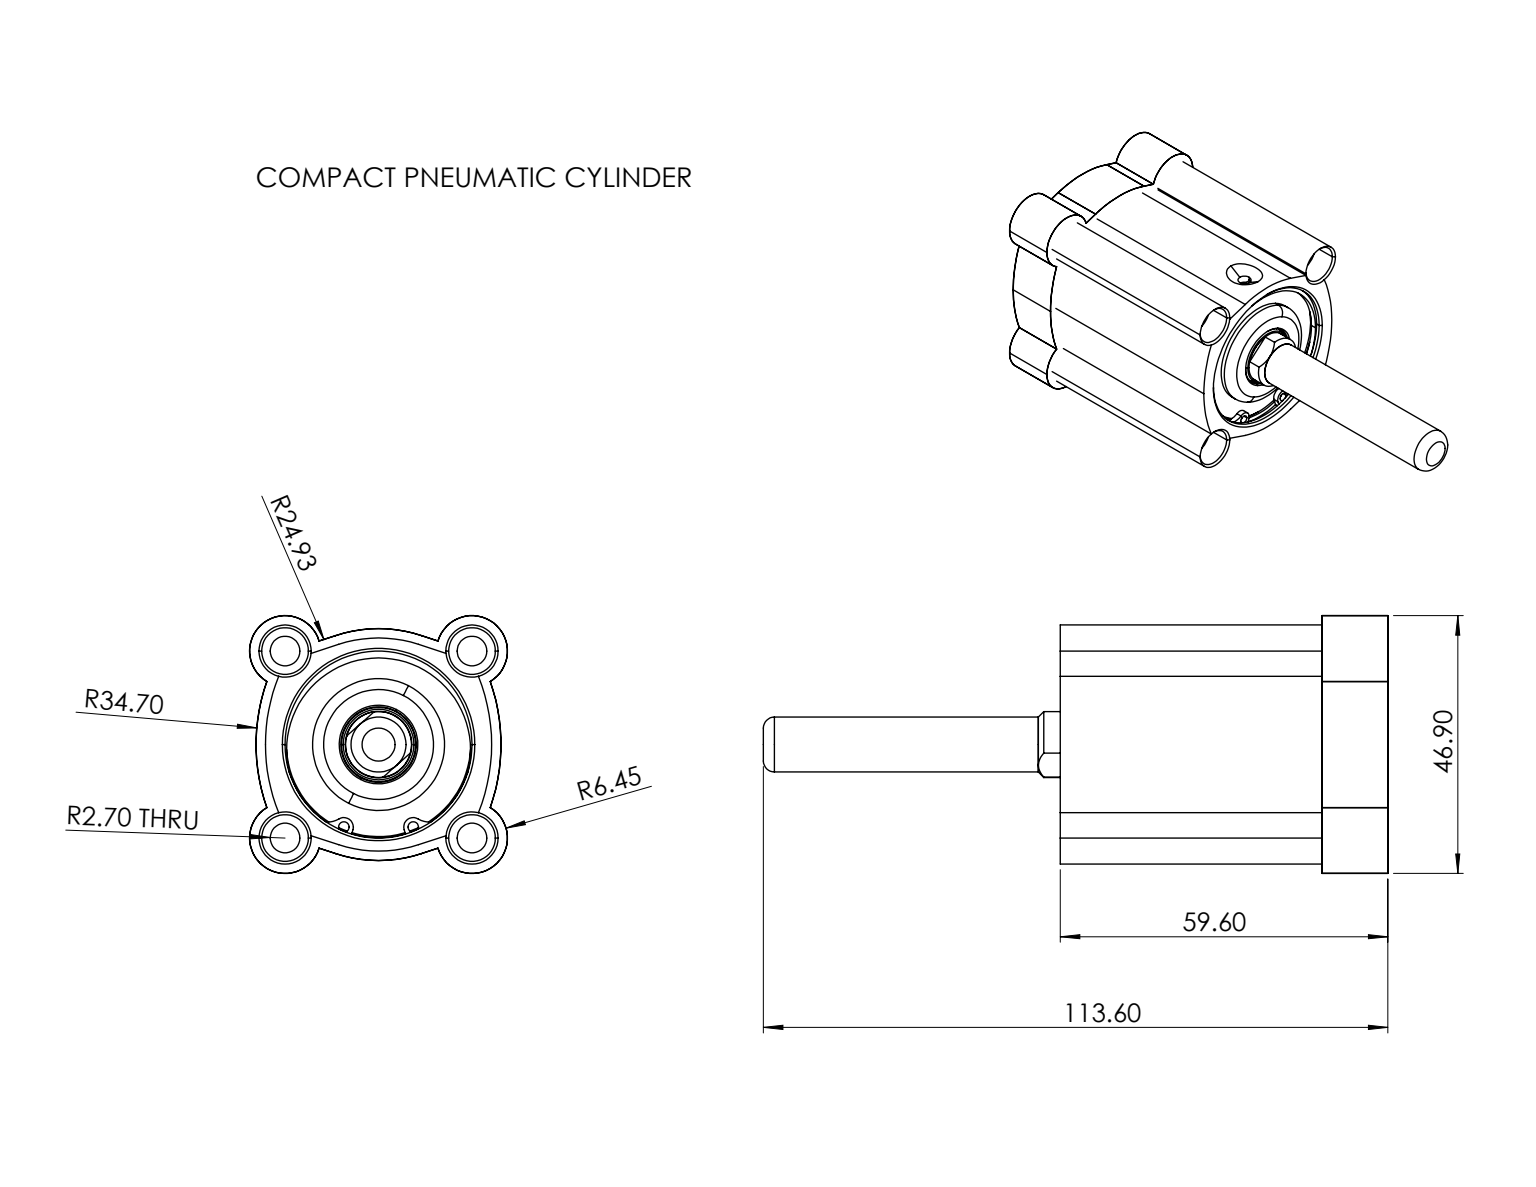
ISO-10303-21;
HEADER;
FILE_DESCRIPTION (('STEP AP214'),
    '1' );
FILE_NAME ('compact pneumatic cylinder.step',
    '2026-10-07T17:53:07',
    ( '' ),
    ( '' ),
    'SwSTEP 2.0',
    'SolidWorks 2025',
    '' );
FILE_SCHEMA (( 'AUTOMOTIVE_DESIGN' ));
ENDSEC;

DATA;
#3=CARTESIAN_POINT ( 'NONE',  ( -18.05918829504999934, 10.97290950744599947, 5.250000000000000000 ) ) ;
#4=FACE_OUTER_BOUND ( 'NONE', #8386, .T. ) ;
#6=VERTEX_POINT ( 'NONE', #3958 ) ;
#8=DIRECTION ( 'NONE',  ( -1.000000000000000000, 0.000000000000000000, 0.000000000000000000 ) ) ;
#10=AXIS2_PLACEMENT_3D ( 'NONE', #13272, #6842, #503 ) ;
#12=CARTESIAN_POINT ( 'NONE',  ( -40.33164489498319938, 10.97290950744599947, 5.250000000000000000 ) ) ;
#16=AXIS2_PLACEMENT_3D ( 'NONE', #5876, #10870, #7634 ) ;
#17=DIRECTION ( 'NONE',  ( -1.000000000000000000, 0.000000000000000000, 0.000000000000000000 ) ) ;
#19=CIRCLE ( 'NONE', #13399, 4.000000000000000888 ) ;
#22=ORIENTED_EDGE ( 'NONE', *, *, #9153, .T. ) ;
#23=EDGE_LOOP ( 'NONE', ( #6039, #6851, #1913, #2067 ) ) ;
#24=CARTESIAN_POINT ( 'NONE',  ( -26.35918829505000005, 10.97290950744599947, 61.86500000000000199 ) ) ;
#26=EDGE_LOOP ( 'NONE', ( #8749, #11948, #13282, #3929 ) ) ;
#27=DIRECTION ( 'NONE',  ( 0.000000000000000000, 0.000000000000000000, -1.000000000000000000 ) ) ;
#28=FACE_OUTER_BOUND ( 'NONE', #13183, .T. ) ;
#30=CARTESIAN_POINT ( 'NONE',  ( -18.05918829504999934, 10.97290950744599947, 57.35000000000000142 ) ) ;
#33=CIRCLE ( 'NONE', #3398, 4.749999999999997335 ) ;
#35=ADVANCED_FACE ( 'NONE', ( #1932 ), #13451, .T. ) ;
#40=CARTESIAN_POINT ( 'NONE',  ( -23.49332020752115113, 0.2738342970428629952, 62.85000000000000142 ) ) ;
#41=DIRECTION ( 'NONE',  ( 1.000000000000000000, 0.000000000000000000, 0.000000000000000000 ) ) ;
#42=CARTESIAN_POINT ( 'NONE',  ( -18.32356812262639068, 30.35913048975403683, 52.99871736656052690 ) ) ;
#44=CARTESIAN_POINT ( 'NONE',  ( -18.05918829505001355, 3.709013078446008027, 62.03182374100007479 ) ) ;
#46=CARTESIAN_POINT ( 'NONE',  ( -1.904759825251885141, 5.678153534393399759, 62.14999999999999858 ) ) ;
#48=( NAMED_UNIT ( * ) SI_UNIT ( $, .STERADIAN. ) SOLID_ANGLE_UNIT ( ) );
#49=CONICAL_SURFACE ( 'NONE', #4748, 17.00000000000000000, 0.7853981633974476129 ) ;
#50=EDGE_CURVE ( 'NONE', #1000, #13804, #2021, .T. ) ;
#53=ORIENTED_EDGE ( 'NONE', *, *, #11858, .F. ) ;
#55=CARTESIAN_POINT ( 'NONE',  ( -10.25088531517542023, -8.860076549334110041, 17.25000000000000000 ) ) ;
#56=CIRCLE ( 'NONE', #12775, 5.000000000000000888 ) ;
#57=CARTESIAN_POINT ( 'NONE',  ( -18.05918829504999934, 10.97290950744599947, 64.85000000000000853 ) ) ;
#58=SURFACE_SIDE_STYLE ('',( #2323 ) ) ;
#59=ORIENTED_EDGE ( 'NONE', *, *, #13776, .F. ) ;
#60=PLANE ( 'NONE',  #2670 ) ;
#62=DIRECTION ( 'NONE',  ( 1.000000000000000000, 0.000000000000000000, 0.000000000000000000 ) ) ;
#63=CARTESIAN_POINT ( 'NONE',  ( -5.631644894983189431, 10.97290950744599947, 17.25000000000000000 ) ) ;
#64=AXIS2_PLACEMENT_3D ( 'NONE', #1240, #10758, #11538 ) ;
#65=ORIENTED_EDGE ( 'NONE', *, *, #6040, .F. ) ;
#69=FACE_OUTER_BOUND ( 'NONE', #8366, .T. ) ;
#70=EDGE_CURVE ( 'NONE', #6919, #7844, #9610, .T. ) ;
#77=CARTESIAN_POINT ( 'NONE',  ( -24.37001676333060018, -4.028726038184999858, 62.14999999999999858 ) ) ;
#78=FACE_OUTER_BOUND ( 'NONE', #2382, .T. ) ;
#82=ORIENTED_EDGE ( 'NONE', *, *, #9714, .T. ) ;
#83=ORIENTED_EDGE ( 'NONE', *, *, #1868, .T. ) ;
#84=EDGE_LOOP ( 'NONE', ( #6155, #12083, #10918, #3272 ) ) ;
#87=VERTEX_POINT ( 'NONE', #8553 ) ;
#90=CARTESIAN_POINT ( 'NONE',  ( -19.42965429280413048, 26.91526772932534683, 56.72114474750378577 ) ) ;
#92=FACE_OUTER_BOUND ( 'NONE', #5027, .T. ) ;
#93=DIRECTION ( 'NONE',  ( 0.000000000000000000, 0.000000000000000000, -1.000000000000000000 ) ) ;
#94=ORIENTED_EDGE ( 'NONE', *, *, #9388, .F. ) ;
#95=VERTEX_POINT ( 'NONE', #8619 ) ;
#96=CARTESIAN_POINT ( 'NONE',  ( -15.05918829504999756, 10.97290950744599947, 118.8499999999999943 ) ) ;
#97=ORIENTED_EDGE ( 'NONE', *, *, #11700, .F. ) ;
#101=AXIS2_PLACEMENT_3D ( 'NONE', #2685, #3784, #6912 ) ;
#103=CARTESIAN_POINT ( 'NONE',  ( -29.51816008892539855, -2.179141222803619993, 63.45000000000000284 ) ) ;
#104=ORIENTED_EDGE ( 'NONE', *, *, #12811, .F. ) ;
#105=CARTESIAN_POINT ( 'NONE',  ( -3.531395436049983960, 3.709013078445997369, 62.03182374100001084 ) ) ;
#107=CARTESIAN_POINT ( 'NONE',  ( -20.77625425128555392, 5.623371902244430842, 57.35000000000000142 ) ) ;
#110=CLOSED_SHELL ( 'NONE', ( #5060, #3881, #6623, #9987, #3732, #7105, #7461, #11688, #1191, #4265, #947, #3436, #2543, #10818, #12397, #3818, #11545, #6558, #4609, #2381, #2843, #3214, #13267, #5308, #5232, #10919, #9049, #5614, #7802, #750 ) ) ;
#113=AXIS2_PLACEMENT_3D ( 'NONE', #7430, #11720, #2167 ) ;
#114=DIRECTION ( 'NONE',  ( 0.000000000000000000, 0.000000000000000000, 1.000000000000000000 ) ) ;
#116=ORIENTED_EDGE ( 'NONE', *, *, #8831, .F. ) ;
#117=ORIENTED_EDGE ( 'NONE', *, *, #6877, .T. ) ;
#118=PLANE ( 'NONE',  #6613 ) ;
#121=CYLINDRICAL_SURFACE ( 'NONE', #12455, 6.000000000000000888 ) ;
#122=LINE ( 'NONE', #4468, #12298 ) ;
#123=AXIS2_PLACEMENT_3D ( 'NONE', #1081, #954, #12877 ) ;
#124=DIRECTION ( 'NONE',  ( 0.000000000000000000, 0.000000000000000000, 1.000000000000000000 ) ) ;
#125=CARTESIAN_POINT ( 'NONE',  ( -18.05918829504999934, 10.97290950744599947, 68.84999999999999432 ) ) ;
#129=VERTEX_POINT ( 'NONE', #4238 ) ;
#130=EDGE_CURVE ( 'NONE', #6071, #11290, #13719, .T. ) ;
#131=CARTESIAN_POINT ( 'NONE',  ( -15.41688231577083101, 30.20956267305470178, 54.20385837980890642 ) ) ;
#134=FACE_OUTER_BOUND ( 'NONE', #5191, .T. ) ;
#136=PLANE ( 'NONE',  #5988 ) ;
#138=DIRECTION ( 'NONE',  ( 0.000000000000000000, 0.000000000000000000, 1.000000000000000000 ) ) ;
#139=ADVANCED_FACE ( 'NONE', ( #10588 ), #13367, .T. ) ;
#142=ORIENTED_EDGE ( 'NONE', *, *, #754, .F. ) ;
#143=EDGE_CURVE ( 'NONE', #7877, #9433, #12710, .T. ) ;
#144=DIRECTION ( 'NONE',  ( 0.000000000000000000, 0.000000000000000000, -1.000000000000000000 ) ) ;
#145=ORIENTED_EDGE ( 'NONE', *, *, #6603, .F. ) ;
#148=CARTESIAN_POINT ( 'NONE',  ( -25.33503448090910126, -7.245613863947209410, 64.85000000000000853 ) ) ;
#149=LINE ( 'NONE', #12938, #855 ) ;
#150=ORIENTED_EDGE ( 'NONE', *, *, #10812, .F. ) ;
#151=CARTESIAN_POINT ( 'NONE',  ( -1.059188295049996231, -6.027090492554000534, 7.250000000000000000 ) ) ;
#153=LINE ( 'NONE', #1273, #6867 ) ;
#154=CARTESIAN_POINT ( 'NONE',  ( -30.48673169511680214, 10.97290950744599947, 5.250000000000000000 ) ) ;
#160=VECTOR ( 'NONE', #1857, 1000.000000000000000 ) ;
#163=EDGE_LOOP ( 'NONE', ( #919, #320, #6279, #11884 ) ) ;
#164=EDGE_LOOP ( 'NONE', ( #8775, #9502, #10616, #5660 ) ) ;
#165=FACE_OUTER_BOUND ( 'NONE', #7206, .T. ) ;
#168=CIRCLE ( 'NONE', #7293, 6.299999999999998046 ) ;
#171=CARTESIAN_POINT ( 'NONE',  ( -20.25693731790400776, 30.25607652235614964, 53.78764270006948323 ) ) ;
#173=CARTESIAN_POINT ( 'NONE',  ( -8.964285665223000521, 0.3335619008453594714, 62.14999999999999858 ) ) ;
#175=CARTESIAN_POINT ( 'NONE',  ( -18.05918829504999934, 10.97290950744599947, 67.84999999999999432 ) ) ;
#176=CARTESIAN_POINT ( 'NONE',  ( -18.05918829504999934, 10.97290950744599947, 56.84999999999999432 ) ) ;
#178=AXIS2_PLACEMENT_3D ( 'NONE', #8254, #12725, #10295 ) ;
#180=AXIS2_PLACEMENT_3D ( 'NONE', #7057, #3723, #3934 ) ;
#185=ORIENTED_EDGE ( 'NONE', *, *, #5640, .F. ) ;
#192=VECTOR ( 'NONE', #12361, 1000.000000000000000 ) ;
#193=FILL_AREA_STYLE_COLOUR ( '', #3402 ) ;
#194=VERTEX_POINT ( 'NONE', #10221 ) ;
#195=VECTOR ( 'NONE', #13133, 1000.000000000000114 ) ;
#196=CARTESIAN_POINT ( 'NONE',  ( -35.05918829505000645, -6.027090492554000534, 7.250000000000000000 ) ) ;
#197=DIRECTION ( 'NONE',  ( 0.000000000000000000, 0.000000000000000000, -1.000000000000000000 ) ) ;
#199=CARTESIAN_POINT ( 'NONE',  ( -1.059188295049996231, 27.97290950744599769, 7.250000000000000000 ) ) ;
#203=CIRCLE ( 'NONE', #9813, 17.00000000000000355 ) ;
#204=CARTESIAN_POINT ( 'NONE',  ( -16.07719306376069568, 30.27579076690150117, 53.62366803667482174 ) ) ;
#206=EDGE_CURVE ( 'NONE', #7753, #7831, #10944, .T. ) ;
#210=PRESENTATION_STYLE_ASSIGNMENT (( #5374 ) ) ;
#213=CARTESIAN_POINT ( 'NONE',  ( -24.10918829505000005, 10.97290950744599947, 64.85000000000000853 ) ) ;
#214=AXIS2_PLACEMENT_3D ( 'NONE', #10840, #5509, #2126 ) ;
#215=AXIS2_PLACEMENT_3D ( 'NONE', #11989, #2447, #13100 ) ;
#216=ORIENTED_EDGE ( 'NONE', *, *, #2968, .F. ) ;
#218=ORIENTED_EDGE ( 'NONE', *, *, #1514, .T. ) ;
#219=DIRECTION ( 'NONE',  ( 0.000000000000000000, 0.000000000000000000, 1.000000000000000000 ) ) ;
#221=EDGE_CURVE ( 'NONE', #8225, #10962, #1891, .T. ) ;
#223=VERTEX_POINT ( 'NONE', #1688 ) ;
#224=VECTOR ( 'NONE', #4940, 1000.000000000000114 ) ;
#226=CIRCLE ( 'NONE', #12506, 15.45000000000000462 ) ;
#227=CONICAL_SURFACE ( 'NONE', #2931, 8.300000000000000711, 0.08573846772804097349 ) ;
#228=AXIS2_PLACEMENT_3D ( 'NONE', #13430, #6224, #8258 ) ;
#229=MANIFOLD_SOLID_BREP ( 'Boss-Extrude1', #6124 ) ;
#232=DIRECTION ( 'NONE',  ( 0.000000000000000000, 0.000000000000000000, 1.000000000000000000 ) ) ;
#233=EDGE_LOOP ( 'NONE', ( #8305, #2316, #6219, #5928, #5645 ) ) ;
#234=EDGE_CURVE ( 'NONE', #8205, #12910, #5618, .T. ) ;
#235=FACE_OUTER_BOUND ( 'NONE', #11663, .T. ) ;
#236=DIRECTION ( 'NONE',  ( -1.000000000000000000, 0.000000000000000000, 0.000000000000000000 ) ) ;
#237=CARTESIAN_POINT ( 'NONE',  ( -18.05918829504999223, 19.28555359244598932, 63.26601075299999621 ) ) ;
#238=CARTESIAN_POINT ( 'NONE',  ( -1.059188295049996231, 27.97290950744599769, 68.85549045786049760 ) ) ;
#239=ADVANCED_FACE ( 'NONE', ( #2830 ), #5929, .T. ) ;
#241=CIRCLE ( 'NONE', #3164, 3.450000000000001510 ) ;
#244=CIRCLE ( 'NONE', #12065, 6.449999999999997513 ) ;
#248=DIRECTION ( 'NONE',  ( 1.000000000000000000, 0.000000000000000000, 0.000000000000000000 ) ) ;
#250=DIRECTION ( 'NONE',  ( 0.000000000000000000, 0.000000000000000000, -1.000000000000000000 ) ) ;
#252=PLANE ( 'NONE',  #16 ) ;
#254=CARTESIAN_POINT ( 'NONE',  ( -19.60333775920156185, 30.30889438432964056, 53.36507960493299407 ) ) ;
#256=CIRCLE ( 'NONE', #8054, 7.618085573000000110 ) ;
#260=VECTOR ( 'NONE', #6397, 1000.000000000000000 ) ;
#261=DIRECTION ( 'NONE',  ( 1.000000000000000000, 0.000000000000000000, 0.000000000000000000 ) ) ;
#265=CIRCLE ( 'NONE', #7605, 16.66282263685194920 ) ;
#270=LINE ( 'NONE', #7860, #10180 ) ;
#271=ORIENTED_EDGE ( 'NONE', *, *, #8365, .T. ) ;
#272=CARTESIAN_POINT ( 'NONE',  ( -32.35918829505000360, -6.027090492554000534, 58.85000000000000142 ) ) ;
#273=CARTESIAN_POINT ( 'NONE',  ( -12.26420230435512160, 9.417873376788568507, 67.84999999999999432 ) ) ;
#277=CARTESIAN_POINT ( 'NONE',  ( -25.33503448090910126, -7.245613863947209410, 7.250000000000000000 ) ) ;
#278=FACE_OUTER_BOUND ( 'NONE', #4596, .T. ) ;
#281=DIRECTION ( 'NONE',  ( -1.000000000000000000, 0.000000000000000000, 0.000000000000000000 ) ) ;
#282=ADVANCED_FACE ( 'NONE', ( #9827 ), #5462, .T. ) ;
#288=CARTESIAN_POINT ( 'NONE',  ( -18.05918829504999934, 30.36027202460864771, 52.99086025162979752 ) ) ;
#290=CARTESIAN_POINT ( 'NONE',  ( -18.05918829249645086, 2.672909507443099741, 63.15000000009349179 ) ) ;
#291=CARTESIAN_POINT ( 'NONE',  ( -20.77625425128555392, 5.623371902244430842, 57.35000000000000142 ) ) ;
#293=CARTESIAN_POINT ( 'NONE',  ( 3.690811704950004657, 27.97290950744599769, 68.85549045786049760 ) ) ;
#297=ADVANCED_FACE ( 'NONE', ( #9087, #3790 ), #4208, .F. ) ;
#300=ORIENTED_EDGE ( 'NONE', *, *, #13287, .F. ) ;
#302=DIRECTION ( 'NONE',  ( 0.000000000000000000, 0.000000000000000000, 1.000000000000000000 ) ) ;
#306=ORIENTED_EDGE ( 'NONE', *, *, #4813, .T. ) ;
#308=DIRECTION ( 'NONE',  ( 0.4528443260392610026, 0.8915896008669278450, 0.000000000000000000 ) ) ;
#311=DIRECTION ( 'NONE',  ( 0.000000000000000000, 0.000000000000000000, 1.000000000000000000 ) ) ;
#312=DIRECTION ( 'NONE',  ( 0.1353548076753729457, 0.000000000000000000, -0.9907971921837297469 ) ) ;
#313=DIRECTION ( 'NONE',  ( -0.6615960714621569316, 0.7498604124941123938, 0.000000000000000000 ) ) ;
#316=ORIENTED_EDGE ( 'NONE', *, *, #12153, .T. ) ;
#318=VERTEX_POINT ( 'NONE', #915 ) ;
#319=CYLINDRICAL_SURFACE ( 'NONE', #4383, 15.45000000000000462 ) ;
#320=ORIENTED_EDGE ( 'NONE', *, *, #2823, .T. ) ;
#321=DIRECTION ( 'NONE',  ( -0.000000000000000000, -0.000000000000000000, 1.000000000000000000 ) ) ;
#322=VERTEX_POINT ( 'NONE', #8389 ) ;
#324=CARTESIAN_POINT ( 'NONE',  ( -21.18139722880372489, 30.14955231547764569, 54.83540917236412326 ) ) ;
#326=CARTESIAN_POINT ( 'NONE',  ( -18.05918829504999934, 2.872909508741170015, 63.35000000000700027 ) ) ;
#328=DIRECTION ( 'NONE',  ( 0.000000000000000000, 0.000000000000000000, 1.000000000000000000 ) ) ;
#330=ORIENTED_EDGE ( 'NONE', *, *, #13140, .T. ) ;
#331=EDGE_CURVE ( 'NONE', #12272, #3141, #6992, .T. ) ;
#334=DIRECTION ( 'NONE',  ( 1.000000000000000000, 0.000000000000000000, 0.000000000000000000 ) ) ;
#335=ORIENTED_EDGE ( 'NONE', *, *, #4099, .T. ) ;
#340=DIRECTION ( 'NONE',  ( -0.9496839325805417342, 0.3132098788326399541, 0.000000000000000000 ) ) ;
#341=LINE ( 'NONE', #9058, #8440 ) ;
#342=CARTESIAN_POINT ( 'NONE',  ( -34.05918829504999934, 10.97290950744599947, 56.84999999999999432 ) ) ;
#345=EDGE_CURVE ( 'NONE', #1822, #1130, #8251, .T. ) ;
#349=VERTEX_POINT ( 'NONE', #11530 ) ;
#350=EDGE_CURVE ( 'NONE', #12769, #6072, #4260, .T. ) ;
#351=ORIENTED_EDGE ( 'NONE', *, *, #13017, .F. ) ;
#358=DIRECTION ( 'NONE',  ( 0.000000000000000000, 0.000000000000000000, -1.000000000000000000 ) ) ;
#360=FACE_OUTER_BOUND ( 'NONE', #13071, .T. ) ;
#364=DIRECTION ( 'NONE',  ( 1.000000000000000000, 0.000000000000000000, 0.000000000000000000 ) ) ;
#368=CARTESIAN_POINT ( 'NONE',  ( -32.58698115404997253, 18.23680593644601089, 62.03182374100001084 ) ) ;
#370=CARTESIAN_POINT ( 'NONE',  ( -11.06274345774342116, 24.74796884084004844, 60.65000000000000568 ) ) ;
#372=CIRCLE ( 'NONE', #1703, 1.725000000000000755 ) ;
#373=CARTESIAN_POINT ( 'NONE',  ( -17.25681213616876164, 26.95277304015176512, 56.08231620102305470 ) ) ;
#382=LINE ( 'NONE', #4652, #10884 ) ;
#383=CARTESIAN_POINT ( 'NONE',  ( -21.60736175305857998, 30.08769857173765416, 55.71792893088887411 ) ) ;
#385=DIRECTION ( 'NONE',  ( -1.000000000000000000, 0.000000000000000000, 0.000000000000000000 ) ) ;
#386=DIRECTION ( 'NONE',  ( -0.9496839325805417342, -0.3132098788326399541, 0.000000000000000000 ) ) ;
#388=AXIS2_PLACEMENT_3D ( 'NONE', #10817, #5485, #2106 ) ;
#393=CIRCLE ( 'NONE', #6637, 4.749999999999997335 ) ;
#394=AXIS2_PLACEMENT_3D ( 'NONE', #13518, #1937, #13587 ) ;
#397=CYLINDRICAL_SURFACE ( 'NONE', #11158, 6.450000000000009948 ) ;
#398=ORIENTED_EDGE ( 'NONE', *, *, #7843, .T. ) ;
#406=ADVANCED_FACE ( 'NONE', ( #4 ), #7444, .T. ) ;
#407=LINE ( 'NONE', #1517, #3985 ) ;
#409=PLANE ( 'NONE',  #6769 ) ;
#410=LINE ( 'NONE', #10063, #2675 ) ;
#411=AXIS2_PLACEMENT_3D ( 'NONE', #10209, #2683, #4898 ) ;
#415=ORIENTED_EDGE ( 'NONE', *, *, #1664, .T. ) ;
#416=LINE ( 'NONE', #7878, #12614 ) ;
#418=VECTOR ( 'NONE', #5319, 1000.000000000000000 ) ;
#419=AXIS2_PLACEMENT_3D ( 'NONE', #7166, #4046, #8361 ) ;
#420=ORIENTED_EDGE ( 'NONE', *, *, #7245, .F. ) ;
#421=ADVANCED_FACE ( 'NONE', ( #4551 ), #12019, .T. ) ;
#422=DIRECTION ( 'NONE',  ( 0.000000000000000000, 0.000000000000000000, -1.000000000000000000 ) ) ;
#423=AXIS2_PLACEMENT_3D ( 'NONE', #11901, #6648, #2493 ) ;
#425=ORIENTED_EDGE ( 'NONE', *, *, #4953, .T. ) ;
#428=EDGE_CURVE ( 'NONE', #7051, #87, #10065, .T. ) ;
#429=CARTESIAN_POINT ( 'NONE',  ( -24.10918829505000005, 10.97290950744599947, 64.85000000000000853 ) ) ;
#430=CIRCLE ( 'NONE', #8236, 6.145833333000000565 ) ;
#432=EDGE_LOOP ( 'NONE', ( #10471, #3421, #1762, #3978 ) ) ;
#439=ORIENTED_EDGE ( 'NONE', *, *, #6372, .F. ) ;
#441=ORIENTED_EDGE ( 'NONE', *, *, #8899, .T. ) ;
#443=CONICAL_SURFACE ( 'NONE', #7785, 16.95000000000000284, 0.7853981633974433940 ) ;
#444=FACE_OUTER_BOUND ( 'NONE', #7372, .T. ) ;
#446=DIRECTION ( 'NONE',  ( -1.000000000000000000, 0.000000000000000000, 0.000000000000000000 ) ) ;
#450=VECTOR ( 'NONE', #8530, 1000.000000000000227 ) ;
#451=VECTOR ( 'NONE', #9676, 1000.000000000000000 ) ;
#456=CARTESIAN_POINT ( 'NONE',  ( -21.14708333414588637, 30.15419697583712733, 54.78115759698135889 ) ) ;
#457=CARTESIAN_POINT ( 'NONE',  ( -18.05918829504999934, 10.97290950744599947, 57.35000000000000142 ) ) ;
#458=CARTESIAN_POINT ( 'NONE',  ( -41.50918829505000218, -6.027090492554000534, 17.25000000000000000 ) ) ;
#460=DIRECTION ( 'NONE',  ( 0.000000000000000000, 0.000000000000000000, -1.000000000000000000 ) ) ;
#461=DIRECTION ( 'NONE',  ( -0.000000000000000000, -0.000000000000000000, 1.000000000000000000 ) ) ;
#462=VECTOR ( 'NONE', #11230, 1000.000000000000227 ) ;
#466=AXIS2_PLACEMENT_3D ( 'NONE', #5182, #8642, #10822 ) ;
#467=VERTEX_POINT ( 'NONE', #290 ) ;
#469=EDGE_CURVE ( 'NONE', #3141, #10024, #8658, .T. ) ;
#471=CARTESIAN_POINT ( 'NONE',  ( -12.54628844161313950, -7.366404416634599883, 63.45000000000000284 ) ) ;
#472=CONICAL_SURFACE ( 'NONE', #3607, 6.049999999999999822, 0.1357715569457985105 ) ;
#474=DIRECTION ( 'NONE',  ( 1.000000000000000000, 0.000000000000000000, 0.000000000000000000 ) ) ;
#475=AXIS2_PLACEMENT_3D ( 'NONE', #3143, #10327, #12625 ) ;
#476=EDGE_LOOP ( 'NONE', ( #7429, #4886, #7264, #4257 ) ) ;
#477=CYLINDRICAL_SURFACE ( 'NONE', #9605, 8.299999999999998934 ) ;
#480=CARTESIAN_POINT ( 'NONE',  ( 0.09777679598749920709, -1.420146627243660031, 68.85549045786049760 ) ) ;
#482=DIRECTION ( 'NONE',  ( -1.000000000000000000, 0.000000000000000000, 0.000000000000000000 ) ) ;
#483=DIRECTION ( 'NONE',  ( -0.000000000000000000, -0.000000000000000000, 1.000000000000000000 ) ) ;
#484=DIRECTION ( 'NONE',  ( -0.3132098788326420635, -0.9496839325805410681, 0.000000000000000000 ) ) ;
#485=DIRECTION ( 'NONE',  ( 0.000000000000000000, 0.000000000000000000, -1.000000000000000000 ) ) ;
#491=ORIENTED_EDGE ( 'NONE', *, *, #6716, .F. ) ;
#493=CARTESIAN_POINT ( 'NONE',  ( -23.85417428574490373, 12.52794563810342154, 67.84999999999999432 ) ) ;
#494=ORIENTED_EDGE ( 'NONE', *, *, #12786, .T. ) ;
#495=EDGE_LOOP ( 'NONE', ( #8465, #5386, #11204, #2294 ) ) ;
#497=EDGE_CURVE ( 'NONE', #7929, #3451, #2337, .T. ) ;
#500=LINE ( 'NONE', #3780, #1311 ) ;
#501=CARTESIAN_POINT ( 'NONE',  ( 1.640811704950005057, 27.97290950744599769, 7.250000000000000000 ) ) ;
#502=CARTESIAN_POINT ( 'NONE',  ( -11.75918829505000041, 10.97290950744599947, 61.86500000000000199 ) ) ;
#503=DIRECTION ( 'NONE',  ( -1.000000000000000000, 0.000000000000000000, 0.000000000000000000 ) ) ;
#504=EDGE_CURVE ( 'NONE', #3446, #7761, #4041, .T. ) ;
#506=VERTEX_POINT ( 'NONE', #8735 ) ;
#508=CARTESIAN_POINT ( 'NONE',  ( -16.54062941099373063, 30.31058478656570188, 61.34775567103718430 ) ) ;
#509=ORIENTED_EDGE ( 'NONE', *, *, #7168, .F. ) ;
#512=EDGE_LOOP ( 'NONE', ( #3363, #9806, #10726, #5357 ) ) ;
#515=CARTESIAN_POINT ( 'NONE',  ( -18.05918829504999934, 10.97290950744599947, 61.65955166399999854 ) ) ;
#516=DIRECTION ( 'NONE',  ( 0.000000000000000000, 0.000000000000000000, 1.000000000000000000 ) ) ;
#518=CYLINDRICAL_SURFACE ( 'NONE', #11011, 6.299999999999999822 ) ;
#520=CARTESIAN_POINT ( 'NONE',  ( -30.80918829504999934, -6.027090492554000534, 64.35000000000000853 ) ) ;
#521=ADVANCED_FACE ( 'NONE', ( #9868 ), #13062, .F. ) ;
#523=EDGE_CURVE ( 'NONE', #7555, #10214, #3846, .T. ) ;
#524=LINE ( 'NONE', #7913, #11304 ) ;
#526=CARTESIAN_POINT ( 'NONE',  ( -25.64433075620760150, -3.961216307075045240, 61.85000000000000142 ) ) ;
#527=CARTESIAN_POINT ( 'NONE',  ( -21.02695553212586432, 30.16999431196798298, 60.09573059200643286 ) ) ;
#529=DIRECTION ( 'NONE',  ( 0.000000000000000000, 0.000000000000000000, -1.000000000000000000 ) ) ;
#531=AXIS2_PLACEMENT_3D ( 'NONE', #7726, #6695, #2740 ) ;
#532=DIRECTION ( 'NONE',  ( 0.000000000000000000, 0.000000000000000000, -1.000000000000000000 ) ) ;
#533=VERTEX_POINT ( 'NONE', #10767 ) ;
#534=CARTESIAN_POINT ( 'NONE',  ( -18.05918829504999934, 10.00028003023991907, 62.14999999999999858 ) ) ;
#537=DIRECTION ( 'NONE',  ( 1.000000000000000000, 0.000000000000000000, 0.000000000000000000 ) ) ;
#538=( LENGTH_UNIT ( ) NAMED_UNIT ( * ) SI_UNIT ( .MILLI., .METRE. ) );
#542=DIRECTION ( 'NONE',  ( 0.000000000000000000, 0.000000000000000000, 1.000000000000000000 ) ) ;
#545=DIRECTION ( 'NONE',  ( 1.000000000000000000, 0.000000000000000000, 0.000000000000000000 ) ) ;
#546=MECHANICAL_DESIGN_GEOMETRIC_PRESENTATION_REPRESENTATION('',(#12596),#10109);
#547=DIRECTION ( 'NONE',  ( 0.000000000000000000, 0.000000000000000000, -1.000000000000000000 ) ) ;
#548=DIRECTION ( 'NONE',  ( 0.000000000000000000, 0.000000000000000000, -1.000000000000000000 ) ) ;
#549=ORIENTED_EDGE ( 'NONE', *, *, #8020, .F. ) ;
#550=ORIENTED_EDGE ( 'NONE', *, *, #345, .F. ) ;
#552=ORIENTED_EDGE ( 'NONE', *, *, #7488, .T. ) ;
#553=ORIENTED_EDGE ( 'NONE', *, *, #616, .F. ) ;
#554=FACE_OUTER_BOUND ( 'NONE', #6549, .T. ) ;
#557=EDGE_LOOP ( 'NONE', ( #13661, #2052 ) ) ;
#558=DIRECTION ( 'NONE',  ( 0.000000000000000000, 0.000000000000000000, -1.000000000000000000 ) ) ;
#560=VECTOR ( 'NONE', #10996, 1000.000000000000227 ) ;
#563=CARTESIAN_POINT ( 'NONE',  ( -18.05918829504999934, 10.97290950744599947, 62.14999999999999858 ) ) ;
#564=DIRECTION ( 'NONE',  ( 0.000000000000000000, 0.000000000000000000, -1.000000000000000000 ) ) ;
#567=ORIENTED_EDGE ( 'NONE', *, *, #3893, .T. ) ;
#568=VECTOR ( 'NONE', #12571, 1000.000000000000000 ) ;
#569=ORIENTED_EDGE ( 'NONE', *, *, #3319, .T. ) ;
#575=CARTESIAN_POINT ( 'NONE',  ( -32.58698115404997253, 3.709013078445997369, 62.03182374100001084 ) ) ;
#576=CARTESIAN_POINT ( 'NONE',  ( -36.21615338608749823, -1.420146627243662030, 64.85000000000000853 ) ) ;
#578=LINE ( 'NONE', #5112, #2725 ) ;
#579=CARTESIAN_POINT ( 'NONE',  ( -24.37001676333060018, -4.028726038184999858, 62.14999999999999858 ) ) ;
#581=DIRECTION ( 'NONE',  ( 0.000000000000000000, 0.000000000000000000, 1.000000000000000000 ) ) ;
#582=AXIS2_PLACEMENT_3D ( 'NONE', #4592, #10119, #13246 ) ;
#584=EDGE_CURVE ( 'NONE', #1164, #10151, #226, .T. ) ;
#585=ORIENTED_EDGE ( 'NONE', *, *, #2198, .T. ) ;
#586=VERTEX_POINT ( 'NONE', #11046 ) ;
#587=AXIS2_PLACEMENT_3D ( 'NONE', #4402, #8584, #10906 ) ;
#588=DIRECTION ( 'NONE',  ( 1.000000000000000000, 0.000000000000000000, 0.000000000000000000 ) ) ;
#589=ORIENTED_EDGE ( 'NONE', *, *, #8356, .F. ) ;
#590=CARTESIAN_POINT ( 'NONE',  ( -18.05918829504999934, 10.97290950744599947, 63.64999999999999858 ) ) ;
#592=CARTESIAN_POINT ( 'NONE',  ( -20.85553867603828593, 30.19135017469169924, 60.31826595084313425 ) ) ;
#593=DIRECTION ( 'NONE',  ( 0.000000000000000000, 0.000000000000000000, -1.000000000000000000 ) ) ;
#594=CARTESIAN_POINT ( 'NONE',  ( -30.80918829504999934, 27.97290950744599769, 64.35000000000000853 ) ) ;
#596=CARTESIAN_POINT ( 'NONE',  ( -25.67727386805000123, 10.97290950744599947, 61.65955166399999854 ) ) ;
#598=CIRCLE ( 'NONE', #5937, 17.00000000000000355 ) ;
#601=DIRECTION ( 'NONE',  ( 0.000000000000000000, 0.000000000000000000, 1.000000000000000000 ) ) ;
#603=CARTESIAN_POINT ( 'NONE',  ( -1.059188295049996231, 27.97290950744599769, 58.85000000000000142 ) ) ;
#605=CARTESIAN_POINT ( 'NONE',  ( -10.38347696868452097, 26.08535324214045303, 57.35000000000000142 ) ) ;
#606=CARTESIAN_POINT ( 'NONE',  ( -18.05918829504999934, 10.97290950744599947, 118.8499999999999943 ) ) ;
#609=DIRECTION ( 'NONE',  ( 0.000000000000000000, 0.000000000000000000, -1.000000000000000000 ) ) ;
#611=CARTESIAN_POINT ( 'NONE',  ( -18.05918829504999934, 10.97290950744599947, 23.90000000000000213 ) ) ;
#613=AXIS2_PLACEMENT_3D ( 'NONE', #13711, #12870, #3257 ) ;
#614=CIRCLE ( 'NONE', #1290, 1.999999999999998890 ) ;
#616=EDGE_CURVE ( 'NONE', #1958, #10012, #1673, .T. ) ;
#617=DIRECTION ( 'NONE',  ( 1.000000000000000000, 0.000000000000000000, 0.000000000000000000 ) ) ;
#625=AXIS2_PLACEMENT_3D ( 'NONE', #11625, #6317, #6376 ) ;
#626=CARTESIAN_POINT ( 'NONE',  ( -34.49120980104999035, 2.756898754446010180, 63.36264408499989287 ) ) ;
#628=CYLINDRICAL_SURFACE ( 'NONE', #4795, 6.449999999999997513 ) ;
#632=ADVANCED_FACE ( 'NONE', ( #10206 ), #9225, .F. ) ;
#633=CIRCLE ( 'NONE', #10686, 12.00000000000000355 ) ;
#635=CARTESIAN_POINT ( 'NONE',  ( -15.98447378135880292, 30.26743272304607402, 61.00728932202151356 ) ) ;
#637=ORIENTED_EDGE ( 'NONE', *, *, #12632, .F. ) ;
#639=CARTESIAN_POINT ( 'NONE',  ( -46.97970805730049904, -0.1071066662815775977, 64.85000000000000853 ) ) ;
#640=CARTESIAN_POINT ( 'NONE',  ( -32.37473156004999453, 18.13068114044599710, 61.70038048200006386 ) ) ;
#641=LINE ( 'NONE', #12326, #4442 ) ;
#642=VERTEX_POINT ( 'NONE', #12160 ) ;
#643=CARTESIAN_POINT ( 'NONE',  ( 0.09777679598749920709, -1.420146627243660031, 64.85000000000000853 ) ) ;
#644=DIRECTION ( 'NONE',  ( 1.000000000000000000, 0.000000000000000000, 0.000000000000000000 ) ) ;
#647=CARTESIAN_POINT ( 'NONE',  ( -16.74984313037099781, 27.92258346524268475, 58.10825715175638351 ) ) ;
#648=CIRCLE ( 'NONE', #4894, 6.595833333000001630 ) ;
#649=DIRECTION ( 'NONE',  ( 0.000000000000000000, 0.000000000000000000, -1.000000000000000000 ) ) ;
#651=VERTEX_POINT ( 'NONE', #8027 ) ;
#652=ORIENTED_EDGE ( 'NONE', *, *, #9198, .T. ) ;
#653=CIRCLE ( 'NONE', #8245, 18.00000000000000000 ) ;
#658=DIRECTION ( 'NONE',  ( -1.000000000000000000, 0.000000000000000000, 0.000000000000000000 ) ) ;
#659=DIRECTION ( 'NONE',  ( 0.000000000000000000, 0.000000000000000000, -1.000000000000000000 ) ) ;
#665=VERTEX_POINT ( 'NONE', #12304 ) ;
#666=ORIENTED_EDGE ( 'NONE', *, *, #3497, .T. ) ;
#668=CARTESIAN_POINT ( 'NONE',  ( -32.35918829505000360, 27.97290950744599769, 58.85000000000000142 ) ) ;
#670=DIRECTION ( 'NONE',  ( 0.000000000000000000, 0.000000000000000000, -1.000000000000000000 ) ) ;
#671=DIRECTION ( 'NONE',  ( -1.000000000000000000, 0.000000000000000000, 0.000000000000000000 ) ) ;
#672=AXIS2_PLACEMENT_3D ( 'NONE', #7930, #1510, #1232 ) ;
#673=AXIS2_PLACEMENT_3D ( 'NONE', #3504, #2473, #9929 ) ;
#676=DIRECTION ( 'NONE',  ( 1.000000000000000000, 0.000000000000000000, 0.000000000000000000 ) ) ;
#677=AXIS2_PLACEMENT_3D ( 'NONE', #13631, #848, #1908 ) ;
#679=DIRECTION ( 'NONE',  ( 0.000000000000000000, -1.000000000000000000, 0.000000000000000000 ) ) ;
#684=VECTOR ( 'NONE', #328, 1000.000000000000000 ) ;
#686=DIRECTION ( 'NONE',  ( 0.000000000000000000, 1.000000000000000000, 0.000000000000000000 ) ) ;
#688=EDGE_CURVE ( 'NONE', #1735, #8958, #13408, .T. ) ;
#690=CYLINDRICAL_SURFACE ( 'NONE', #8513, 6.449999999999997513 ) ;
#692=AXIS2_PLACEMENT_3D ( 'NONE', #1538, #7951, #7885 ) ;
#693=AXIS2_PLACEMENT_3D ( 'NONE', #7006, #13442, #12398 ) ;
#695=AXIS2_PLACEMENT_3D ( 'NONE', #7919, #9259, #8346 ) ;
#697=DIRECTION ( 'NONE',  ( 0.000000000000000000, 0.000000000000000000, 1.000000000000000000 ) ) ;
#698=AXIS2_PLACEMENT_3D ( 'NONE', #6763, #12980, #13188 ) ;
#700=CARTESIAN_POINT ( 'NONE',  ( -15.26994104352865023, 30.19221003217483101, 60.32689770076000713 ) ) ;
#701=ADVANCED_FACE ( 'NONE', ( #12089 ), #8706, .T. ) ;
#702=ORIENTED_EDGE ( 'NONE', *, *, #5578, .T. ) ;
#703=VERTEX_POINT ( 'NONE', #12706 ) ;
#705=LINE ( 'NONE', #2058, #9615 ) ;
#707=VERTEX_POINT ( 'NONE', #6065 ) ;
#708=DIRECTION ( 'NONE',  ( 0.000000000000000000, 0.000000000000000000, 1.000000000000000000 ) ) ;
#709=DIRECTION ( 'NONE',  ( 0.000000000000000000, 0.000000000000000000, -1.000000000000000000 ) ) ;
#711=DIRECTION ( 'NONE',  ( 0.000000000000000000, 0.000000000000000000, 1.000000000000000000 ) ) ;
#714=EDGE_CURVE ( 'NONE', #95, #9971, #5288, .T. ) ;
#717=ORIENTED_EDGE ( 'NONE', *, *, #9515, .F. ) ;
#718=EDGE_CURVE ( 'NONE', #999, #11456, #9839, .T. ) ;
#722=VERTEX_POINT ( 'NONE', #5224 ) ;
#723=ORIENTED_EDGE ( 'NONE', *, *, #3044, .T. ) ;
#725=CARTESIAN_POINT ( 'NONE',  ( -10.89348439749693931, -4.443078545630354981, 62.14999999999999858 ) ) ;
#727=DIRECTION ( 'NONE',  ( 0.000000000000000000, 0.000000000000000000, -1.000000000000000000 ) ) ;
#735=ORIENTED_EDGE ( 'NONE', *, *, #3847, .F. ) ;
#737=CIRCLE ( 'NONE', #12119, 2.700000000000000178 ) ;
#739=EDGE_CURVE ( 'NONE', #9938, #3923, #2277, .T. ) ;
#741=ORIENTED_EDGE ( 'NONE', *, *, #9101, .T. ) ;
#742=CARTESIAN_POINT ( 'NONE',  ( -22.02876472382295248, 15.47207198241065029, 64.85000000000000853 ) ) ;
#743=DIRECTION ( 'NONE',  ( 0.4528443260392608916, 0.8915896008669279560, 0.000000000000000000 ) ) ;
#744=AXIS2_PLACEMENT_3D ( 'NONE', #7799, #6965, #281 ) ;
#747=DIRECTION ( 'NONE',  ( -1.000000000000000000, 0.000000000000000000, 0.000000000000000000 ) ) ;
#750=ADVANCED_FACE ( 'NONE', ( #8166 ), #4053, .F. ) ;
#751=DIRECTION ( 'NONE',  ( 0.4528443260392610026, 0.8915896008669277339, 0.000000000000000000 ) ) ;
#752=CARTESIAN_POINT ( 'NONE',  ( -25.33503448090910126, -7.245613863947209410, 68.85549045786049760 ) ) ;
#753=EDGE_CURVE ( 'NONE', #8302, #651, #10078, .T. ) ;
#754=EDGE_CURVE ( 'NONE', #707, #12928, #8309, .T. ) ;
#756=ORIENTED_EDGE ( 'NONE', *, *, #234, .F. ) ;
#758=ORIENTED_EDGE ( 'NONE', *, *, #5194, .F. ) ;
#759=VERTEX_POINT ( 'NONE', #5020 ) ;
#760=ORIENTED_EDGE ( 'NONE', *, *, #5002, .F. ) ;
#762=CARTESIAN_POINT ( 'NONE',  ( -18.05918829504999934, 10.97290950744599947, 57.54999999999999716 ) ) ;
#763=CARTESIAN_POINT ( 'NONE',  ( -18.05918829504999934, 10.97290950744599947, 64.85000000000000853 ) ) ;
#766=CARTESIAN_POINT ( 'NONE',  ( -28.87730642030694739, 29.81324547859995278, 17.25000000000000000 ) ) ;
#767=EDGE_CURVE ( 'NONE', #7051, #13581, #9290, .T. ) ;
#768=CARTESIAN_POINT ( 'NONE',  ( -10.47404583389237942, 25.90703532196704728, 61.85000000000000142 ) ) ;
#769=FACE_OUTER_BOUND ( 'NONE', #2166, .T. ) ;
#771=ORIENTED_EDGE ( 'NONE', *, *, #9810, .F. ) ;
#773=CARTESIAN_POINT ( 'NONE',  ( -14.47298380915872329, 30.08178984978628279, 55.82826930748674243 ) ) ;
#774=EDGE_LOOP ( 'NONE', ( #9428, #4976, #4421, #4256 ) ) ;
#777=CARTESIAN_POINT ( 'NONE',  ( -27.15409092487699994, 0.3335619008453594714, 62.14999999999999858 ) ) ;
#781=DIRECTION ( 'NONE',  ( -0.3132098788326352912, -0.9496839325805432885, 0.000000000000000000 ) ) ;
#782=DIRECTION ( 'NONE',  ( 1.000000000000000000, 0.000000000000000000, 0.000000000000000000 ) ) ;
#783=DIRECTION ( 'NONE',  ( -1.000000000000000000, 0.000000000000000000, 0.000000000000000000 ) ) ;
#784=DIRECTION ( 'NONE',  ( -1.000000000000000000, 0.000000000000000000, 0.000000000000000000 ) ) ;
#787=EDGE_LOOP ( 'NONE', ( #3326, #3499 ) ) ;
#788=ORIENTED_EDGE ( 'NONE', *, *, #13319, .F. ) ;
#790=ORIENTED_EDGE ( 'NONE', *, *, #753, .T. ) ;
#793=CARTESIAN_POINT ( 'NONE',  ( -37.75918829505000218, -6.027090492554000534, 7.250000000000000000 ) ) ;
#794=CARTESIAN_POINT ( 'NONE',  ( -18.05918829504999934, 10.97290950744599947, 61.86500000000000199 ) ) ;
#795=CYLINDRICAL_SURFACE ( 'NONE', #10653, 4.250000000000000000 ) ;
#800=AXIS2_PLACEMENT_3D ( 'NONE', #3403, #6591, #6800 ) ;
#803=VERTEX_POINT ( 'NONE', #7376 ) ;
#804=EDGE_LOOP ( 'NONE', ( #9625, #4091 ) ) ;
#805=LINE ( 'NONE', #3755, #462 ) ;
#806=FACE_OUTER_BOUND ( 'NONE', #11782, .T. ) ;
#807=DIRECTION ( 'NONE',  ( 0.000000000000000000, -1.000000000000000000, 0.000000000000000000 ) ) ;
#808=DIRECTION ( 'NONE',  ( 0.000000000000000000, 0.000000000000000000, 1.000000000000000000 ) ) ;
#811=FACE_OUTER_BOUND ( 'NONE', #12970, .T. ) ;
#813=DIRECTION ( 'NONE',  ( 0.6615960714621564875, -0.7498604124941129490, 0.000000000000000000 ) ) ;
#814=FILL_AREA_STYLE_COLOUR ( '', #12680 ) ;
#815=ORIENTED_EDGE ( 'NONE', *, *, #331, .F. ) ;
#817=VECTOR ( 'NONE', #10677, 1000.000000000000000 ) ;
#819=ORIENTED_EDGE ( 'NONE', *, *, #1738, .F. ) ;
#822=ORIENTED_EDGE ( 'NONE', *, *, #13532, .F. ) ;
#824=DIRECTION ( 'NONE',  ( 0.000000000000000000, 0.000000000000000000, -1.000000000000000000 ) ) ;
#828=EDGE_CURVE ( 'NONE', #4114, #7318, #4718, .T. ) ;
#832=ORIENTED_EDGE ( 'NONE', *, *, #10912, .T. ) ;
#833=ADVANCED_FACE ( 'NONE', ( #2460 ), #12829, .F. ) ;
#834=CARTESIAN_POINT ( 'NONE',  ( -14.45668717981020457, 30.07924626547106683, 55.87780969119025087 ) ) ;
#835=CIRCLE ( 'NONE', #2430, 8.250000000000001776 ) ;
#838=ORIENTED_EDGE ( 'NONE', *, *, #4604, .F. ) ;
#842=DIRECTION ( 'NONE',  ( -1.000000000000000000, 0.000000000000000000, 0.000000000000000000 ) ) ;
#843=CARTESIAN_POINT ( 'NONE',  ( -18.05918829505001000, 2.755752219877027009, 63.35000000030875356 ) ) ;
#845=DIRECTION ( 'NONE',  ( -1.000000000000000000, 0.000000000000000000, 0.000000000000000000 ) ) ;
#846=CARTESIAN_POINT ( 'NONE',  ( -35.05918829505000645, -6.027090492554000534, 17.25000000000000000 ) ) ;
#847=EDGE_CURVE ( 'NONE', #13286, #11868, #12517, .T. ) ;
#848=DIRECTION ( 'NONE',  ( 0.000000000000000000, 0.000000000000000000, -1.000000000000000000 ) ) ;
#849=CARTESIAN_POINT ( 'NONE',  ( 2.262399129208274573, -0.4981161769137525952, 5.250000000000000000 ) ) ;
#850=CARTESIAN_POINT ( 'NONE',  ( -6.600216501174579697, -2.179141222803619993, 62.14999999999999858 ) ) ;
#852=AXIS2_PLACEMENT_3D ( 'NONE', #4821, #3857, #4429 ) ;
#853=VECTOR ( 'NONE', #4362, 1000.000000000000000 ) ;
#855=VECTOR ( 'NONE', #2074, 999.9999999999998863 ) ;
#857=ORIENTED_EDGE ( 'NONE', *, *, #1780, .T. ) ;
#860=CIRCLE ( 'NONE', #13355, 1.725000000000000755 ) ;
#863=DIRECTION ( 'NONE',  ( 0.000000000000000000, 0.000000000000000000, 1.000000000000000000 ) ) ;
#865=EDGE_CURVE ( 'NONE', #4986, #349, #9169, .T. ) ;
#866=CARTESIAN_POINT ( 'NONE',  ( -19.16403910648224596, 30.33404188115190436, 61.52219105696395474 ) ) ;
#868=CARTESIAN_POINT ( 'NONE',  ( -13.40033457972183939, -4.525318844826149878, 62.14999999999999858 ) ) ;
#873=ORIENTED_EDGE ( 'NONE', *, *, #5532, .F. ) ;
#874=EDGE_LOOP ( 'NONE', ( #7978, #8631 ) ) ;
#876=VECTOR ( 'NONE', #5241, 1000.000000000000000 ) ;
#877=DIRECTION ( 'NONE',  ( 0.000000000000000000, 0.000000000000000000, -1.000000000000000000 ) ) ;
#879=ORIENTED_EDGE ( 'NONE', *, *, #9126, .F. ) ;
#884=DIRECTION ( 'NONE',  ( 1.000000000000000000, 0.000000000000000000, 0.000000000000000000 ) ) ;
#888=AXIS2_PLACEMENT_3D ( 'NONE', #11953, #2684, #6911 ) ;
#889=CARTESIAN_POINT ( 'NONE',  ( 0.000000000000000000, 0.000000000000000000, 7.250000000000000000 ) ) ;
#890=AXIS2_PLACEMENT_3D ( 'NONE', #8915, #4733, #3547 ) ;
#893=ORIENTED_EDGE ( 'NONE', *, *, #7390, .F. ) ;
#894=ORIENTED_EDGE ( 'NONE', *, *, #7603, .F. ) ;
#897=CARTESIAN_POINT ( 'NONE',  ( -40.33164489498319938, 10.97290950744599947, 17.25000000000000000 ) ) ;
#898=VERTEX_POINT ( 'NONE', #7433 ) ;
#899=ORIENTED_EDGE ( 'NONE', *, *, #1394, .F. ) ;
#900=DIRECTION ( 'NONE',  ( -1.000000000000000000, 0.000000000000000000, 0.000000000000000000 ) ) ;
#902=CARTESIAN_POINT ( 'NONE',  ( -41.50918829505000218, -6.027090492554000534, 5.250000000000000000 ) ) ;
#903=CARTESIAN_POINT ( 'NONE',  ( -18.05918829504999934, 10.97290950744599947, 63.02000000000000313 ) ) ;
#907=CIRCLE ( 'NONE', #2271, 6.849999999999999645 ) ;
#909=ORIENTED_EDGE ( 'NONE', *, *, #1487, .F. ) ;
#910=CARTESIAN_POINT ( 'NONE',  ( -14.60499646201505186, 30.10205818033629299, 59.22435544807014907 ) ) ;
#912=VERTEX_POINT ( 'NONE', #6408 ) ;
#913=DIRECTION ( 'NONE',  ( 0.000000000000000000, 0.000000000000000000, 1.000000000000000000 ) ) ;
#914=CIRCLE ( 'NONE', #8279, 16.00000000000000000 ) ;
#915=CARTESIAN_POINT ( 'NONE',  ( -11.71335496205000126, 10.97290950744599947, 60.40999999999999659 ) ) ;
#916=VECTOR ( 'NONE', #2209, 1000.000000000000000 ) ;
#918=VERTEX_POINT ( 'NONE', #6688 ) ;
#919=ORIENTED_EDGE ( 'NONE', *, *, #9714, .F. ) ;
#921=FACE_OUTER_BOUND ( 'NONE', #12157, .T. ) ;
#924=DIRECTION ( 'NONE',  ( 0.000000000000000000, 0.000000000000000000, -1.000000000000000000 ) ) ;
#925=DIRECTION ( 'NONE',  ( 1.000000000000000000, 0.000000000000000000, 0.000000000000000000 ) ) ;
#927=DIRECTION ( 'NONE',  ( 1.000000000000000000, -1.792228749776983267E-15, 0.000000000000000000 ) ) ;
#929=AXIS2_PLACEMENT_3D ( 'NONE', #13132, #12161, #1467 ) ;
#930=AXIS2_PLACEMENT_3D ( 'NONE', #2140, #27, #6855 ) ;
#936=VERTEX_POINT ( 'NONE', #9767 ) ;
#942=CARTESIAN_POINT ( 'NONE',  ( -20.31624426159365626, 30.25036691372644881, 60.86381688408464896 ) ) ;
#943=CIRCLE ( 'NONE', #11875, 2.700000000000000178 ) ;
#946=FACE_OUTER_BOUND ( 'NONE', #13280, .T. ) ;
#947=ADVANCED_FACE ( 'NONE', ( #11786 ), #472, .F. ) ;
#951=AXIS2_PLACEMENT_3D ( 'NONE', #11850, #9687, #9544 ) ;
#952=VERTEX_POINT ( 'NONE', #9701 ) ;
#953=ORIENTED_EDGE ( 'NONE', *, *, #5603, .T. ) ;
#954=DIRECTION ( 'NONE',  ( 0.000000000000000000, 0.000000000000000000, -1.000000000000000000 ) ) ;
#955=DIRECTION ( 'NONE',  ( 0.000000000000000000, 0.000000000000000000, -1.000000000000000000 ) ) ;
#956=VERTEX_POINT ( 'NONE', #4333 ) ;
#957=LINE ( 'NONE', #5336, #4928 ) ;
#962=LINE ( 'NONE', #4945, #9540 ) ;
#963=CARTESIAN_POINT ( 'NONE',  ( -18.05918829504999934, 10.97290950744599947, 17.25000000000000000 ) ) ;
#964=DIRECTION ( 'NONE',  ( -1.000000000000000000, 0.000000000000000000, 0.000000000000000000 ) ) ;
#965=AXIS2_PLACEMENT_3D ( 'NONE', #794, #4025, #1642 ) ;
#966=LINE ( 'NONE', #11855, #9582 ) ;
#967=FACE_BOUND ( 'NONE', #1057, .T. ) ;
#968=ORIENTED_EDGE ( 'NONE', *, *, #7622, .F. ) ;
#969=CIRCLE ( 'NONE', #4104, 5.000000000000000888 ) ;
#974=ORIENTED_EDGE ( 'NONE', *, *, #3018, .T. ) ;
#975=CARTESIAN_POINT ( 'NONE',  ( -20.72384131171161670, 15.28981433190530481, 68.77695026631712949 ) ) ;
#977=DIRECTION ( 'NONE',  ( -1.000000000000000000, 0.000000000000000000, 0.000000000000000000 ) ) ;
#979=DIRECTION ( 'NONE',  ( 1.000000000000000000, 0.000000000000000000, 0.000000000000000000 ) ) ;
#981=AXIS2_PLACEMENT_3D ( 'NONE', #1980, #1903, #12787 ) ;
#983=EDGE_LOOP ( 'NONE', ( #822, #4361, #9939, #6406 ) ) ;
#984=CARTESIAN_POINT ( 'NONE',  ( -14.25042417982650278, 30.04605120274296581, 56.81979108752121732 ) ) ;
#986=EDGE_CURVE ( 'NONE', #8958, #194, #11849, .T. ) ;
#988=EDGE_LOOP ( 'NONE', ( #8522, #8841 ) ) ;
#993=CARTESIAN_POINT ( 'NONE',  ( -25.86749127492454647, -8.860076549334129581, 5.250000000000000000 ) ) ;
#994=DIRECTION ( 'NONE',  ( 1.000000000000000000, 0.000000000000000000, 0.000000000000000000 ) ) ;
#995=DIRECTION ( 'NONE',  ( -0.6615960714621568206, 0.7498604124941127269, 0.000000000000000000 ) ) ;
#998=EDGE_CURVE ( 'NONE', #1834, #3793, #2322, .T. ) ;
#999=VERTEX_POINT ( 'NONE', #9979 ) ;
#1000=VERTEX_POINT ( 'NONE', #12281 ) ;
#1001=CARTESIAN_POINT ( 'NONE',  ( -1.059188295049996231, 10.97290950744599947, 64.35000000000000853 ) ) ;
#1004=DIRECTION ( 'NONE',  ( 0.000000000000000000, 0.000000000000000000, -1.000000000000000000 ) ) ;
#1005=CARTESIAN_POINT ( 'NONE',  ( -17.78571402079797892, 26.97096642121225685, 55.86712588480680353 ) ) ;
#1007=DIRECTION ( 'NONE',  ( -1.000000000000000000, 0.000000000000000000, 0.000000000000000000 ) ) ;
#1009=AXIS2_PLACEMENT_3D ( 'NONE', #10779, #9586, #6641 ) ;
#1010=DIRECTION ( 'NONE',  ( 0.7071067811865500152, 0.000000000000000000, 0.7071067811865450192 ) ) ;
#1013=ADVANCED_FACE ( 'NONE', ( #7022 ), #3760, .F. ) ;
#1018=DIRECTION ( 'NONE',  ( 0.000000000000000000, 0.000000000000000000, -1.000000000000000000 ) ) ;
#1020=DIRECTION ( 'NONE',  ( 0.000000000000000000, 1.000000000000000000, 0.000000000000000000 ) ) ;
#1021=DIRECTION ( 'NONE',  ( 0.000000000000000000, 0.000000000000000000, -1.000000000000000000 ) ) ;
#1022=CARTESIAN_POINT ( 'NONE',  ( -23.85417428574490373, 12.52794563810342154, 64.85000000000000853 ) ) ;
#1023=ADVANCED_FACE ( 'NONE', ( #5698 ), #6891, .T. ) ;
#1027=( BOUNDED_SURFACE ( )  B_SPLINE_SURFACE ( 3, 3, ( 
 ( #12793, #11740, #6432, #2340 ),
 ( #9511, #10771, #1190, #8741 ),
 ( #3106, #13757, #7328, #8457 ),
 ( #2550, #11050, #12094, #7668 ) ),
 .UNSPECIFIED., .F., .F., .F. ) 
 B_SPLINE_SURFACE_WITH_KNOTS ( ( 4, 4 ),
 ( 4, 4 ),
 ( 0.000000000000000000, 1.000000000000000000 ),
 ( 0.000000000000000000, 1.000000000000000000 ),
 .UNSPECIFIED. ) 
 GEOMETRIC_REPRESENTATION_ITEM ( )  RATIONAL_B_SPLINE_SURFACE ( (
 ( 1.000000000000000000, 0.3333333333333329818, 0.3333333333333329818, 1.000000000000000000),
 ( 0.7553208711179729695, 0.2517736237059909898, 0.2517736237059909898, 0.7553208711179729695),
 ( 0.7553208711179729695, 0.2517736237059909898, 0.2517736237059909898, 0.7553208711179729695),
 ( 1.000000000000000000, 0.3333333333333329818, 0.3333333333333329818, 1.000000000000000000) ) ) 
 REPRESENTATION_ITEM ( '' )  SURFACE ( )  );
#1029=ORIENTED_EDGE ( 'NONE', *, *, #10898, .T. ) ;
#1030=ORIENTED_EDGE ( 'NONE', *, *, #428, .F. ) ;
#1031=DIRECTION ( 'NONE',  ( 1.000000000000000000, 0.000000000000000000, 0.000000000000000000 ) ) ;
#1032=AXIS2_PLACEMENT_3D ( 'NONE', #7320, #3174, #6360 ) ;
#1037=CARTESIAN_POINT ( 'NONE',  ( -18.05918829504999934, 10.97290950744599947, 60.85000000000000142 ) ) ;
#1041=DIRECTION ( 'NONE',  ( 1.000000000000000000, 0.000000000000000000, 0.000000000000000000 ) ) ;
#1042=VERTEX_POINT ( 'NONE', #1724 ) ;
#1047=CYLINDRICAL_SURFACE ( 'NONE', #5313, 18.00000000000000000 ) ;
#1050=DIRECTION ( 'NONE',  ( 1.000000000000000000, 0.000000000000000000, 0.000000000000000000 ) ) ;
#1051=EDGE_CURVE ( 'NONE', #13262, #13219, #7867, .T. ) ;
#1055=EDGE_LOOP ( 'NONE', ( #11743, #1398, #10361, #10586 ) ) ;
#1056=DIRECTION ( 'NONE',  ( 1.000000000000000000, 0.000000000000000000, 0.000000000000000000 ) ) ;
#1057=EDGE_LOOP ( 'NONE', ( #4199, #7252 ) ) ;
#1058=ORIENTED_EDGE ( 'NONE', *, *, #8481, .T. ) ;
#1061=DIRECTION ( 'NONE',  ( 0.000000000000000000, 0.000000000000000000, -1.000000000000000000 ) ) ;
#1064=DIRECTION ( 'NONE',  ( 0.000000000000000000, 2.732534507816520408E-15, 1.000000000000000000 ) ) ;
#1065=CIRCLE ( 'NONE', #852, 3.000000000000001332 ) ;
#1066=DIRECTION ( 'NONE',  ( -2.267612386897784912E-16, 1.000000000000000000, 0.000000000000000000 ) ) ;
#1069=VECTOR ( 'NONE', #11237, 1000.000000000000000 ) ;
#1070=CYLINDRICAL_SURFACE ( 'NONE', #3179, 4.750000000000000888 ) ;
#1071=CIRCLE ( 'NONE', #6425, 16.75000000000000355 ) ;
#1072=DIRECTION ( 'NONE',  ( -1.000000000000000000, 0.000000000000000000, 0.000000000000000000 ) ) ;
#1078=EDGE_LOOP ( 'NONE', ( #8229, #12932, #2407, #9421, #12105, #10029, #4887, #9297 ) ) ;
#1080=VECTOR ( 'NONE', #13189, 1000.000000000000000 ) ;
#1081=CARTESIAN_POINT ( 'NONE',  ( -18.05918829504999934, 10.97290950744599947, 64.85000000000000853 ) ) ;
#1082=ORIENTED_EDGE ( 'NONE', *, *, #3973, .T. ) ;
#1085=DIRECTION ( 'NONE',  ( 0.000000000000000000, 0.000000000000000000, 1.000000000000000000 ) ) ;
#1086=FACE_OUTER_BOUND ( 'NONE', #3397, .T. ) ;
#1088=CARTESIAN_POINT ( 'NONE',  ( -18.05918829505001355, 3.364325185446006117, 61.98378871700002435 ) ) ;
#1091=EDGE_CURVE ( 'NONE', #8284, #12316, #5585, .T. ) ;
#1093=ADVANCED_FACE ( 'NONE', ( #8928 ), #13314, .T. ) ;
#1094=ORIENTED_EDGE ( 'NONE', *, *, #12335, .T. ) ;
#1095=CARTESIAN_POINT ( 'NONE',  ( -25.33503448090910126, 29.19143287883919768, 64.85000000000000853 ) ) ;
#1099=CIRCLE ( 'NONE', #2017, 6.449999999999997513 ) ;
#1101=CARTESIAN_POINT ( 'NONE',  ( -15.65757483969475139, 6.423926902242667047, 68.70888082541688391 ) ) ;
#1102=DIRECTION ( 'NONE',  ( 0.000000000000000000, 0.000000000000000000, -1.000000000000000000 ) ) ;
#1105=ORIENTED_EDGE ( 'NONE', *, *, #143, .F. ) ;
#1106=ADVANCED_FACE ( 'NONE', ( #9134 ), #6762, .F. ) ;
#1107=CARTESIAN_POINT ( 'NONE',  ( -16.30182512297070829, 30.29372715573303054, 53.48163241110348309 ) ) ;
#1108=VERTEX_POINT ( 'NONE', #3836 ) ;
#1110=FACE_OUTER_BOUND ( 'NONE', #6091, .T. ) ;
#1111=DIRECTION ( 'NONE',  ( -1.000000000000000000, 0.000000000000000000, -0.000000000000000000 ) ) ;
#1112=DIRECTION ( 'NONE',  ( 0.000000000000000000, 0.000000000000000000, -1.000000000000000000 ) ) ;
#1115=CIRCLE ( 'NONE', #672, 2.000000000000000000 ) ;
#1118=CYLINDRICAL_SURFACE ( 'NONE', #3129, 16.72262947720610171 ) ;
#1119=CARTESIAN_POINT ( 'NONE',  ( -37.05918829505000645, 29.97290950744599769, 64.85000000000000853 ) ) ;
#1123=ORIENTED_EDGE ( 'NONE', *, *, #7029, .T. ) ;
#1124=VECTOR ( 'NONE', #7353, 999.9999999999998863 ) ;
#1128=VERTEX_POINT ( 'NONE', #8999 ) ;
#1130=VERTEX_POINT ( 'NONE', #1513 ) ;
#1133=EDGE_CURVE ( 'NONE', #7637, #11014, #11860, .T. ) ;
#1134=CARTESIAN_POINT ( 'NONE',  ( -18.05918829504999934, 7.130333642789880244, 5.250000000000000000 ) ) ;
#1136=LINE ( 'NONE', #10578, #6722 ) ;
#1137=CYLINDRICAL_SURFACE ( 'NONE', #11440, 4.749999999999997335 ) ;
#1139=DIRECTION ( 'NONE',  ( -1.000000000000000000, 0.000000000000000000, 0.000000000000000000 ) ) ;
#1140=CARTESIAN_POINT ( 'NONE',  ( -13.05918829504999756, 10.97290950744599947, 116.8499999999999943 ) ) ;
#1141=AXIS2_PLACEMENT_3D ( 'NONE', #9226, #4896, #12642 ) ;
#1142=AXIS2_PLACEMENT_3D ( 'NONE', #2025, #13458, #8422 ) ;
#1143=PRODUCT_CONTEXT ( 'NONE', #8055, 'mechanical' ) ;
#1144=ORIENTED_EDGE ( 'NONE', *, *, #5002, .T. ) ;
#1146=VERTEX_POINT ( 'NONE', #2090 ) ;
#1152=DIRECTION ( 'NONE',  ( 0.4528443260392607250, 0.8915896008669278450, 0.000000000000000000 ) ) ;
#1153=CARTESIAN_POINT ( 'NONE',  ( -18.84164940403275423, 30.34709526170029648, 53.08392589000639816 ) ) ;
#1156=DIRECTION ( 'NONE',  ( 1.000000000000000000, 0.000000000000000000, 0.000000000000000000 ) ) ;
#1157=CARTESIAN_POINT ( 'NONE',  ( -24.37001676333060018, -4.028726038184999858, 62.14999999999999858 ) ) ;
#1158=DIRECTION ( 'NONE',  ( 1.000000000000000000, 0.000000000000000000, -0.000000000000000000 ) ) ;
#1160=VECTOR ( 'NONE', #6393, 1000.000000000000000 ) ;
#1161=EDGE_CURVE ( 'NONE', #586, #956, #1938, .T. ) ;
#1163=DIRECTION ( 'NONE',  ( 1.000000000000000000, 0.000000000000000000, 0.000000000000000000 ) ) ;
#1164=VERTEX_POINT ( 'NONE', #3139 ) ;
#1166=ORIENTED_EDGE ( 'NONE', *, *, #5935, .F. ) ;
#1168=CARTESIAN_POINT ( 'NONE',  ( -18.05918829504999934, 10.97290950744599947, 62.14999999999999858 ) ) ;
#1171=DIRECTION ( 'NONE',  ( 1.000000000000000000, 0.000000000000000000, 0.000000000000000000 ) ) ;
#1172=CARTESIAN_POINT ( 'NONE',  ( -18.05918829504999934, 10.97290950744599947, 68.84999999999999432 ) ) ;
#1175=DIRECTION ( 'NONE',  ( -1.000000000000000000, 0.000000000000000000, 0.000000000000000000 ) ) ;
#1178=CIRCLE ( 'NONE', #4978, 3.449999999999999734 ) ;
#1180=CARTESIAN_POINT ( 'NONE',  ( -16.38228052275427160, 30.29966228814565454, 53.43569657597039679 ) ) ;
#1181=ORIENTED_EDGE ( 'NONE', *, *, #8350, .F. ) ;
#1182=ADVANCED_FACE ( 'NONE', ( #9419, #12620 ), #5004, .T. ) ;
#1183=DIRECTION ( 'NONE',  ( 0.000000000000000000, 0.000000000000000000, -1.000000000000000000 ) ) ;
#1186=EDGE_LOOP ( 'NONE', ( #4778, #9164, #12277, #13400 ) ) ;
#1189=CIRCLE ( 'NONE', #3879, 8.395833332999997012 ) ;
#1190=CARTESIAN_POINT ( 'NONE',  ( -1.627166789049998563, 19.18892026044596832, 63.36264408499989287 ) ) ;
#1191=ADVANCED_FACE ( 'NONE', ( #8146 ), #3177, .T. ) ;
#1193=ORIENTED_EDGE ( 'NONE', *, *, #10839, .T. ) ;
#1195=DIRECTION ( 'NONE',  ( 0.000000000000000000, 0.000000000000000000, 1.000000000000000000 ) ) ;
#1197=ORIENTED_EDGE ( 'NONE', *, *, #12093, .T. ) ;
#1198=ORIENTED_EDGE ( 'NONE', *, *, #6040, .T. ) ;
#1199=CYLINDRICAL_SURFACE ( 'NONE', #2450, 3.000000000000001332 ) ;
#1201=EDGE_LOOP ( 'NONE', ( #7692, #6041, #5461, #4296 ) ) ;
#1202=DIRECTION ( 'NONE',  ( 0.000000000000000000, 0.000000000000000000, 1.000000000000000000 ) ) ;
#1203=CARTESIAN_POINT ( 'NONE',  ( -17.20901794878084701, 26.95030579715291807, 56.11417500233394406 ) ) ;
#1204=CARTESIAN_POINT ( 'NONE',  ( -35.05918829505000645, 27.97290950744599769, 64.35000000000000853 ) ) ;
#1205=CARTESIAN_POINT ( 'NONE',  ( -18.05918829504999934, 10.97290950744599947, 30.59999999999999787 ) ) ;
#1206=DIRECTION ( 'NONE',  ( 0.000000000000000000, 0.000000000000000000, 1.000000000000000000 ) ) ;
#1209=ORIENTED_EDGE ( 'NONE', *, *, #11415, .F. ) ;
#1211=CYLINDRICAL_SURFACE ( 'NONE', #7038, 12.00000000000000355 ) ;
#1213=DIRECTION ( 'NONE',  ( 0.000000000000000000, 0.000000000000000000, -1.000000000000000000 ) ) ;
#1216=AXIS2_PLACEMENT_3D ( 'NONE', #1473, #7960, #11057 ) ;
#1217=CARTESIAN_POINT ( 'NONE',  ( -18.74037715811554961, 30.35031926759491938, 53.06094751610090299 ) ) ;
#1218=CARTESIAN_POINT ( 'NONE',  ( -39.30918829504999934, 27.97290950744599769, 64.35000000000000853 ) ) ;
#1219=VERTEX_POINT ( 'NONE', #5070 ) ;
#1220=DIRECTION ( 'NONE',  ( 0.000000000000000000, 0.000000000000000000, -1.000000000000000000 ) ) ;
#1226=AXIS2_PLACEMENT_3D ( 'NONE', #13677, #3850, #13600 ) ;
#1227=EDGE_CURVE ( 'NONE', #1958, #10203, #10982, .T. ) ;
#1228=ORIENTED_EDGE ( 'NONE', *, *, #13497, .F. ) ;
#1231=ORIENTED_EDGE ( 'NONE', *, *, #5670, .T. ) ;
#1232=DIRECTION ( 'NONE',  ( 0.4528443260392606695, 0.8915896008669279560, 0.000000000000000000 ) ) ;
#1234=DIRECTION ( 'NONE',  ( 0.000000000000000000, 0.000000000000000000, -1.000000000000000000 ) ) ;
#1236=LINE ( 'NONE', #3086, #12541 ) ;
#1238=LINE ( 'NONE', #12982, #4262 ) ;
#1240=CARTESIAN_POINT ( 'NONE',  ( -18.05918829504999934, 10.97290950744599947, 58.54999999999999716 ) ) ;
#1241=DIRECTION ( 'NONE',  ( 0.000000000000000000, 0.000000000000000000, -1.000000000000000000 ) ) ;
#1242=ORIENTED_EDGE ( 'NONE', *, *, #6372, .T. ) ;
#1244=EDGE_CURVE ( 'NONE', #11891, #1905, #6044, .T. ) ;
#1247=CARTESIAN_POINT ( 'NONE',  ( -15.75124634074425956, 30.24535125669912716, 53.87933641254778649 ) ) ;
#1248=LINE ( 'NONE', #7515, #9967 ) ;
#1252=ORIENTED_EDGE ( 'NONE', *, *, #4145, .T. ) ;
#1253=CARTESIAN_POINT ( 'NONE',  ( -12.69835982676941910, -4.028726038184999858, 62.14999999999999858 ) ) ;
#1260=ORIENTED_EDGE ( 'NONE', *, *, #10582, .F. ) ;
#1261=VERTEX_POINT ( 'NONE', #7222 ) ;
#1262=PLANE ( 'NONE',  #1009 ) ;
#1264=VERTEX_POINT ( 'NONE', #11367 ) ;
#1266=VECTOR ( 'NONE', #6258, 1000.000000000000000 ) ;
#1267=ADVANCED_FACE ( 'NONE', ( #9479 ), #1874, .T. ) ;
#1269=CARTESIAN_POINT ( 'NONE',  ( -28.87730642030694739, 29.81324547859995278, 83.57661607529820458 ) ) ;
#1273=CARTESIAN_POINT ( 'NONE',  ( -23.42001676333060090, -4.028726038184999858, 62.14999999999999858 ) ) ;
#1274=CARTESIAN_POINT ( 'NONE',  ( -18.88016301897669891, 16.91647750172969822, 64.85000000000000853 ) ) ;
#1275=CARTESIAN_POINT ( 'NONE',  ( -18.05918829504999934, 10.97290950744599947, 62.14999999999999858 ) ) ;
#1276=VECTOR ( 'NONE', #1860, 1000.000000000000000 ) ;
#1279=VERTEX_POINT ( 'NONE', #13724 ) ;
#1281=VERTEX_POINT ( 'NONE', #9338 ) ;
#1282=EDGE_CURVE ( 'NONE', #6154, #1279, #5373, .T. ) ;
#1283=FACE_OUTER_BOUND ( 'NONE', #1055, .T. ) ;
#1284=CIRCLE ( 'NONE', #7510, 6.299999999999998046 ) ;
#1287=CONICAL_SURFACE ( 'NONE', #5299, 16.95000000000000284, 0.7853981633974433940 ) ;
#1290=AXIS2_PLACEMENT_3D ( 'NONE', #10171, #9189, #2921 ) ;
#1291=CARTESIAN_POINT ( 'NONE',  ( -19.57774717906803374, 30.31058478656889932, 53.35224432894259650 ) ) ;
#1292=CARTESIAN_POINT ( 'NONE',  ( -2.059188295050000228, 10.97290950744599947, 7.250000000000000000 ) ) ;
#1293=ORIENTED_EDGE ( 'NONE', *, *, #4670, .T. ) ;
#1294=DIRECTION ( 'NONE',  ( 0.000000000000000000, 1.000000000000000000, 0.000000000000000000 ) ) ;
#1295=DIRECTION ( 'NONE',  ( -1.000000000000000000, 0.000000000000000000, 0.000000000000000000 ) ) ;
#1296=CARTESIAN_POINT ( 'NONE',  ( -15.41280400920135030, 7.973467857469549891, 27.30000000000000071 ) ) ;
#1298=AXIS2_PLACEMENT_3D ( 'NONE', #9090, #13349, #2770 ) ;
#1304=ORIENTED_EDGE ( 'NONE', *, *, #7232, .F. ) ;
#1306=LINE ( 'NONE', #2243, #817 ) ;
#1308=DIRECTION ( 'NONE',  ( -1.000000000000000000, 0.000000000000000000, 0.000000000000000000 ) ) ;
#1311=VECTOR ( 'NONE', #10141, 1000.000000000000000 ) ;
#1313=CARTESIAN_POINT ( 'NONE',  ( -14.75120793773922045, 7.223607444975439940, 68.84999999999999432 ) ) ;
#1315=CARTESIAN_POINT ( 'NONE',  ( -18.05918829504999934, 10.97290950744599947, 56.84999999999999432 ) ) ;
#1316=CIRCLE ( 'NONE', #4639, 3.449999999999999734 ) ;
#1319=ADVANCED_FACE ( 'NONE', ( #1086 ), #3472, .T. ) ;
#1321=CARTESIAN_POINT ( 'NONE',  ( -15.59876235566975744, 30.22970645086915198, 54.01720515842198012 ) ) ;
#1323=ORIENTED_EDGE ( 'NONE', *, *, #6995, .T. ) ;
#1326=DIRECTION ( 'NONE',  ( 0.000000000000000000, 0.000000000000000000, -1.000000000000000000 ) ) ;
#1329=EDGE_CURVE ( 'NONE', #11446, #5675, #3215, .T. ) ;
#1330=DIRECTION ( 'NONE',  ( 4.866859854469739928E-30, 2.732534507816520408E-15, 1.000000000000000000 ) ) ;
#1332=LINE ( 'NONE', #429, #5353 ) ;
#1333=AXIS2_PLACEMENT_3D ( 'NONE', #2821, #5923, #8031 ) ;
#1334=VECTOR ( 'NONE', #1010, 1000.000000000000000 ) ;
#1335=ORIENTED_EDGE ( 'NONE', *, *, #6857, .T. ) ;
#1336=ORIENTED_EDGE ( 'NONE', *, *, #1950, .F. ) ;
#1338=DIRECTION ( 'NONE',  ( 0.6615960714621569316, -0.7498604124941123938, 0.000000000000000000 ) ) ;
#1341=AXIS2_PLACEMENT_3D ( 'NONE', #3898, #12351, #2799 ) ;
#1344=CONICAL_SURFACE ( 'NONE', #11169, 6.145833333000000565, 0.7853981633974503884 ) ;
#1347=DIRECTION ( 'NONE',  ( 1.000000000000000000, 0.000000000000000000, 0.000000000000000000 ) ) ;
#1348=EDGE_CURVE ( 'NONE', #12241, #3252, #9630, .T. ) ;
#1349=FACE_OUTER_BOUND ( 'NONE', #5034, .T. ) ;
#1351=CARTESIAN_POINT ( 'NONE',  ( -34.78181777225609750, 10.00028003023991907, 62.14999999999999858 ) ) ;
#1354=AXIS2_PLACEMENT_3D ( 'NONE', #12587, #4972, #11466 ) ;
#1355=CIRCLE ( 'NONE', #10736, 17.00000000000000355 ) ;
#1358=ORIENTED_EDGE ( 'NONE', *, *, #9793, .F. ) ;
#1359=ORIENTED_EDGE ( 'NONE', *, *, #2598, .T. ) ;
#1360=DIRECTION ( 'NONE',  ( 0.000000000000000000, 0.000000000000000000, -1.000000000000000000 ) ) ;
#1361=ORIENTED_EDGE ( 'NONE', *, *, #9651, .T. ) ;
#1366=CARTESIAN_POINT ( 'NONE',  ( -21.77521107841160131, 30.06124217889628270, 58.40862893704163383 ) ) ;
#1367=AXIS2_PLACEMENT_3D ( 'NONE', #5789, #6709, #8951 ) ;
#1368=VECTOR ( 'NONE', #4300, 1000.000000000000000 ) ;
#1370=DIRECTION ( 'NONE',  ( 0.000000000000000000, 0.000000000000000000, 1.000000000000000000 ) ) ;
#1372=CARTESIAN_POINT ( 'NONE',  ( -9.663354962050000552, 10.97290950744599947, 60.75000000000000000 ) ) ;
#1374=CARTESIAN_POINT ( 'NONE',  ( -16.55918829504999579, 28.64232754551664684, 57.35000000000000142 ) ) ;
#1377=CIRCLE ( 'NONE', #930, 17.00000000000000355 ) ;
#1378=ORIENTED_EDGE ( 'NONE', *, *, #1864, .T. ) ;
#1379=ORIENTED_EDGE ( 'NONE', *, *, #5655, .F. ) ;
#1386=DIRECTION ( 'NONE',  ( -0.000000000000000000, -0.000000000000000000, 1.000000000000000000 ) ) ;
#1387=DIRECTION ( 'NONE',  ( 1.000000000000000000, 0.000000000000000000, 0.000000000000000000 ) ) ;
#1388=LINE ( 'NONE', #342, #7140 ) ;
#1389=CIRCLE ( 'NONE', #3641, 8.395833332999998788 ) ;
#1390=DIRECTION ( 'NONE',  ( 1.000000000000000000, -8.410780489584519664E-16, 0.000000000000000000 ) ) ;
#1392=UNCERTAINTY_MEASURE_WITH_UNIT (LENGTH_MEASURE( 1.000000000000000082E-05 ), #1947, 'distance_accuracy_value', 'NONE');
#1394=EDGE_CURVE ( 'NONE', #7753, #7807, #8288, .T. ) ;
#1396=ORIENTED_EDGE ( 'NONE', *, *, #8194, .T. ) ;
#1397=DIRECTION ( 'NONE',  ( 1.000000000000000000, 0.000000000000000000, 0.000000000000000000 ) ) ;
#1398=ORIENTED_EDGE ( 'NONE', *, *, #11335, .T. ) ;
#1400=CARTESIAN_POINT ( 'NONE',  ( -18.05918829504999934, 10.97290950744599947, 67.84999999999999432 ) ) ;
#1402=LINE ( 'NONE', #11048, #7524 ) ;
#1403=( BOUNDED_CURVE ( )  B_SPLINE_CURVE ( 3, ( #5809, #3725, #7972, #9944 ),
 .UNSPECIFIED., .F., .F. ) 
 B_SPLINE_CURVE_WITH_KNOTS ( ( 4, 4 ),
 ( 0.06314145699999899886, 0.9368585429999889413 ),
 .UNSPECIFIED. ) 
 CURVE ( )  GEOMETRIC_REPRESENTATION_ITEM ( )  RATIONAL_B_SPLINE_CURVE ( ( 0.9565783021659940433, 0.7697947703959779897, 0.7697947703959749921, 0.9565783021659860497 ) ) 
 REPRESENTATION_ITEM ( '' )  );
#1404=FACE_OUTER_BOUND ( 'NONE', #8374, .T. ) ;
#1405=DIRECTION ( 'NONE',  ( 2.612535355386759959E-17, 0.000000000000000000, 1.000000000000000000 ) ) ;
#1406=AXIS2_PLACEMENT_3D ( 'NONE', #7837, #5605, #6651 ) ;
#1408=ORIENTED_EDGE ( 'NONE', *, *, #6290, .T. ) ;
#1410=EDGE_CURVE ( 'NONE', #10847, #759, #5593, .T. ) ;
#1412=CARTESIAN_POINT ( 'NONE',  ( -34.25918829536686872, 2.872909506853352557, 63.35000000001154774 ) ) ;
#1414=ORIENTED_EDGE ( 'NONE', *, *, #8081, .T. ) ;
#1415=CIRCLE ( 'NONE', #9457, 7.150000000000001243 ) ;
#1418=CARTESIAN_POINT ( 'NONE',  ( -18.05918829504999934, 10.97290950744599947, 60.85000000000000142 ) ) ;
#1420=VERTEX_POINT ( 'NONE', #793 ) ;
#1423=CARTESIAN_POINT ( 'NONE',  ( -1.059188295049996231, -6.027090492554000534, 64.85000000000000853 ) ) ;
#1426=ADVANCED_FACE ( 'NONE', ( #235 ), #7590, .F. ) ;
#1427=EDGE_LOOP ( 'NONE', ( #893, #4786, #13084, #12703 ) ) ;
#1431=FACE_OUTER_BOUND ( 'NONE', #8321, .T. ) ;
#1433=CARTESIAN_POINT ( 'NONE',  ( -20.58544311336878962, 30.22252884699266673, 60.61712719099885760 ) ) ;
#1434=ORIENTED_EDGE ( 'NONE', *, *, #13277, .F. ) ;
#1435=CARTESIAN_POINT ( 'NONE',  ( -35.05918829505000645, -6.027090492554000534, 83.57661607529820458 ) ) ;
#1439=EDGE_CURVE ( 'NONE', #3793, #7909, #4068, .T. ) ;
#1440=VERTEX_POINT ( 'NONE', #7338 ) ;
#1442=LINE ( 'NONE', #471, #4155 ) ;
#1446=LINE ( 'NONE', #8851, #5059 ) ;
#1448=FACE_OUTER_BOUND ( 'NONE', #13325, .T. ) ;
#1451=DIRECTION ( 'NONE',  ( 0.000000000000000000, 0.000000000000000000, -1.000000000000000000 ) ) ;
#1452=DIRECTION ( 'NONE',  ( 0.000000000000000000, 0.000000000000000000, 1.000000000000000000 ) ) ;
#1453=CARTESIAN_POINT ( 'NONE',  ( -30.30918829504999934, -6.027090492554000534, 64.85000000000000853 ) ) ;
#1455=CARTESIAN_POINT ( 'NONE',  ( -18.05918829504999934, 10.97290950744599947, 7.250000000000000000 ) ) ;
#1457=ORIENTED_EDGE ( 'NONE', *, *, #10898, .F. ) ;
#1459=FACE_OUTER_BOUND ( 'NONE', #9173, .T. ) ;
#1460=ORIENTED_EDGE ( 'NONE', *, *, #70, .T. ) ;
#1465=EDGE_CURVE ( 'NONE', #13804, #13429, #12960, .T. ) ;
#1467=DIRECTION ( 'NONE',  ( 0.000000000000000000, -1.000000000000000000, 0.000000000000000000 ) ) ;
#1468=FACE_BOUND ( 'NONE', #12423, .T. ) ;
#1471=AXIS2_PLACEMENT_3D ( 'NONE', #9039, #1639, #8322 ) ;
#1473=CARTESIAN_POINT ( 'NONE',  ( -18.05918829504999934, 21.47290950744600124, 57.35000000000000142 ) ) ;
#1477=ORIENTED_EDGE ( 'NONE', *, *, #865, .T. ) ;
#1478=DIRECTION ( 'NONE',  ( 0.000000000000000000, 0.000000000000000000, 1.000000000000000000 ) ) ;
#1480=CARTESIAN_POINT ( 'NONE',  ( -18.05918829504999934, 10.97290950744599947, 118.8499999999999943 ) ) ;
#1482=AXIS2_PLACEMENT_3D ( 'NONE', #5818, #8768, #4514 ) ;
#1483=CARTESIAN_POINT ( 'NONE',  ( -24.37001676333060018, -4.028726038184999858, 62.14999999999999858 ) ) ;
#1484=CARTESIAN_POINT ( 'NONE',  ( -16.85695709240152951, 26.92898083073637494, 56.44676063695975188 ) ) ;
#1485=EDGE_CURVE ( 'NONE', #11380, #936, #11628, .T. ) ;
#1486=CARTESIAN_POINT ( 'NONE',  ( -18.05918829504999934, 10.97290950744599947, 62.14999999999999858 ) ) ;
#1487=EDGE_CURVE ( 'NONE', #11722, #6370, #1136, .T. ) ;
#1488=EDGE_CURVE ( 'NONE', #10360, #2746, #8543, .T. ) ;
#1489=ORIENTED_EDGE ( 'NONE', *, *, #11587, .T. ) ;
#1491=VERTEX_POINT ( 'NONE', #5455 ) ;
#1494=LINE ( 'NONE', #526, #7505 ) ;
#1495=CARTESIAN_POINT ( 'NONE',  ( -20.84535740604768250, 30.19258199390759145, 60.33062495464709940 ) ) ;
#1496=LINE ( 'NONE', #11920, #1629 ) ;
#1497=DIRECTION ( 'NONE',  ( 0.3132098788326365124, -0.9496839325805429555, 0.000000000000000000 ) ) ;
#1499=CARTESIAN_POINT ( 'NONE',  ( -18.05918829504999934, 10.97290950744599947, 63.14999999999999858 ) ) ;
#1501=COLOUR_RGB ( '', 0.72549020, 0.75294118, 0.79215686) ;
#1507=AXIS2_PLACEMENT_3D ( 'NONE', #3121, #3758, #2073 ) ;
#1508=CARTESIAN_POINT ( 'NONE',  ( -18.05918829504999934, 10.97290950744599947, 31.09999999999999787 ) ) ;
#1510=DIRECTION ( 'NONE',  ( 0.8915896008669277339, -0.4528443260392608916, 0.000000000000000000 ) ) ;
#1511=FACE_OUTER_BOUND ( 'NONE', #6643, .T. ) ;
#1512=CARTESIAN_POINT ( 'NONE',  ( -18.05918829504999934, 10.97290950744599947, 64.85000000000000853 ) ) ;
#1513=CARTESIAN_POINT ( 'NONE',  ( -10.38347696868452097, 26.08535324214045303, 60.85000000000000142 ) ) ;
#1514=EDGE_CURVE ( 'NONE', #8485, #3005, #5525, .T. ) ;
#1516=CARTESIAN_POINT ( 'NONE',  ( -9.759188295050000406, 10.97290950744599947, 63.14999999999999858 ) ) ;
#1517=CARTESIAN_POINT ( 'NONE',  ( -14.95720466168106100, 17.08029827338444662, 61.25000000000000000 ) ) ;
#1521=FACE_OUTER_BOUND ( 'NONE', #2833, .T. ) ;
#1522=AXIS2_PLACEMENT_3D ( 'NONE', #13541, #9363, #3089 ) ;
#1523=AXIS2_PLACEMENT_3D ( 'NONE', #5451, #4423, #2834 ) ;
#1524=CIRCLE ( 'NONE', #1746, 34.69999999999999574 ) ;
#1525=CIRCLE ( 'NONE', #7516, 3.000000000000000888 ) ;
#1526=ADVANCED_FACE ( 'NONE', ( #9672, #3311 ), #9524, .T. ) ;
#1527=UNCERTAINTY_MEASURE_WITH_UNIT (LENGTH_MEASURE( 1.000000000000000082E-05 ), #2265, 'distance_accuracy_value', 'NONE');
#1528=EDGE_CURVE ( 'NONE', #2555, #12583, #256, .T. ) ;
#1529=EDGE_LOOP ( 'NONE', ( #7431, #11443 ) ) ;
#1530=VERTEX_POINT ( 'NONE', #7616 ) ;
#1531=MECHANICAL_DESIGN_GEOMETRIC_PRESENTATION_REPRESENTATION('',(#9796),#10238);
#1535=CARTESIAN_POINT ( 'NONE',  ( -1.059188295049996231, 10.97290950744599947, 57.35000000000000142 ) ) ;
#1536=AXIS2_PLACEMENT_3D ( 'NONE', #515, #10094, #7614 ) ;
#1538=CARTESIAN_POINT ( 'NONE',  ( -18.05918829504999934, 28.64232754551664684, 57.35000000000000142 ) ) ;
#1539=DIRECTION ( 'NONE',  ( 0.4528443260392610026, 0.8915896008669278450, 0.000000000000000000 ) ) ;
#1540=EDGE_CURVE ( 'NONE', #10854, #13546, #9597, .T. ) ;
#1541=DIRECTION ( 'NONE',  ( 0.000000000000000000, 0.000000000000000000, 1.000000000000000000 ) ) ;
#1542=FACE_OUTER_BOUND ( 'NONE', #12537, .T. ) ;
#1543=ADVANCED_FACE ( 'NONE', ( #9812 ), #3195, .T. ) ;
#1546=EDGE_CURVE ( 'NONE', #10428, #6071, #1377, .T. ) ;
#1548=ORIENTED_EDGE ( 'NONE', *, *, #5160, .F. ) ;
#1549=ORIENTED_EDGE ( 'NONE', *, *, #12646, .F. ) ;
#1550=CARTESIAN_POINT ( 'NONE',  ( -17.37799943181128626, 30.35031926759487675, 61.63905248387093394 ) ) ;
#1553=EDGE_LOOP ( 'NONE', ( #3942, #7911, #7578, #6630, #552, #7539, #7897, #7173, #3995, #4191, #5278, #1888, #2472, #13515, #9187, #10950, #53, #11982, #4644, #8269, #4358 ) ) ;
#1555=DIRECTION ( 'NONE',  ( -1.000000000000000000, 0.000000000000000000, 0.000000000000000000 ) ) ;
#1558=DIRECTION ( 'NONE',  ( 0.000000000000000000, 0.000000000000000000, 1.000000000000000000 ) ) ;
#1559=CIRCLE ( 'NONE', #4687, 17.00000000000000355 ) ;
#1560=FACE_OUTER_BOUND ( 'NONE', #1201, .T. ) ;
#1562=CYLINDRICAL_SURFACE ( 'NONE', #11812, 8.250000000000001776 ) ;
#1563=CARTESIAN_POINT ( 'NONE',  ( -11.06274345774342116, 24.74796884084004844, 57.35000000000000142 ) ) ;
#1566=EDGE_CURVE ( 'NONE', #1261, #6644, #5611, .T. ) ;
#1570=CARTESIAN_POINT ( 'NONE',  ( -21.31400196563854266, 30.13112197624766964, 59.63668312139478900 ) ) ;
#1571=FACE_OUTER_BOUND ( 'NONE', #13452, .T. ) ;
#1572=FACE_OUTER_BOUND ( 'NONE', #2832, .T. ) ;
#1574=DIRECTION ( 'NONE',  ( -1.000000000000000000, 0.000000000000000000, 0.000000000000000000 ) ) ;
#1575=CYLINDRICAL_SURFACE ( 'NONE', #8023, 4.749999999999997335 ) ;
#1576=CIRCLE ( 'NONE', #12727, 4.750000000000000000 ) ;
#1579=AXIS2_PLACEMENT_3D ( 'NONE', #3244, #2063, #927 ) ;
#1581=ORIENTED_EDGE ( 'NONE', *, *, #12580, .F. ) ;
#1584=AXIS2_PLACEMENT_3D ( 'NONE', #12805, #10716, #1202 ) ;
#1588=CYLINDRICAL_SURFACE ( 'NONE', #1341, 8.395833332999997012 ) ;
#1589=CARTESIAN_POINT ( 'NONE',  ( -11.75918829505000041, 10.97290950744599947, 61.86500000000000199 ) ) ;
#1590=FACE_OUTER_BOUND ( 'NONE', #6386, .T. ) ;
#1591=CARTESIAN_POINT ( 'NONE',  ( -38.38077571930825371, 22.44393519180574970, 17.25000000000000000 ) ) ;
#1595=CARTESIAN_POINT ( 'NONE',  ( -12.69835982676941910, -4.028726038184999858, 63.45000000000000284 ) ) ;
#1597=DIRECTION ( 'NONE',  ( 0.000000000000000000, 0.000000000000000000, -1.000000000000000000 ) ) ;
#1598=EDGE_CURVE ( 'NONE', #318, #1219, #8736, .T. ) ;
#1600=AXIS2_PLACEMENT_3D ( 'NONE', #6949, #10176, #10041 ) ;
#1601=ORIENTED_EDGE ( 'NONE', *, *, #4222, .T. ) ;
#1604=VERTEX_POINT ( 'NONE', #5732 ) ;
#1605=DIRECTION ( 'NONE',  ( -1.000000000000000000, 0.000000000000000000, 0.000000000000000000 ) ) ;
#1610=CARTESIAN_POINT ( 'NONE',  ( -1.059188295049996231, 27.97290950744599769, 64.35000000000000853 ) ) ;
#1615=VECTOR ( 'NONE', #5971, 1000.000000000000000 ) ;
#1618=DIRECTION ( 'NONE',  ( 0.000000000000000000, 0.000000000000000000, 1.000000000000000000 ) ) ;
#1621=ORIENTED_EDGE ( 'NONE', *, *, #1485, .F. ) ;
#1623=ORIENTED_EDGE ( 'NONE', *, *, #4075, .T. ) ;
#1624=CARTESIAN_POINT ( 'NONE',  ( -18.05918829504999934, 10.97290950744599947, 63.45000000000000284 ) ) ;
#1629=VECTOR ( 'NONE', #6805, 1000.000000000000000 ) ;
#1630=DIRECTION ( 'NONE',  ( 1.000000000000000000, 0.000000000000000000, 0.000000000000000000 ) ) ;
#1633=VERTEX_POINT ( 'NONE', #6732 ) ;
#1634=ORIENTED_EDGE ( 'NONE', *, *, #10598, .F. ) ;
#1635=AXIS2_PLACEMENT_3D ( 'NONE', #6619, #924, #3431 ) ;
#1636=VERTEX_POINT ( 'NONE', #7836 ) ;
#1637=ORIENTED_EDGE ( 'NONE', *, *, #12185, .T. ) ;
#1638=ORIENTED_EDGE ( 'NONE', *, *, #13674, .T. ) ;
#1639=DIRECTION ( 'NONE',  ( 0.000000000000000000, 0.000000000000000000, 1.000000000000000000 ) ) ;
#1640=CARTESIAN_POINT ( 'NONE',  ( -16.55918829504999579, 27.90660372932210009, 57.35000000000000142 ) ) ;
#1641=CARTESIAN_POINT ( 'NONE',  ( -20.70149429739183944, 30.20956267044833865, 60.49614159523773793 ) ) ;
#1642=DIRECTION ( 'NONE',  ( 0.000000000000000000, -1.000000000000000000, 1.672022627447524796E-15 ) ) ;
#1643=DIRECTION ( 'NONE',  ( -2.267612386897784912E-16, 1.000000000000000000, 0.000000000000000000 ) ) ;
#1646=CARTESIAN_POINT ( 'NONE',  ( -18.05918829504999934, 14.81548537210212046, 5.250000000000000000 ) ) ;
#1653=CARTESIAN_POINT ( 'NONE',  ( -30.48673169511680214, 10.97290950744599947, 17.25000000000000000 ) ) ;
#1654=CARTESIAN_POINT ( 'NONE',  ( -18.05918829504999934, 10.97290950744599947, 23.90000000000000213 ) ) ;
#1655=DIRECTION ( 'NONE',  ( -1.000000000000000000, 0.000000000000000000, 0.000000000000000000 ) ) ;
#1657=LINE ( 'NONE', #12482, #1615 ) ;
#1659=LINE ( 'NONE', #8662, #11567 ) ;
#1661=DIRECTION ( 'NONE',  ( -0.9496839325805428444, -0.3132098788326364569, 0.000000000000000000 ) ) ;
#1663=CARTESIAN_POINT ( 'NONE',  ( -7.241070169793059286, -7.867426463707969830, 17.25000000000000000 ) ) ;
#1664=EDGE_CURVE ( 'NONE', #2189, #3894, #5167, .T. ) ;
#1665=ADVANCED_FACE ( 'NONE', ( #7903 ), #5879, .T. ) ;
#1667=VERTEX_POINT ( 'NONE', #11132 ) ;
#1673=LINE ( 'NONE', #4757, #6249 ) ;
#1676=AXIS2_PLACEMENT_3D ( 'NONE', #13416, #5794, #8171 ) ;
#1677=CARTESIAN_POINT ( 'NONE',  ( -18.05918829504999223, 19.18892026044601096, 63.36264408500002787 ) ) ;
#1678=DIRECTION ( 'NONE',  ( 0.000000000000000000, 0.000000000000000000, -1.000000000000000000 ) ) ;
#1679=EDGE_CURVE ( 'NONE', #13687, #10707, #1403, .T. ) ;
#1681=ADVANCED_FACE ( 'NONE', ( #1349 ), #3523, .F. ) ;
#1682=ORIENTED_EDGE ( 'NONE', *, *, #3550, .F. ) ;
#1685=CARTESIAN_POINT ( 'NONE',  ( -17.32805791519659522, 30.34876749365187720, 61.62799931076499860 ) ) ;
#1686=ORIENTED_EDGE ( 'NONE', *, *, #688, .T. ) ;
#1687=VERTEX_POINT ( 'NONE', #4567 ) ;
#1688=CARTESIAN_POINT ( 'NONE',  ( -1.336558817843898073, 10.00028003023991907, 63.45000000000000284 ) ) ;
#1691=DIRECTION ( 'NONE',  ( -1.000000000000000000, 0.000000000000000000, 0.000000000000000000 ) ) ;
#1692=FACE_OUTER_BOUND ( 'NONE', #8193, .T. ) ;
#1695=CARTESIAN_POINT ( 'NONE',  ( -18.25896549665364432, 27.97289716965712358, 58.84983448222843805 ) ) ;
#1699=ORIENTED_EDGE ( 'NONE', *, *, #4145, .F. ) ;
#1701=ORIENTED_EDGE ( 'NONE', *, *, #1854, .T. ) ;
#1703=AXIS2_PLACEMENT_3D ( 'NONE', #3465, #2364, #248 ) ;
#1704=DIRECTION ( 'NONE',  ( 0.000000000000000000, 0.000000000000000000, -1.000000000000000000 ) ) ;
#1705=CARTESIAN_POINT ( 'NONE',  ( -20.33293068681281923, 30.24873049275584691, 60.84977818423778473 ) ) ;
#1707=CARTESIAN_POINT ( 'NONE',  ( -18.05918829504999934, 10.97290950744599947, 60.75000000000000000 ) ) ;
#1708=DIRECTION ( 'NONE',  ( 0.4528443260392608916, 0.8915896008669279560, 0.000000000000000000 ) ) ;
#1712=EDGE_LOOP ( 'NONE', ( #6233, #12262, #6482, #5448 ) ) ;
#1713=AXIS2_PLACEMENT_3D ( 'NONE', #9012, #13263, #11589 ) ;
#1714=EDGE_CURVE ( 'NONE', #12649, #2384, #8715, .T. ) ;
#1715=EDGE_LOOP ( 'NONE', ( #8381, #3310, #9397, #11626 ) ) ;
#1720=DIRECTION ( 'NONE',  ( 0.4528443260392608916, 0.8915896008669277339, 0.000000000000000000 ) ) ;
#1721=CARTESIAN_POINT ( 'NONE',  ( -5.809188295050001116, -6.027090492554000534, 64.85000000000000853 ) ) ;
#1722=AXIS2_PLACEMENT_3D ( 'NONE', #1168, #2319, #12976 ) ;
#1724=CARTESIAN_POINT ( 'NONE',  ( -35.55918829505000645, 10.97290950744599947, 64.85000000000000853 ) ) ;
#1725=CARTESIAN_POINT ( 'NONE',  ( -22.68187722381259519, 13.56225431454274677, 68.55150892931679607 ) ) ;
#1728=DIRECTION ( 'NONE',  ( 1.000000000000000000, 0.000000000000000000, 0.000000000000000000 ) ) ;
#1733=CIRCLE ( 'NONE', #8449, 6.000000000000002665 ) ;
#1734=AXIS2_PLACEMENT_3D ( 'NONE', #5337, #1018, #3331 ) ;
#1735=VERTEX_POINT ( 'NONE', #3797 ) ;
#1737=ORIENTED_EDGE ( 'NONE', *, *, #8744, .F. ) ;
#1738=EDGE_CURVE ( 'NONE', #5595, #11930, #4484, .T. ) ;
#1739=ADVANCED_FACE ( 'NONE', ( #1985, #7256 ), #8123, .F. ) ;
#1740=ORIENTED_EDGE ( 'NONE', *, *, #8433, .T. ) ;
#1741=CARTESIAN_POINT ( 'NONE',  ( -20.80749866017044880, 15.21600409713747304, 68.79477705781098962 ) ) ;
#1742=DIRECTION ( 'NONE',  ( 0.4528443260392608916, 0.8915896008669277339, 0.000000000000000000 ) ) ;
#1743=VECTOR ( 'NONE', #2328, 1000.000000000000000 ) ;
#1744=CARTESIAN_POINT ( 'NONE',  ( -18.05918829504999934, 10.97290950744599947, 64.85000000000000853 ) ) ;
#1746=AXIS2_PLACEMENT_3D ( 'NONE', #5773, #483, #3965 ) ;
#1748=AXIS2_PLACEMENT_3D ( 'NONE', #1918, #10241, #7069 ) ;
#1749=CARTESIAN_POINT ( 'NONE',  ( -18.05918829504999934, 2.673908674445999889, 63.13003331699999876 ) ) ;
#1750=CARTESIAN_POINT ( 'NONE',  ( -25.86749127492459976, 30.80589556422609832, 5.250000000000000000 ) ) ;
#1753=EDGE_CURVE ( 'NONE', #13237, #7790, #1807, .T. ) ;
#1754=VECTOR ( 'NONE', #10980, 1000.000000000000000 ) ;
#1756=CIRCLE ( 'NONE', #10916, 16.66282263685194920 ) ;
#1757=ORIENTED_EDGE ( 'NONE', *, *, #3815, .F. ) ;
#1758=AXIS2_PLACEMENT_3D ( 'NONE', #13253, #7796, #482 ) ;
#1760=CARTESIAN_POINT ( 'NONE',  ( -15.65696070512129268, 30.23571877985226664, 60.73654365824928192 ) ) ;
#1761=ADVANCED_FACE ( 'NONE', ( #12525 ), #10355, .F. ) ;
#1762=ORIENTED_EDGE ( 'NONE', *, *, #7451, .T. ) ;
#1763=SURFACE_STYLE_FILL_AREA ( #11400 ) ;
#1769=EDGE_LOOP ( 'NONE', ( #13762, #13610, #6302, #4328 ) ) ;
#1770=EDGE_CURVE ( 'NONE', #1905, #5559, #11471, .T. ) ;
#1774=AXIS2_PLACEMENT_3D ( 'NONE', #9931, #558, #1539 ) ;
#1775=DIRECTION ( 'NONE',  ( 0.000000000000000000, 0.000000000000000000, 1.000000000000000000 ) ) ;
#1780=EDGE_CURVE ( 'NONE', #11171, #1958, #578, .T. ) ;
#1783=CONICAL_SURFACE ( 'NONE', #4021, 16.00000000000000000, 0.7853981633974476129 ) ;
#1784=VERTEX_POINT ( 'NONE', #9246 ) ;
#1785=CARTESIAN_POINT ( 'NONE',  ( -18.05918829504999934, 10.97290950744599947, 61.86500000000000199 ) ) ;
#1787=DIRECTION ( 'NONE',  ( 0.4528443260392608916, 0.8915896008669279560, 0.000000000000000000 ) ) ;
#1789=CARTESIAN_POINT ( 'NONE',  ( -10.78334210919089919, 29.19143287883919768, 64.85000000000000853 ) ) ;
#1793=AXIS2_PLACEMENT_3D ( 'NONE', #5792, #9017, #13271 ) ;
#1795=ADVANCED_FACE ( 'NONE', ( #11537 ), #10284, .T. ) ;
#1797=EDGE_LOOP ( 'NONE', ( #899, #4051 ) ) ;
#1799=CARTESIAN_POINT ( 'NONE',  ( -35.05918829505000645, 10.97290950744599947, 64.35000000000000853 ) ) ;
#1800=CARTESIAN_POINT ( 'NONE',  ( -18.05918829504999934, 10.97290950744599947, 61.85000000000000142 ) ) ;
#1801=DIRECTION ( 'NONE',  ( 0.000000000000000000, 0.000000000000000000, 1.000000000000000000 ) ) ;
#1802=VECTOR ( 'NONE', #6818, 1000.000000000000000 ) ;
#1804=VECTOR ( 'NONE', #4144, 1000.000000000000000 ) ;
#1805=DIRECTION ( 'NONE',  ( -1.000000000000000000, 0.000000000000000000, 0.000000000000000000 ) ) ;
#1806=CARTESIAN_POINT ( 'NONE',  ( 1.640811704950000172, -6.027090492554000534, 58.85000000000000142 ) ) ;
#1807=CIRCLE ( 'NONE', #228, 2.700000000000000178 ) ;
#1808=FACE_OUTER_BOUND ( 'NONE', #7399, .T. ) ;
#1809=PLANE ( 'NONE',  #475 ) ;
#1810=EDGE_CURVE ( 'NONE', #194, #5817, #3936, .T. ) ;
#1812=FACE_BOUND ( 'NONE', #8651, .T. ) ;
#1818=VERTEX_POINT ( 'NONE', #6996 ) ;
#1820=CARTESIAN_POINT ( 'NONE',  ( -20.70557258089865016, 13.97235115742243927, 27.30000000000000071 ) ) ;
#1821=VERTEX_POINT ( 'NONE', #13352 ) ;
#1822=VERTEX_POINT ( 'NONE', #11270 ) ;
#1824=CARTESIAN_POINT ( 'NONE',  ( -18.05918829504999934, 14.81548537210212046, 64.85000000000000853 ) ) ;
#1825=DIRECTION ( 'NONE',  ( -0.3984948954980490621, 0.000000000000000000, 0.9171705502587831349 ) ) ;
#1826=AXIS2_PLACEMENT_3D ( 'NONE', #8216, #3010, #12481 ) ;
#1828=AXIS2_PLACEMENT_3D ( 'NONE', #3461, #7621, #11906 ) ;
#1829=CARTESIAN_POINT ( 'NONE',  ( -1.059188295049996231, 27.97290950744599769, 64.85000000000000853 ) ) ;
#1832=EDGE_LOOP ( 'NONE', ( #8526, #8359, #2040, #9188, #3719, #8864, #8867, #3023, #5613, #8596, #1757, #6530, #6187, #11312, #2638 ) ) ;
#1834=VERTEX_POINT ( 'NONE', #643 ) ;
#1835=CARTESIAN_POINT ( 'NONE',  ( -15.83721163932141529, 30.25376030684627082, 60.89272510006725980 ) ) ;
#1836=ORIENTED_EDGE ( 'NONE', *, *, #1810, .T. ) ;
#1838=CARTESIAN_POINT ( 'NONE',  ( -18.05918829504999934, 10.97290950744599947, 61.86500000000000199 ) ) ;
#1839=ORIENTED_EDGE ( 'NONE', *, *, #7568, .F. ) ;
#1843=FACE_OUTER_BOUND ( 'NONE', #10573, .T. ) ;
#1844=DIRECTION ( 'NONE',  ( 0.000000000000000000, 0.000000000000000000, -1.000000000000000000 ) ) ;
#1845=DIRECTION ( 'NONE',  ( 0.4528443260392610581, 0.8915896008669278450, 0.000000000000000000 ) ) ;
#1847=EDGE_CURVE ( 'NONE', #8804, #5387, #1238, .T. ) ;
#1848=VERTEX_POINT ( 'NONE', #13696 ) ;
#1850=ORIENTED_EDGE ( 'NONE', *, *, #10144, .F. ) ;
#1852=VERTEX_POINT ( 'NONE', #9921 ) ;
#1853=AXIS2_PLACEMENT_3D ( 'NONE', #12468, #5052, #2924 ) ;
#1854=EDGE_CURVE ( 'NONE', #9534, #5483, #122, .T. ) ;
#1855=EDGE_LOOP ( 'NONE', ( #9780, #9648, #6092, #7714 ) ) ;
#1856=ORIENTED_EDGE ( 'NONE', *, *, #11943, .F. ) ;
#1857=DIRECTION ( 'NONE',  ( 0.000000000000000000, 0.000000000000000000, -1.000000000000000000 ) ) ;
#1858=CARTESIAN_POINT ( 'NONE',  ( -20.28967185382198224, 30.25294134169608995, 60.88576449748650532 ) ) ;
#1860=DIRECTION ( 'NONE',  ( 0.3202092937642119774, 0.6304490528084089052, 0.7071067811865507924 ) ) ;
#1864=EDGE_CURVE ( 'NONE', #8825, #2555, #11613, .T. ) ;
#1865=EDGE_CURVE ( 'NONE', #8537, #9462, #5639, .T. ) ;
#1866=EDGE_CURVE ( 'NONE', #6343, #8303, #1388, .T. ) ;
#1867=CARTESIAN_POINT ( 'NONE',  ( -2.059188295050000228, 10.97290950744599947, 64.85000000000000853 ) ) ;
#1868=EDGE_CURVE ( 'NONE', #12210, #5647, #8268, .T. ) ;
#1870=ORIENTED_EDGE ( 'NONE', *, *, #1865, .F. ) ;
#1871=DIRECTION ( 'NONE',  ( 0.2000659497483225358, -2.450101249776580428E-17, 0.9797824328652262604 ) ) ;
#1874=CYLINDRICAL_SURFACE ( 'NONE', #1826, 15.45000000000000462 ) ;
#1875=CARTESIAN_POINT ( 'NONE',  ( -22.74060393451187423, 13.51044018961873938, 68.52518719986740336 ) ) ;
#1876=ORIENTED_EDGE ( 'NONE', *, *, #11038, .F. ) ;
#1879=CARTESIAN_POINT ( 'NONE',  ( -16.40519811639460102, 9.098258476210720147, 53.85000000000000142 ) ) ;
#1881=FACE_OUTER_BOUND ( 'NONE', #13106, .T. ) ;
#1887=CARTESIAN_POINT ( 'NONE',  ( -18.05918829504999934, 21.47290950744600124, 57.35000000000000142 ) ) ;
#1888=ORIENTED_EDGE ( 'NONE', *, *, #4118, .T. ) ;
#1890=CARTESIAN_POINT ( 'NONE',  ( -18.05918829504999934, 10.97290950744599947, 61.72253826518770836 ) ) ;
#1891=CIRCLE ( 'NONE', #7214, 6.449999999999997513 ) ;
#1898=CARTESIAN_POINT ( 'NONE',  ( -14.68608402389303613, 30.11415384993292221, 59.40884097298657451 ) ) ;
#1903=DIRECTION ( 'NONE',  ( 0.000000000000000000, 0.000000000000000000, -1.000000000000000000 ) ) ;
#1905=VERTEX_POINT ( 'NONE', #12659 ) ;
#1906=DIRECTION ( 'NONE',  ( 0.000000000000000000, 0.000000000000000000, -1.000000000000000000 ) ) ;
#1908=DIRECTION ( 'NONE',  ( 1.000000000000000000, 0.000000000000000000, 0.000000000000000000 ) ) ;
#1909=CARTESIAN_POINT ( 'NONE',  ( -30.80918829504999934, -6.027090492554000534, 58.85000000000000142 ) ) ;
#1910=CARTESIAN_POINT ( 'NONE',  ( -35.05918829505000645, -6.027090492554000534, 17.25000000000000000 ) ) ;
#1911=DIRECTION ( 'NONE',  ( -1.000000000000000000, 0.000000000000000000, 0.000000000000000000 ) ) ;
#1912=AXIS2_PLACEMENT_3D ( 'NONE', #5352, #6403, #10673 ) ;
#1913=ORIENTED_EDGE ( 'NONE', *, *, #7508, .F. ) ;
#1918=CARTESIAN_POINT ( 'NONE',  ( -18.05918829504999934, 14.81548537210212046, 83.57661607529820458 ) ) ;
#1920=CARTESIAN_POINT ( 'NONE',  ( -19.69645725958885762, 30.30251685228200031, 61.28626485309589356 ) ) ;
#1923=ADVANCED_FACE ( 'NONE', ( #4142 ), #13390, .F. ) ;
#1924=FACE_OUTER_BOUND ( 'NONE', #6017, .T. ) ;
#1925=CARTESIAN_POINT ( 'NONE',  ( -18.05918829504999934, 10.97290950744599947, 57.35000000000000142 ) ) ;
#1929=EDGE_LOOP ( 'NONE', ( #10797, #758, #11962, #439, #12567, #2606 ) ) ;
#1931=DIRECTION ( 'NONE',  ( 0.4528443260392610581, 0.8915896008669278450, 0.000000000000000000 ) ) ;
#1932=FACE_OUTER_BOUND ( 'NONE', #10506, .T. ) ;
#1935=DIRECTION ( 'NONE',  ( 0.000000000000000000, 0.000000000000000000, -1.000000000000000000 ) ) ;
#1936=ADVANCED_FACE ( 'NONE', ( #278 ), #13049, .T. ) ;
#1937=DIRECTION ( 'NONE',  ( 0.000000000000000000, 0.000000000000000000, -1.000000000000000000 ) ) ;
#1938=LINE ( 'NONE', #13665, #7827 ) ;
#1941=EDGE_LOOP ( 'NONE', ( #150, #11027, #10349, #12721 ) ) ;
#1944=DIRECTION ( 'NONE',  ( 0.000000000000000000, 0.000000000000000000, 1.000000000000000000 ) ) ;
#1946=CARTESIAN_POINT ( 'NONE',  ( -25.64433075620760150, -3.961216307075045240, 58.54999999999999716 ) ) ;
#1947=( LENGTH_UNIT ( ) NAMED_UNIT ( * ) SI_UNIT ( .MILLI., .METRE. ) );
#1950=EDGE_CURVE ( 'NONE', #6107, #10154, #13176, .T. ) ;
#1951=AXIS2_PLACEMENT_3D ( 'NONE', #11496, #10450, #3896 ) ;
#1952=VERTEX_POINT ( 'NONE', #9453 ) ;
#1955=CARTESIAN_POINT ( 'NONE',  ( -13.40033457972183939, -4.525318844826149878, 62.14999999999999858 ) ) ;
#1956=ORIENTED_EDGE ( 'NONE', *, *, #11434, .F. ) ;
#1957=ORIENTED_EDGE ( 'NONE', *, *, #8761, .F. ) ;
#1958=VERTEX_POINT ( 'NONE', #3353 ) ;
#1959=ADVANCED_FACE ( 'NONE', ( #7586 ), #11874, .F. ) ;
#1960=DIRECTION ( 'NONE',  ( 0.000000000000000000, 0.000000000000000000, 1.000000000000000000 ) ) ;
#1961=DIRECTION ( 'NONE',  ( 0.000000000000000000, 0.000000000000000000, -1.000000000000000000 ) ) ;
#1962=EDGE_LOOP ( 'NONE', ( #2238, #8863, #4237, #11616, #13149 ) ) ;
#1964=DIRECTION ( 'NONE',  ( 0.000000000000000000, 0.000000000000000000, 1.000000000000000000 ) ) ;
#1968=AXIS2_PLACEMENT_3D ( 'NONE', #4094, #12539, #7269 ) ;
#1969=EDGE_CURVE ( 'NONE', #5251, #1420, #12949, .T. ) ;
#1970=VERTEX_POINT ( 'NONE', #4947 ) ;
#1971=ORIENTED_EDGE ( 'NONE', *, *, #8018, .T. ) ;
#1972=CARTESIAN_POINT ( 'NONE',  ( -15.84264309710664165, 30.25428168447941246, 60.89715136093798975 ) ) ;
#1976=ORIENTED_EDGE ( 'NONE', *, *, #5277, .T. ) ;
#1977=ADVANCED_FACE ( 'NONE', ( #13392 ), #4045, .T. ) ;
#1978=FACE_OUTER_BOUND ( 'NONE', #10922, .T. ) ;
#1980=CARTESIAN_POINT ( 'NONE',  ( -1.059188295049996231, 27.97290950744599769, 64.85000000000000853 ) ) ;
#1981=FACE_OUTER_BOUND ( 'NONE', #13011, .T. ) ;
#1982=ORIENTED_EDGE ( 'NONE', *, *, #9115, .T. ) ;
#1984=CARTESIAN_POINT ( 'NONE',  ( -16.40519811639460102, 9.098258476210720147, 53.85000000000000142 ) ) ;
#1985=FACE_BOUND ( 'NONE', #12473, .T. ) ;
#1987=LINE ( 'NONE', #850, #12912 ) ;
#1989=DIRECTION ( 'NONE',  ( 0.000000000000000000, -1.000000000000000000, 0.000000000000000000 ) ) ;
#1990=VECTOR ( 'NONE', #8575, 1000.000000000000000 ) ;
#1991=VECTOR ( 'NONE', #12937, 1000.000000000000000 ) ;
#1995=ORIENTED_EDGE ( 'NONE', *, *, #8301, .T. ) ;
#2003=CIRCLE ( 'NONE', #8447, 4.750000000000000000 ) ;
#2005=DIRECTION ( 'NONE',  ( 0.4528443260392608916, 0.8915896008669279560, 0.000000000000000000 ) ) ;
#2007=ORIENTED_EDGE ( 'NONE', *, *, #12117, .T. ) ;
#2009=CARTESIAN_POINT ( 'NONE',  ( -19.26123285687782172, 26.92898414971012144, 56.44653808050201604 ) ) ;
#2014=VERTEX_POINT ( 'NONE', #1453 ) ;
#2015=ORIENTED_EDGE ( 'NONE', *, *, #4918, .T. ) ;
#2016=EDGE_CURVE ( 'NONE', #6494, #5283, #8089, .T. ) ;
#2017=AXIS2_PLACEMENT_3D ( 'NONE', #1910, #5941, #784 ) ;
#2019=ORIENTED_EDGE ( 'NONE', *, *, #5327, .T. ) ;
#2021=LINE ( 'NONE', #12407, #2187 ) ;
#2022=ORIENTED_EDGE ( 'NONE', *, *, #5657, .T. ) ;
#2023=DIRECTION ( 'NONE',  ( 0.000000000000000000, 0.000000000000000000, -1.000000000000000000 ) ) ;
#2024=LINE ( 'NONE', #4038, #1266 ) ;
#2025=CARTESIAN_POINT ( 'NONE',  ( -35.05918829505000645, 27.97290950744599769, 17.25000000000000000 ) ) ;
#2026=DIRECTION ( 'NONE',  ( 1.000000000000000000, 0.000000000000000000, 0.000000000000000000 ) ) ;
#2028=DIRECTION ( 'NONE',  ( 0.000000000000000000, 0.000000000000000000, 1.000000000000000000 ) ) ;
#2030=DIRECTION ( 'NONE',  ( -1.000000000000000000, 0.000000000000000000, 0.000000000000000000 ) ) ;
#2031=AXIS2_PLACEMENT_3D ( 'NONE', #5718, #1330, #13065 ) ;
#2034=EDGE_CURVE ( 'NONE', #13684, #9242, #6963, .T. ) ;
#2037=LINE ( 'NONE', #6122, #4591 ) ;
#2038=VECTOR ( 'NONE', #10861, 1000.000000000000000 ) ;
#2039=AXIS2_PLACEMENT_3D ( 'NONE', #6487, #8723, #8393 ) ;
#2040=ORIENTED_EDGE ( 'NONE', *, *, #12628, .F. ) ;
#2041=ORIENTED_EDGE ( 'NONE', *, *, #8256, .F. ) ;
#2042=DIRECTION ( 'NONE',  ( 0.000000000000000000, 0.000000000000000000, -1.000000000000000000 ) ) ;
#2044=FACE_OUTER_BOUND ( 'NONE', #10676, .T. ) ;
#2045=DIRECTION ( 'NONE',  ( 0.000000000000000000, 0.000000000000000000, -1.000000000000000000 ) ) ;
#2046=CARTESIAN_POINT ( 'NONE',  ( -18.05918829504999934, 14.81548537210212046, 5.250000000000000000 ) ) ;
#2051=CARTESIAN_POINT ( 'NONE',  ( -14.69313762561336212, 30.11514052169665590, 55.27969735402319884 ) ) ;
#2052=ORIENTED_EDGE ( 'NONE', *, *, #10164, .F. ) ;
#2054=DIRECTION ( 'NONE',  ( 0.4678190685372707325, -0.5302313826179287926, 0.7071067811865475727 ) ) ;
#2055=ADVANCED_FACE ( 'NONE', ( #2806 ), #5586, .F. ) ;
#2056=AXIS2_PLACEMENT_3D ( 'NONE', #8028, #13265, #8803 ) ;
#2058=CARTESIAN_POINT ( 'NONE',  ( -25.86749127492460332, 30.80589556422609476, 83.57661607529820458 ) ) ;
#2061=DIRECTION ( 'NONE',  ( 0.000000000000000000, 0.000000000000000000, -1.000000000000000000 ) ) ;
#2063=DIRECTION ( 'NONE',  ( 0.000000000000000000, 0.000000000000000000, -1.000000000000000000 ) ) ;
#2064=EDGE_CURVE ( 'NONE', #10722, #5219, #5804, .T. ) ;
#2066=CIRCLE ( 'NONE', #9871, 34.69999999999999574 ) ;
#2067=ORIENTED_EDGE ( 'NONE', *, *, #13210, .F. ) ;
#2068=ORIENTED_EDGE ( 'NONE', *, *, #1780, .F. ) ;
#2070=ORIENTED_EDGE ( 'NONE', *, *, #9844, .F. ) ;
#2071=EDGE_CURVE ( 'NONE', #4627, #533, #8283, .T. ) ;
#2073=DIRECTION ( 'NONE',  ( -0.6615960714621564875, 0.7498604124941129490, 0.000000000000000000 ) ) ;
#2074=DIRECTION ( 'NONE',  ( 1.049727191138617833E-16, 0.5150380749100549327, -0.8571673007021118895 ) ) ;
#2075=VERTEX_POINT ( 'NONE', #2597 ) ;
#2077=AXIS2_PLACEMENT_3D ( 'NONE', #6263, #10806, #4378 ) ;
#2080=CARTESIAN_POINT ( 'NONE',  ( -10.44110272205000101, 10.97290950744599947, 61.65955166399999854 ) ) ;
#2081=DIRECTION ( 'NONE',  ( 0.000000000000000000, 0.000000000000000000, 1.000000000000000000 ) ) ;
#2082=VERTEX_POINT ( 'NONE', #1595 ) ;
#2085=LINE ( 'NONE', #11706, #7244 ) ;
#2088=CARTESIAN_POINT ( 'NONE',  ( -36.05918829505000645, 10.97290950744599947, 63.45000000000000284 ) ) ;
#2090=CARTESIAN_POINT ( 'NONE',  ( -0.3963656581980404825, 10.97290950744599947, 6.250000000000000000 ) ) ;
#2091=FILL_AREA_STYLE_COLOUR ( '', #10994 ) ;
#2092=CARTESIAN_POINT ( 'NONE',  ( -5.173045190668890569, -15.68519459986890041, 5.250000000000000000 ) ) ;
#2094=ADVANCED_FACE ( 'NONE', ( #12416 ), #6766, .F. ) ;
#2095=CARTESIAN_POINT ( 'NONE',  ( -25.05563313235659706, -2.802149825948039741, 57.35000000000000142 ) ) ;
#2096=CIRCLE ( 'NONE', #13448, 0.9499999999999995115 ) ;
#2097=CYLINDRICAL_SURFACE ( 'NONE', #13596, 4.750000000000000888 ) ;
#2104=ORIENTED_EDGE ( 'NONE', *, *, #2194, .F. ) ;
#2105=VERTEX_POINT ( 'NONE', #11100 ) ;
#2106=DIRECTION ( 'NONE',  ( -1.000000000000000000, 0.000000000000000000, 0.000000000000000000 ) ) ;
#2110=ORIENTED_EDGE ( 'NONE', *, *, #9459, .T. ) ;
#2111=CARTESIAN_POINT ( 'NONE',  ( -16.03669512066808878, 6.089431995824910793, 68.56428208524678780 ) ) ;
#2113=DIRECTION ( 'NONE',  ( 0.000000000000000000, 0.000000000000000000, -1.000000000000000000 ) ) ;
#2115=CARTESIAN_POINT ( 'NONE',  ( -18.05918829504999934, 10.97290950744599947, 62.14999999999999858 ) ) ;
#2117=EDGE_LOOP ( 'NONE', ( #1870, #3117, #10090, #5500, #145, #13107 ) ) ;
#2118=ORIENTED_EDGE ( 'NONE', *, *, #10161, .F. ) ;
#2121=DIRECTION ( 'NONE',  ( 0.000000000000000000, 0.000000000000000000, -1.000000000000000000 ) ) ;
#2123=FACE_BOUND ( 'NONE', #3187, .T. ) ;
#2126=DIRECTION ( 'NONE',  ( -0.4528443260392610026, -0.8915896008669278450, 0.000000000000000000 ) ) ;
#2127=EDGE_CURVE ( 'NONE', #9316, #10025, #6114, .T. ) ;
#2128=DIRECTION ( 'NONE',  ( 0.000000000000000000, 0.000000000000000000, -1.000000000000000000 ) ) ;
#2129=ADVANCED_FACE ( 'NONE', ( #13670, #811 ), #1809, .F. ) ;
#2130=ORIENTED_EDGE ( 'NONE', *, *, #5610, .T. ) ;
#2131=ORIENTED_EDGE ( 'NONE', *, *, #12002, .T. ) ;
#2134=EDGE_LOOP ( 'NONE', ( #8813, #10347 ) ) ;
#2135=CLOSED_SHELL ( 'NONE', ( #10986, #4360, #4734, #1977, #11427, #9285, #12252, #2793, #13511, #4146, #8949, #2966, #4475, #282, #1182, #2890, #9514, #7397, #9351, #9390, #1023, #7312, #701, #1959, #11279, #11167, #4130 ) ) ;
#2136=CARTESIAN_POINT ( 'NONE',  ( -0.05918829504999999908, 10.97290950744599947, 62.14999999999999858 ) ) ;
#2139=ORIENTED_EDGE ( 'NONE', *, *, #3841, .F. ) ;
#2140=CARTESIAN_POINT ( 'NONE',  ( -18.05918829504999934, 10.97290950744599947, 63.54999999999999716 ) ) ;
#2141=DIRECTION ( 'NONE',  ( -0.4528443260392611136, -0.8915896008669277339, 0.000000000000000000 ) ) ;
#2143=CYLINDRICAL_SURFACE ( 'NONE', #5999, 6.000000000000002665 ) ;
#2144=CIRCLE ( 'NONE', #1676, 16.75000000000000355 ) ;
#2147=ORIENTED_EDGE ( 'NONE', *, *, #2760, .F. ) ;
#2150=VECTOR ( 'NONE', #11865, 1000.000000000000227 ) ;
#2154=DIRECTION ( 'NONE',  ( 1.000000000000000000, 0.000000000000000000, 0.000000000000000000 ) ) ;
#2155=CARTESIAN_POINT ( 'NONE',  ( -19.45034526138887188, 30.31858837287976272, 53.29192511634208529 ) ) ;
#2156=CARTESIAN_POINT ( 'NONE',  ( -11.74835982676941981, -4.028726038184999858, 62.14999999999999858 ) ) ;
#2158=CARTESIAN_POINT ( 'NONE',  ( -21.16117192841894834, 4.865520741507539881, 61.25000000000000000 ) ) ;
#2159=CARTESIAN_POINT ( 'NONE',  ( -39.30918829504999934, 27.97290950744599769, 58.85000000000000142 ) ) ;
#2165=EDGE_CURVE ( 'NONE', #1164, #11479, #13593, .T. ) ;
#2166=EDGE_LOOP ( 'NONE', ( #3453, #7119, #2202, #7275 ) ) ;
#2167=DIRECTION ( 'NONE',  ( 0.4528443260392608360, 0.8915896008669278450, 0.000000000000000000 ) ) ;
#2171=VECTOR ( 'NONE', #1183, 1000.000000000000000 ) ;
#2173=DIRECTION ( 'NONE',  ( 0.000000000000000000, 0.000000000000000000, -1.000000000000000000 ) ) ;
#2177=CIRCLE ( 'NONE', #11750, 33.00000000000000000 ) ;
#2178=EDGE_CURVE ( 'NONE', #7807, #7753, #19, .T. ) ;
#2179=ORIENTED_EDGE ( 'NONE', *, *, #3469, .T. ) ;
#2180=EDGE_CURVE ( 'NONE', #10750, #586, #4056, .T. ) ;
#2181=CARTESIAN_POINT ( 'NONE',  ( -15.53293347889121989, 30.22252884722569988, 54.08287280684341880 ) ) ;
#2182=ORIENTED_EDGE ( 'NONE', *, *, #2264, .T. ) ;
#2185=DIRECTION ( 'NONE',  ( 0.000000000000000000, 0.000000000000000000, -1.000000000000000000 ) ) ;
#2186=DIRECTION ( 'NONE',  ( 1.000000000000000000, 0.000000000000000000, 0.000000000000000000 ) ) ;
#2187=VECTOR ( 'NONE', #955, 1000.000000000000000 ) ;
#2189=VERTEX_POINT ( 'NONE', #1022 ) ;
#2191=FACE_OUTER_BOUND ( 'NONE', #2483, .T. ) ;
#2193=DIRECTION ( 'NONE',  ( 0.000000000000000000, 0.000000000000000000, -1.000000000000000000 ) ) ;
#2194=EDGE_CURVE ( 'NONE', #2935, #703, #11852, .T. ) ;
#2196=CIRCLE ( 'NONE', #9998, 2.500000000000000000 ) ;
#2197=ORIENTED_EDGE ( 'NONE', *, *, #12092, .F. ) ;
#2198=EDGE_CURVE ( 'NONE', #2014, #4562, #3383, .T. ) ;
#2201=FACE_OUTER_BOUND ( 'NONE', #12238, .T. ) ;
#2202=ORIENTED_EDGE ( 'NONE', *, *, #718, .T. ) ;
#2204=ORIENTED_EDGE ( 'NONE', *, *, #6665, .F. ) ;
#2208=EDGE_LOOP ( 'NONE', ( #3202, #4187, #8745, #10570 ) ) ;
#2209=DIRECTION ( 'NONE',  ( 0.000000000000000000, 0.000000000000000000, -1.000000000000000000 ) ) ;
#2211=CIRCLE ( 'NONE', #10005, 4.750000000000000888 ) ;
#2213=DIRECTION ( 'NONE',  ( 0.000000000000000000, 0.000000000000000000, 1.000000000000000000 ) ) ;
#2214=CIRCLE ( 'NONE', #11556, 24.92993838181874722 ) ;
#2217=ADVANCED_FACE ( 'NONE', ( #7093 ), #4247, .T. ) ;
#2219=VECTOR ( 'NONE', #9243, 1000.000000000000000 ) ;
#2223=CARTESIAN_POINT ( 'NONE',  ( -35.05918829505000645, 27.97290950744599769, 58.85000000000000142 ) ) ;
#2226=EDGE_CURVE ( 'NONE', #6329, #9971, #2870, .T. ) ;
#2230=CARTESIAN_POINT ( 'NONE',  ( -26.45502162804999813, 10.97290950744599947, 60.04999999999999716 ) ) ;
#2231=DIRECTION ( 'NONE',  ( 0.000000000000000000, 0.000000000000000000, -1.000000000000000000 ) ) ;
#2232=DIRECTION ( 'NONE',  ( 0.000000000000000000, 0.000000000000000000, 1.000000000000000000 ) ) ;
#2233=CARTESIAN_POINT ( 'NONE',  ( -1.059188295049996231, 27.97290950744599769, 68.85549045786049760 ) ) ;
#2235=EDGE_CURVE ( 'NONE', #10451, #8158, #11439, .T. ) ;
#2238=ORIENTED_EDGE ( 'NONE', *, *, #8018, .F. ) ;
#2243=CARTESIAN_POINT ( 'NONE',  ( -39.30918829504999934, 27.97290950744599769, 64.85000000000000853 ) ) ;
#2244=EDGE_CURVE ( 'NONE', #912, #8943, #10521, .T. ) ;
#2246=AXIS2_PLACEMENT_3D ( 'NONE', #77, #11683, #994 ) ;
#2248=PLANE ( 'NONE',  #2969 ) ;
#2250=CARTESIAN_POINT ( 'NONE',  ( -18.05918829504999934, 10.97290950744599947, 60.60999999999999943 ) ) ;
#2251=CARTESIAN_POINT ( 'NONE',  ( -10.78334210919089919, 29.19143287883919768, 7.250000000000000000 ) ) ;
#2254=CIRCLE ( 'NONE', #7334, 2.500000000000000000 ) ;
#2256=CIRCLE ( 'NONE', #5566, 1.725000000000000755 ) ;
#2258=CARTESIAN_POINT ( 'NONE',  ( -15.80213232358579667, 30.25036691325134797, 53.83618312000469786 ) ) ;
#2260=ORIENTED_EDGE ( 'NONE', *, *, #11265, .F. ) ;
#2261=ORIENTED_EDGE ( 'NONE', *, *, #12459, .T. ) ;
#2262=DIRECTION ( 'NONE',  ( 0.000000000000000000, 0.000000000000000000, 1.000000000000000000 ) ) ;
#2264=EDGE_CURVE ( 'NONE', #12897, #9534, #6600, .T. ) ;
#2265=( LENGTH_UNIT ( ) NAMED_UNIT ( * ) SI_UNIT ( .MILLI., .METRE. ) );
#2268=CARTESIAN_POINT ( 'NONE',  ( -18.05918829504999934, 10.97290950744599947, 62.14999999999999858 ) ) ;
#2271=AXIS2_PLACEMENT_3D ( 'NONE', #2778, #4843, #1845 ) ;
#2272=AXIS2_PLACEMENT_3D ( 'NONE', #7060, #12387, #782 ) ;
#2274=EDGE_CURVE ( 'NONE', #4079, #1491, #4720, .T. ) ;
#2277=CIRCLE ( 'NONE', #7357, 0.9499999999999995115 ) ;
#2279=VERTEX_POINT ( 'NONE', #3476 ) ;
#2280=ORIENTED_EDGE ( 'NONE', *, *, #3168, .T. ) ;
#2282=DIRECTION ( 'NONE',  ( 0.000000000000000000, 0.000000000000000000, -1.000000000000000000 ) ) ;
#2283=ORIENTED_EDGE ( 'NONE', *, *, #8978, .F. ) ;
#2287=FACE_OUTER_BOUND ( 'NONE', #4614, .T. ) ;
#2288=EDGE_CURVE ( 'NONE', #10798, #2353, #1355, .T. ) ;
#2290=COLOUR_RGB ( '', 0.31764706, 0.68627451, 0.89019608) ;
#2293=CIRCLE ( 'NONE', #1600, 4.750000000000000888 ) ;
#2294=ORIENTED_EDGE ( 'NONE', *, *, #6998, .F. ) ;
#2296=VERTEX_POINT ( 'NONE', #10876 ) ;
#2297=CIRCLE ( 'NONE', #698, 4.250000000000000000 ) ;
#2299=EDGE_LOOP ( 'NONE', ( #666, #3811 ) ) ;
#2300=LINE ( 'NONE', #6535, #12959 ) ;
#2301=CARTESIAN_POINT ( 'NONE',  ( -20.84461927375554779, 30.19267137841694293, 54.36848034354279946 ) ) ;
#2302=LINE ( 'NONE', #11772, #1160 ) ;
#2303=LINE ( 'NONE', #11921, #9799 ) ;
#2305=CYLINDRICAL_SURFACE ( 'NONE', #5365, 8.299999999999998934 ) ;
#2313=ORIENTED_EDGE ( 'NONE', *, *, #9180, .F. ) ;
#2315=ORIENTED_EDGE ( 'NONE', *, *, #7940, .T. ) ;
#2316=ORIENTED_EDGE ( 'NONE', *, *, #1679, .F. ) ;
#2317=ORIENTED_EDGE ( 'NONE', *, *, #8020, .T. ) ;
#2318=ORIENTED_EDGE ( 'NONE', *, *, #13401, .T. ) ;
#2319=DIRECTION ( 'NONE',  ( 0.000000000000000000, 0.000000000000000000, 1.000000000000000000 ) ) ;
#2322=LINE ( 'NONE', #480, #13616 ) ;
#2323=SURFACE_STYLE_FILL_AREA ( #6349 ) ;
#2324=CARTESIAN_POINT ( 'NONE',  ( 0.000000000000000000, 0.000000000000000000, 17.25000000000000000 ) ) ;
#2326=EDGE_CURVE ( 'NONE', #1970, #9632, #4494, .T. ) ;
#2327=DIRECTION ( 'NONE',  ( 0.9496839325805418452, -0.3132098788326394545, 0.000000000000000000 ) ) ;
#2328=DIRECTION ( 'NONE',  ( 0.000000000000000000, 0.000000000000000000, -1.000000000000000000 ) ) ;
#2330=EDGE_CURVE ( 'NONE', #3796, #4496, #9836, .T. ) ;
#2331=CIRCLE ( 'NONE', #12781, 16.50000000000000000 ) ;
#2333=ORIENTED_EDGE ( 'NONE', *, *, #1546, .T. ) ;
#2334=CARTESIAN_POINT ( 'NONE',  ( -16.46704392475020384, 30.30564942409548834, 53.38979243784910267 ) ) ;
#2336=LINE ( 'NONE', #3365, #10855 ) ;
#2337=LINE ( 'NONE', #12992, #7804 ) ;
#2338=DIRECTION ( 'NONE',  ( 0.000000000000000000, 0.000000000000000000, 1.000000000000000000 ) ) ;
#2340=CARTESIAN_POINT ( 'NONE',  ( -18.05918829504999934, 19.05294282444599929, 63.34900083300000517 ) ) ;
#2343=EDGE_CURVE ( 'NONE', #8943, #1848, #244, .T. ) ;
#2344=EDGE_CURVE ( 'NONE', #5817, #3979, #7816, .T. ) ;
#2345=VERTEX_POINT ( 'NONE', #9624 ) ;
#2348=DIRECTION ( 'NONE',  ( -1.000000000000000000, 0.000000000000000000, 0.000000000000000000 ) ) ;
#2350=ORIENTED_EDGE ( 'NONE', *, *, #10332, .T. ) ;
#2352=DIRECTION ( 'NONE',  ( 1.000000000000000000, 0.000000000000000000, 0.000000000000000000 ) ) ;
#2353=VERTEX_POINT ( 'NONE', #46 ) ;
#2354=CARTESIAN_POINT ( 'NONE',  ( -26.45502162804999813, 10.97290950744599947, 60.04999999999999716 ) ) ;
#2355=DIRECTION ( 'NONE',  ( 0.000000000000000000, 0.000000000000000000, 1.000000000000000000 ) ) ;
#2359=ORIENTED_EDGE ( 'NONE', *, *, #6536, .T. ) ;
#2360=ORIENTED_EDGE ( 'NONE', *, *, #8140, .T. ) ;
#2361=EDGE_CURVE ( 'NONE', #322, #11675, #12888, .T. ) ;
#2364=DIRECTION ( 'NONE',  ( 0.000000000000000000, 0.000000000000000000, 1.000000000000000000 ) ) ;
#2366=EDGE_CURVE ( 'NONE', #12635, #12583, #2855, .T. ) ;
#2368=CARTESIAN_POINT ( 'NONE',  ( -18.05918829504999934, 10.97290950744599947, 118.8499999999999943 ) ) ;
#2370=AXIS2_PLACEMENT_3D ( 'NONE', #6985, #3658, #364 ) ;
#2371=CARTESIAN_POINT ( 'NONE',  ( -18.97831362643889364, 30.34240036357632775, 53.11745017557792892 ) ) ;
#2372=CARTESIAN_POINT ( 'NONE',  ( -18.05918829504999934, 10.97290950744599947, 27.09999999999999787 ) ) ;
#2373=ORIENTED_EDGE ( 'NONE', *, *, #4555, .F. ) ;
#2374=CARTESIAN_POINT ( 'NONE',  ( -18.05918829504999934, 3.815137874446000055, 61.70038048199999281 ) ) ;
#2376=DIRECTION ( 'NONE',  ( 1.000000000000000000, 0.000000000000000000, 0.000000000000000000 ) ) ;
#2378=ADVANCED_FACE ( 'NONE', ( #10738 ), #7484, .F. ) ;
#2381=ADVANCED_FACE ( 'NONE', ( #11854 ), #2305, .T. ) ;
#2382=EDGE_LOOP ( 'NONE', ( #7662, #6702 ) ) ;
#2384=VERTEX_POINT ( 'NONE', #10247 ) ;
#2388=DIRECTION ( 'NONE',  ( 0.000000000000000000, 0.000000000000000000, 1.000000000000000000 ) ) ;
#2390=DIRECTION ( 'NONE',  ( 1.000000000000000000, 0.000000000000000000, 0.000000000000000000 ) ) ;
#2391=FACE_OUTER_BOUND ( 'NONE', #164, .T. ) ;
#2392=DIRECTION ( 'NONE',  ( 1.000000000000000000, 0.000000000000000000, 0.000000000000000000 ) ) ;
#2393=EDGE_CURVE ( 'NONE', #467, #10600, #12519, .T. ) ;
#2394=CIRCLE ( 'NONE', #7463, 6.000000000000000888 ) ;
#2400=CARTESIAN_POINT ( 'NONE',  ( -17.52807689001588898, 30.35571874317117036, 53.02236195993357626 ) ) ;
#2401=VERTEX_POINT ( 'NONE', #13372 ) ;
#2403=CARTESIAN_POINT ( 'NONE',  ( -18.05918829504999934, 10.97290950744599947, 60.40999999999999659 ) ) ;
#2405=CARTESIAN_POINT ( 'NONE',  ( 0.09777679598749940137, 23.36596564213564875, 68.85549045786049760 ) ) ;
#2407=ORIENTED_EDGE ( 'NONE', *, *, #11274, .T. ) ;
#2408=LINE ( 'NONE', #1253, #3768 ) ;
#2411=FACE_OUTER_BOUND ( 'NONE', #6638, .T. ) ;
#2412=AXIS2_PLACEMENT_3D ( 'NONE', #2814, #6906, #13130 ) ;
#2413=CARTESIAN_POINT ( 'NONE',  ( -15.74360204493244986, 8.348398063716610196, 68.84999999999999432 ) ) ;
#2414=VERTEX_POINT ( 'NONE', #9047 ) ;
#2417=ORIENTED_EDGE ( 'NONE', *, *, #7104, .T. ) ;
#2420=EDGE_LOOP ( 'NONE', ( #7600, #94, #3579, #494 ) ) ;
#2422=CARTESIAN_POINT ( 'NONE',  ( -18.05918829504999934, 28.64232754551664684, 57.35000000000000142 ) ) ;
#2424=EDGE_CURVE ( 'NONE', #6052, #13581, #2293, .T. ) ;
#2427=CARTESIAN_POINT ( 'NONE',  ( -34.65718996104999405, 19.27191034044602347, 63.13003331700004850 ) ) ;
#2428=CARTESIAN_POINT ( 'NONE',  ( -21.79515398487389888, 3.617295300293844829, 63.64999999999999858 ) ) ;
#2429=CARTESIAN_POINT ( 'NONE',  ( -18.05918829504999934, 10.97290950744599947, 5.250000000000000000 ) ) ;
#2430=AXIS2_PLACEMENT_3D ( 'NONE', #4097, #9526, #8473 ) ;
#2431=AXIS2_PLACEMENT_3D ( 'NONE', #5267, #3205, #2154 ) ;
#2432=VERTEX_POINT ( 'NONE', #3817 ) ;
#2433=ORIENTED_EDGE ( 'NONE', *, *, #3714, .T. ) ;
#2434=LINE ( 'NONE', #6741, #13524 ) ;
#2437=VECTOR ( 'NONE', #11624, 1000.000000000000000 ) ;
#2441=CARTESIAN_POINT ( 'NONE',  ( -20.79267224994196894, 30.19895062614576986, 60.39398676968448854 ) ) ;
#2443=VERTEX_POINT ( 'NONE', #3745 ) ;
#2445=DIRECTION ( 'NONE',  ( 0.000000000000000000, 0.000000000000000000, -1.000000000000000000 ) ) ;
#2446=DIRECTION ( 'NONE',  ( 0.000000000000000000, 0.000000000000000000, -1.000000000000000000 ) ) ;
#2447=DIRECTION ( 'NONE',  ( 0.000000000000000000, 0.000000000000000000, -1.000000000000000000 ) ) ;
#2450=AXIS2_PLACEMENT_3D ( 'NONE', #9885, #8816, #3520 ) ;
#2451=VECTOR ( 'NONE', #3917, 1000.000000000000114 ) ;
#2452=VECTOR ( 'NONE', #4836, 1000.000000000000000 ) ;
#2453=EDGE_LOOP ( 'NONE', ( #5662, #11085, #5895, #12385 ) ) ;
#2455=FACE_BOUND ( 'NONE', #2751, .T. ) ;
#2458=FACE_OUTER_BOUND ( 'NONE', #9489, .T. ) ;
#2459=CARTESIAN_POINT ( 'NONE',  ( -18.05918829504999934, 10.00028003023991907, 62.14999999999999858 ) ) ;
#2460=FACE_OUTER_BOUND ( 'NONE', #1715, .T. ) ;
#2464=DIRECTION ( 'NONE',  ( 0.000000000000000000, 0.000000000000000000, 1.000000000000000000 ) ) ;
#2469=ORIENTED_EDGE ( 'NONE', *, *, #11241, .F. ) ;
#2470=DIRECTION ( 'NONE',  ( 0.000000000000000000, 0.000000000000000000, 1.000000000000000000 ) ) ;
#2472=ORIENTED_EDGE ( 'NONE', *, *, #7416, .T. ) ;
#2473=DIRECTION ( 'NONE',  ( 0.000000000000000000, 0.000000000000000000, 1.000000000000000000 ) ) ;
#2479=VECTOR ( 'NONE', #8806, 1000.000000000000000 ) ;
#2482=EDGE_CURVE ( 'NONE', #7243, #4278, #12969, .T. ) ;
#2483=EDGE_LOOP ( 'NONE', ( #2139, #1836, #2147, #5005 ) ) ;
#2485=ORIENTED_EDGE ( 'NONE', *, *, #70, .F. ) ;
#2491=VECTOR ( 'NONE', #5037, 1000.000000000000114 ) ;
#2492=FACE_OUTER_BOUND ( 'NONE', #432, .T. ) ;
#2493=DIRECTION ( 'NONE',  ( 1.000000000000000000, 0.000000000000000000, 0.000000000000000000 ) ) ;
#2496=CYLINDRICAL_SURFACE ( 'NONE', #5853, 3.450000000000001510 ) ;
#2498=EDGE_CURVE ( 'NONE', #1128, #11621, #12532, .T. ) ;
#2500=AXIS2_PLACEMENT_3D ( 'NONE', #7654, #6553, #8639 ) ;
#2502=EDGE_CURVE ( 'NONE', #9534, #506, #33, .T. ) ;
#2505=DIRECTION ( 'NONE',  ( -0.7071067811865489050, -8.659560562354948882E-17, -0.7071067811865460184 ) ) ;
#2506=CARTESIAN_POINT ( 'NONE',  ( -20.60703947854099027, 30.22015921464618771, 60.59533421581512158 ) ) ;
#2507=AXIS2_PLACEMENT_3D ( 'NONE', #3650, #1326, #9997 ) ;
#2509=DIRECTION ( 'NONE',  ( -1.000000000000000000, 0.000000000000000000, 0.000000000000000000 ) ) ;
#2514=DIRECTION ( 'NONE',  ( 0.000000000000000000, 0.000000000000000000, -1.000000000000000000 ) ) ;
#2518=ORIENTED_EDGE ( 'NONE', *, *, #6001, .T. ) ;
#2519=EDGE_CURVE ( 'NONE', #11621, #1128, #9631, .T. ) ;
#2524=ORIENTED_EDGE ( 'NONE', *, *, #2165, .T. ) ;
#2525=ORIENTED_EDGE ( 'NONE', *, *, #7957, .T. ) ;
#2528=DIRECTION ( 'NONE',  ( 0.000000000000000000, 0.000000000000000000, 1.000000000000000000 ) ) ;
#2533=FACE_OUTER_BOUND ( 'NONE', #3068, .T. ) ;
#2534=DIRECTION ( 'NONE',  ( 0.000000000000000000, 0.000000000000000000, -1.000000000000000000 ) ) ;
#2535=( GEOMETRIC_REPRESENTATION_CONTEXT ( 3 ) GLOBAL_UNCERTAINTY_ASSIGNED_CONTEXT ( ( #10197 ) ) GLOBAL_UNIT_ASSIGNED_CONTEXT ( ( #3271, #4520, #3618 ) ) REPRESENTATION_CONTEXT ( 'NONE', 'WORKASPACE' ) );
#2536=CARTESIAN_POINT ( 'NONE',  ( -18.05918829504999934, 10.97290950744599947, 57.54999999999999716 ) ) ;
#2539=( GEOMETRIC_REPRESENTATION_CONTEXT ( 3 ) GLOBAL_UNCERTAINTY_ASSIGNED_CONTEXT ( ( #3231 ) ) GLOBAL_UNIT_ASSIGNED_CONTEXT ( ( #8984, #5678, #3679 ) ) REPRESENTATION_CONTEXT ( 'NONE', 'WORKASPACE' ) );
#2542=EDGE_CURVE ( 'NONE', #7101, #12858, #13242, .T. ) ;
#2543=ADVANCED_FACE ( 'NONE', ( #5682, #11022 ), #9961, .T. ) ;
#2546=CARTESIAN_POINT ( 'NONE',  ( -18.05918829504999934, 10.97290950744599947, 68.84999999999999432 ) ) ;
#2549=CYLINDRICAL_SURFACE ( 'NONE', #1774, 16.95000000000000284 ) ;
#2550=CARTESIAN_POINT ( 'NONE',  ( -18.05918829504999934, 2.673908674445999889, 63.13003331699999876 ) ) ;
#2552=AXIS2_PLACEMENT_3D ( 'NONE', #3355, #6488, #62 ) ;
#2554=CARTESIAN_POINT ( 'NONE',  ( -21.79515398487389888, 3.617295300293844829, 60.04999999999999716 ) ) ;
#2555=VERTEX_POINT ( 'NONE', #2080 ) ;
#2557=ORIENTED_EDGE ( 'NONE', *, *, #7029, .F. ) ;
#2558=ORIENTED_EDGE ( 'NONE', *, *, #2519, .T. ) ;
#2560=EDGE_LOOP ( 'NONE', ( #6168, #873, #5066, #7682 ) ) ;
#2561=CARTESIAN_POINT ( 'NONE',  ( -32.37473156004999453, 3.815137874445994282, 61.70038048200006386 ) ) ;
#2564=DIRECTION ( 'NONE',  ( -0.000000000000000000, -0.000000000000000000, -1.000000000000000000 ) ) ;
#2566=DIRECTION ( 'NONE',  ( 0.000000000000000000, 0.000000000000000000, 1.000000000000000000 ) ) ;
#2567=DIRECTION ( 'NONE',  ( 0.000000000000000000, 0.000000000000000000, -1.000000000000000000 ) ) ;
#2568=ORIENTED_EDGE ( 'NONE', *, *, #6412, .T. ) ;
#2569=ORIENTED_EDGE ( 'NONE', *, *, #4407, .T. ) ;
#2570=ORIENTED_EDGE ( 'NONE', *, *, #6345, .F. ) ;
#2572=CARTESIAN_POINT ( 'NONE',  ( 3.190811704950004657, 27.97290950744599769, 64.85000000000000853 ) ) ;
#2573=VERTEX_POINT ( 'NONE', #10581 ) ;
#2575=CARTESIAN_POINT ( 'NONE',  ( -21.61797324970345002, 30.08605482698171230, 55.74785149929289219 ) ) ;
#2577=CARTESIAN_POINT ( 'NONE',  ( -18.05918829504999934, 10.97290950744599947, 61.10999999999999943 ) ) ;
#2586=AXIS2_PLACEMENT_3D ( 'NONE', #9879, #302, #11745 ) ;
#2587=DIRECTION ( 'NONE',  ( 0.2878798879079283446, -0.9576665234506834823, 0.000000000000000000 ) ) ;
#2588=DIRECTION ( 'NONE',  ( 0.000000000000000000, 0.000000000000000000, -1.000000000000000000 ) ) ;
#2590=CYLINDRICAL_SURFACE ( 'NONE', #11536, 0.9499999999999995115 ) ;
#2592=DIRECTION ( 'NONE',  ( 1.000000000000000000, 0.000000000000000000, 0.000000000000000000 ) ) ;
#2593=ORIENTED_EDGE ( 'NONE', *, *, #9946, .F. ) ;
#2595=CARTESIAN_POINT ( 'NONE',  ( -18.05918829504999934, 10.97290950744599947, 62.14999999999999858 ) ) ;
#2597=CARTESIAN_POINT ( 'NONE',  ( 3.690811704950009986, -6.027090492554000534, 64.85000000000000853 ) ) ;
#2598=EDGE_CURVE ( 'NONE', #9237, #5689, #9402, .T. ) ;
#2599=DIRECTION ( 'NONE',  ( 0.000000000000000000, 0.000000000000000000, -1.000000000000000000 ) ) ;
#2605=CYLINDRICAL_SURFACE ( 'NONE', #11056, 1.725000000000000755 ) ;
#2606=ORIENTED_EDGE ( 'NONE', *, *, #7448, .F. ) ;
#2607=CARTESIAN_POINT ( 'NONE',  ( -35.05918829505000645, -6.027090492554000534, 5.250000000000000000 ) ) ;
#2609=DIRECTION ( 'NONE',  ( -0.7071067811865500152, 8.659560562354959975E-17, 0.7071067811865450192 ) ) ;
#2611=CARTESIAN_POINT ( 'NONE',  ( -18.05918829504999934, 10.97290950744599947, 61.10999999999999943 ) ) ;
#2612=CARTESIAN_POINT ( 'NONE',  ( -18.05918829504999934, 10.97290950744599947, 17.25000000000000000 ) ) ;
#2614=EDGE_CURVE ( 'NONE', #3389, #10398, #11193, .T. ) ;
#2616=EDGE_LOOP ( 'NONE', ( #3190, #7711, #8717, #7553, #4509 ) ) ;
#2620=CARTESIAN_POINT ( 'NONE',  ( -17.14006296349294445, 30.34240036356348824, 61.58254982436883296 ) ) ;
#2623=ORIENTED_EDGE ( 'NONE', *, *, #2288, .F. ) ;
#2624=ORIENTED_EDGE ( 'NONE', *, *, #8194, .F. ) ;
#2626=DIRECTION ( 'NONE',  ( 0.000000000000000000, 0.000000000000000000, -1.000000000000000000 ) ) ;
#2630=DIRECTION ( 'NONE',  ( 1.000000000000000000, 0.000000000000000000, 0.000000000000000000 ) ) ;
#2637=( GEOMETRIC_REPRESENTATION_CONTEXT ( 3 ) GLOBAL_UNCERTAINTY_ASSIGNED_CONTEXT ( ( #8094 ) ) GLOBAL_UNIT_ASSIGNED_CONTEXT ( ( #538, #4800, #5634 ) ) REPRESENTATION_CONTEXT ( 'NONE', 'WORKASPACE' ) );
#2638=ORIENTED_EDGE ( 'NONE', *, *, #6634, .F. ) ;
#2639=DIRECTION ( 'NONE',  ( 0.000000000000000000, 0.000000000000000000, -1.000000000000000000 ) ) ;
#2641=CARTESIAN_POINT ( 'NONE',  ( -21.45399636639216467, 30.11090903168091870, 59.35894009006398875 ) ) ;
#2642=ORIENTED_EDGE ( 'NONE', *, *, #1410, .T. ) ;
#2643=FILL_AREA_STYLE ('',( #10038 ) ) ;
#2644=DIRECTION ( 'NONE',  ( 0.000000000000000000, 0.000000000000000000, -1.000000000000000000 ) ) ;
#2648=DIRECTION ( 'NONE',  ( 0.000000000000000000, 0.000000000000000000, -1.000000000000000000 ) ) ;
#2649=EDGE_LOOP ( 'NONE', ( #4958, #10882, #10234, #7832 ) ) ;
#2650=ADVANCED_FACE ( 'NONE', ( #6098 ), #10371, .F. ) ;
#2651=AXIS2_PLACEMENT_3D ( 'NONE', #11554, #6242, #9600 ) ;
#2652=CIRCLE ( 'NONE', #3301, 6.449999999999997513 ) ;
#2657=DIRECTION ( 'NONE',  ( 1.000000000000000000, 0.000000000000000000, 0.000000000000000000 ) ) ;
#2658=LINE ( 'NONE', #1799, #224 ) ;
#2659=FACE_OUTER_BOUND ( 'NONE', #11248, .T. ) ;
#2660=DIRECTION ( 'NONE',  ( -0.4528443260392610026, -0.8915896008669278450, 0.000000000000000000 ) ) ;
#2661=DIRECTION ( 'NONE',  ( 0.000000000000000000, 0.000000000000000000, -1.000000000000000000 ) ) ;
#2664=FACE_OUTER_BOUND ( 'NONE', #3235, .T. ) ;
#2665=DIRECTION ( 'NONE',  ( 0.6615960714621567096, -0.7498604124941127269, 0.000000000000000000 ) ) ;
#2668=CIRCLE ( 'NONE', #7292, 24.92993838181874722 ) ;
#2670=AXIS2_PLACEMENT_3D ( 'NONE', #2324, #4467, #10611 ) ;
#2673=ADVANCED_FACE ( 'NONE', ( #946 ), #8277, .T. ) ;
#2674=CARTESIAN_POINT ( 'NONE',  ( -24.37001676333060018, -4.028726038184999858, 62.14999999999999858 ) ) ;
#2675=VECTOR ( 'NONE', #11102, 1000.000000000000000 ) ;
#2678=CARTESIAN_POINT ( 'NONE',  ( -16.55918829504999579, 27.19822998463810393, 57.14449823292466135 ) ) ;
#2682=DIRECTION ( 'NONE',  ( 0.000000000000000000, 0.000000000000000000, 1.000000000000000000 ) ) ;
#2683=DIRECTION ( 'NONE',  ( 0.000000000000000000, 0.000000000000000000, -1.000000000000000000 ) ) ;
#2684=DIRECTION ( 'NONE',  ( 0.000000000000000000, 0.000000000000000000, -1.000000000000000000 ) ) ;
#2685=CARTESIAN_POINT ( 'NONE',  ( -18.05918829504999934, 10.97290950744599947, 62.14999999999999858 ) ) ;
#2688=ORIENTED_EDGE ( 'NONE', *, *, #13210, .T. ) ;
#2693=CARTESIAN_POINT ( 'NONE',  ( -16.76337124042152382, 30.32416700402973575, 61.44969122351110968 ) ) ;
#2696=DIRECTION ( 'NONE',  ( 0.6615960714621565986, -0.7498604124941126159, 0.000000000000000000 ) ) ;
#2702=ORIENTED_EDGE ( 'NONE', *, *, #7155, .F. ) ;
#2704=AXIS2_PLACEMENT_3D ( 'NONE', #563, #9873, #4822 ) ;
#2705=VECTOR ( 'NONE', #13244, 1000.000000000000000 ) ;
#2706=DIRECTION ( 'NONE',  ( -1.000000000000000000, 0.000000000000000000, 0.000000000000000000 ) ) ;
#2707=ORIENTED_EDGE ( 'NONE', *, *, #4060, .T. ) ;
#2709=ORIENTED_EDGE ( 'NONE', *, *, #7319, .T. ) ;
#2710=DIRECTION ( 'NONE',  ( 0.000000000000000000, 0.000000000000000000, 1.000000000000000000 ) ) ;
#2711=VERTEX_POINT ( 'NONE', #7545 ) ;
#2713=ORIENTED_EDGE ( 'NONE', *, *, #6399, .F. ) ;
#2714=EDGE_CURVE ( 'NONE', #9883, #6370, #9185, .T. ) ;
#2716=CARTESIAN_POINT ( 'NONE',  ( -20.96223510382219857, 30.17819129720234628, 60.18295065293622059 ) ) ;
#2720=CARTESIAN_POINT ( 'NONE',  ( -25.86749127492454647, -8.860076549334127805, 5.250000000000000000 ) ) ;
#2721=CIRCLE ( 'NONE', #4052, 4.750000000000000888 ) ;
#2722=VECTOR ( 'NONE', #2661, 1000.000000000000000 ) ;
#2725=VECTOR ( 'NONE', #6013, 1000.000000000000000 ) ;
#2726=AXIS2_PLACEMENT_3D ( 'NONE', #2960, #13539, #6975 ) ;
#2727=CARTESIAN_POINT ( 'NONE',  ( -38.38077571930826082, -0.4981161769137699147, 17.25000000000000000 ) ) ;
#2728=CARTESIAN_POINT ( 'NONE',  ( -18.05918829504999934, 10.97290950744599947, 63.54999999999999716 ) ) ;
#2729=AXIS2_PLACEMENT_3D ( 'NONE', #10537, #6340, #964 ) ;
#2730=VERTEX_POINT ( 'NONE', #1274 ) ;
#2731=CARTESIAN_POINT ( 'NONE',  ( -20.77625425128555392, 5.623371902244430842, 60.04999999999999716 ) ) ;
#2732=EDGE_CURVE ( 'NONE', #10905, #3167, #13196, .T. ) ;
#2735=CARTESIAN_POINT ( 'NONE',  ( -35.05918829505000645, 27.97290950744599769, 64.85000000000000853 ) ) ;
#2736=CARTESIAN_POINT ( 'NONE',  ( -21.78591716150126700, 14.35275298274230771, 68.85000000000003695 ) ) ;
#2737=LINE ( 'NONE', #4745, #8002 ) ;
#2740=DIRECTION ( 'NONE',  ( -1.000000000000000000, 0.000000000000000000, 0.000000000000000000 ) ) ;
#2742=ADVANCED_FACE ( 'NONE', ( #9816 ), #1070, .T. ) ;
#2743=VECTOR ( 'NONE', #12842, 1000.000000000000114 ) ;
#2744=AXIS2_PLACEMENT_3D ( 'NONE', #5604, #311, #4501 ) ;
#2745=AXIS2_PLACEMENT_3D ( 'NONE', #1925, #10438, #7075 ) ;
#2746=VERTEX_POINT ( 'NONE', #4304 ) ;
#2748=VERTEX_POINT ( 'NONE', #4232 ) ;
#2749=DIRECTION ( 'NONE',  ( -1.000000000000000000, 0.000000000000000000, 0.000000000000000000 ) ) ;
#2750=ORIENTED_EDGE ( 'NONE', *, *, #3059, .F. ) ;
#2751=EDGE_LOOP ( 'NONE', ( #1166, #11731 ) ) ;
#2753=FACE_OUTER_BOUND ( 'NONE', #774, .T. ) ;
#2754=CIRCLE ( 'NONE', #4513, 2.500000000000000000 ) ;
#2755=CARTESIAN_POINT ( 'NONE',  ( -18.05918829504999934, 10.97290950744599947, 60.65000000000000568 ) ) ;
#2758=DIRECTION ( 'NONE',  ( 0.000000000000000000, 0.000000000000000000, -1.000000000000000000 ) ) ;
#2759=DIRECTION ( 'NONE',  ( 0.000000000000000000, 0.000000000000000000, -1.000000000000000000 ) ) ;
#2760=EDGE_CURVE ( 'NONE', #5663, #5817, #2066, .T. ) ;
#2765=ORIENTED_EDGE ( 'NONE', *, *, #11415, .T. ) ;
#2766=EDGE_LOOP ( 'NONE', ( #9909, #7352, #13693, #5713, #2359, #9445, #4998, #6703, #10631, #832, #13574, #7415, #7002, #6417, #2882 ) ) ;
#2768=ORIENTED_EDGE ( 'NONE', *, *, #469, .T. ) ;
#2770=DIRECTION ( 'NONE',  ( 0.000000000000000000, -1.000000000000000000, 0.000000000000000000 ) ) ;
#2772=ORIENTED_EDGE ( 'NONE', *, *, #10363, .F. ) ;
#2774=VECTOR ( 'NONE', #1066, 1000.000000000000000 ) ;
#2775=DIRECTION ( 'NONE',  ( 1.000000000000000000, 0.000000000000000000, 0.000000000000000000 ) ) ;
#2776=DIRECTION ( 'NONE',  ( 1.000000000000000000, 0.000000000000000000, 0.000000000000000000 ) ) ;
#2778=CARTESIAN_POINT ( 'NONE',  ( -18.05918829504999934, 10.97290950744599947, 64.54999999999999716 ) ) ;
#2780=CIRCLE ( 'NONE', #9454, 4.750000000000000000 ) ;
#2781=VERTEX_POINT ( 'NONE', #5326 ) ;
#2782=ORIENTED_EDGE ( 'NONE', *, *, #1866, .T. ) ;
#2783=ORIENTED_EDGE ( 'NONE', *, *, #2795, .F. ) ;
#2784=EDGE_LOOP ( 'NONE', ( #4148, #7186, #11195, #9958, #2179 ) ) ;
#2787=DIRECTION ( 'NONE',  ( 0.000000000000000000, 0.000000000000000000, 1.000000000000000000 ) ) ;
#2788=CARTESIAN_POINT ( 'NONE',  ( -35.05918829505000645, -6.027090492554000534, 64.35000000000000853 ) ) ;
#2789=DIRECTION ( 'NONE',  ( 0.6615960714621568206, -0.7498604124941125049, 0.000000000000000000 ) ) ;
#2790=FACE_OUTER_BOUND ( 'NONE', #6814, .T. ) ;
#2791=ORIENTED_EDGE ( 'NONE', *, *, #4555, .T. ) ;
#2793=ADVANCED_FACE ( 'NONE', ( #8686 ), #11832, .T. ) ;
#2794=ADVANCED_FACE ( 'NONE', ( #6654 ), #7686, .F. ) ;
#2795=EDGE_CURVE ( 'NONE', #10214, #13286, #12082, .T. ) ;
#2796=CARTESIAN_POINT ( 'NONE',  ( -24.35918829505000005, 10.97290950744599947, 63.02000000000000313 ) ) ;
#2798=EDGE_LOOP ( 'NONE', ( #8036, #5301, #3189, #9082 ) ) ;
#2799=DIRECTION ( 'NONE',  ( -1.000000000000000000, 0.000000000000000000, 0.000000000000000000 ) ) ;
#2801=CARTESIAN_POINT ( 'NONE',  ( -30.32854245105399826, 27.54455229823479812, 68.85549045786049760 ) ) ;
#2804=DIRECTION ( 'NONE',  ( 0.000000000000000000, 0.000000000000000000, 1.000000000000000000 ) ) ;
#2806=FACE_OUTER_BOUND ( 'NONE', #2117, .T. ) ;
#2810=ORIENTED_EDGE ( 'NONE', *, *, #10201, .T. ) ;
#2811=LINE ( 'NONE', #897, #568 ) ;
#2812=CLOSED_SHELL ( 'NONE', ( #13467, #5366, #833, #3183, #11924, #11985, #1267, #11129, #12404, #9536, #3247, #9036, #2842, #12521, #10500, #11684, #8483, #10388, #3757, #8654, #2922, #12950, #8702, #5981, #5775, #3924, #6119, #297, #2886, #6063, #3501, #1681, #3918 ) ) ;
#2813=EDGE_LOOP ( 'NONE', ( #2313, #4007, #10116, #12536 ) ) ;
#2814=CARTESIAN_POINT ( 'NONE',  ( -35.05918829505000645, -6.027090492554000534, 68.85549045786049760 ) ) ;
#2816=EDGE_CURVE ( 'NONE', #8976, #10798, #4504, .T. ) ;
#2819=VECTOR ( 'NONE', #10921, 1000.000000000000000 ) ;
#2820=CARTESIAN_POINT ( 'NONE',  ( -18.05918829504999223, 2.660265422445993622, 63.26601075299999621 ) ) ;
#2821=CARTESIAN_POINT ( 'NONE',  ( -18.05918829504999934, 10.97290950744599947, 61.65955166399999854 ) ) ;
#2822=DIRECTION ( 'NONE',  ( 0.000000000000000000, 0.000000000000000000, 1.000000000000000000 ) ) ;
#2823=EDGE_CURVE ( 'NONE', #2711, #13343, #5330, .T. ) ;
#2824=ORIENTED_EDGE ( 'NONE', *, *, #8285, .T. ) ;
#2825=CIRCLE ( 'NONE', #5912, 17.00000000000000000 ) ;
#2826=VERTEX_POINT ( 'NONE', #2428 ) ;
#2827=CARTESIAN_POINT ( 'NONE',  ( -14.81288417521985856, 30.13232420324952443, 55.04779169721881971 ) ) ;
#2829=EDGE_CURVE ( 'NONE', #1279, #7735, #1559, .T. ) ;
#2830=FACE_OUTER_BOUND ( 'NONE', #26, .T. ) ;
#2831=DIRECTION ( 'NONE',  ( 0.000000000000000000, 0.000000000000000000, 1.000000000000000000 ) ) ;
#2832=EDGE_LOOP ( 'NONE', ( #10672, #4684, #5805, #8541 ) ) ;
#2833=EDGE_LOOP ( 'NONE', ( #5875, #6796, #5453, #10803, #2104, #8113 ) ) ;
#2834=DIRECTION ( 'NONE',  ( 1.000000000000000000, 0.000000000000000000, 0.000000000000000000 ) ) ;
#2839=CARTESIAN_POINT ( 'NONE',  ( -22.71804201037815218, -4.525318844826149878, 63.45000000000000284 ) ) ;
#2842=ADVANCED_FACE ( 'NONE', ( #2287 ), #2143, .F. ) ;
#2843=ADVANCED_FACE ( 'NONE', ( #92 ), #7113, .F. ) ;
#2846=AXIS2_PLACEMENT_3D ( 'NONE', #3, #3292, #3439 ) ;
#2847=ADVANCED_FACE ( 'NONE', ( #3670 ), #10021, .F. ) ;
#2850=CARTESIAN_POINT ( 'NONE',  ( -20.28307750662727571, 30.25357667928725647, 60.89116620645845046 ) ) ;
#2855=( BOUNDED_CURVE ( )  B_SPLINE_CURVE ( 3, ( #10810, #4584, #7427, #6470 ),
 .UNSPECIFIED., .F., .F. ) 
 B_SPLINE_CURVE_WITH_KNOTS ( ( 4, 4 ),
 ( 0.04873315200000220143, 0.9512668486397960477 ),
 .UNSPECIFIED. ) 
 CURVE ( )  GEOMETRIC_REPRESENTATION_ITEM ( )  RATIONAL_B_SPLINE_CURVE ( ( 0.9230982619916300314, 0.4726811438562560364, 0.4726811441755530141, 0.9230982629495190217 ) ) 
 REPRESENTATION_ITEM ( '' )  );
#2857=ORIENTED_EDGE ( 'NONE', *, *, #2393, .F. ) ;
#2859=CARTESIAN_POINT ( 'NONE',  ( -25.32001676333059947, -4.028726038184999858, 62.14999999999999858 ) ) ;
#2862=DIRECTION ( 'NONE',  ( 0.4528443260392608916, 0.8915896008669279560, 0.000000000000000000 ) ) ;
#2863=DIRECTION ( 'NONE',  ( -0.4528443260392611136, -0.8915896008669277339, 0.000000000000000000 ) ) ;
#2867=CARTESIAN_POINT ( 'NONE',  ( -21.36716865236079954, 14.72221156991656166, 68.84999999999999432 ) ) ;
#2870=LINE ( 'NONE', #11371, #9408 ) ;
#2871=FACE_OUTER_BOUND ( 'NONE', #4641, .T. ) ;
#2872=AXIS2_PLACEMENT_3D ( 'NONE', #4523, #12400, #11424 ) ;
#2873=AXIS2_PLACEMENT_3D ( 'NONE', #12688, #10871, #1152 ) ;
#2880=AXIS2_PLACEMENT_3D ( 'NONE', #6978, #7685, #4503 ) ;
#2882=ORIENTED_EDGE ( 'NONE', *, *, #8783, .T. ) ;
#2883=CIRCLE ( 'NONE', #12880, 6.000000000000002665 ) ;
#2884=CONICAL_SURFACE ( 'NONE', #8882, 4.250000000000000000, 0.7853981633974524978 ) ;
#2885=CARTESIAN_POINT ( 'NONE',  ( -24.65502162805000097, 10.97290950744599947, 60.40999999999999659 ) ) ;
#2886=ADVANCED_FACE ( 'NONE', ( #3604 ), #1562, .F. ) ;
#2887=AXIS2_PLACEMENT_3D ( 'NONE', #7900, #13285, #5523 ) ;
#2890=ADVANCED_FACE ( 'NONE', ( #6793 ), #8897, .T. ) ;
#2894=VECTOR ( 'NONE', #9046, 1000.000000000000000 ) ;
#2896=AXIS2_PLACEMENT_3D ( 'NONE', #5772, #1451, #3762 ) ;
#2897=EDGE_LOOP ( 'NONE', ( #9668, #4967, #1209, #7175 ) ) ;
#2898=CARTESIAN_POINT ( 'NONE',  ( -14.57973916105114753, 30.09823897628803024, 59.16325671210135795 ) ) ;
#2900=VERTEX_POINT ( 'NONE', #4781 ) ;
#2903=DIRECTION ( 'NONE',  ( 0.000000000000000000, 0.000000000000000000, -1.000000000000000000 ) ) ;
#2905=LINE ( 'NONE', #8255, #2452 ) ;
#2906=EDGE_CURVE ( 'NONE', #3674, #2748, #8459, .T. ) ;
#2909=CYLINDRICAL_SURFACE ( 'NONE', #8330, 6.449999999999997513 ) ;
#2910=EDGE_CURVE ( 'NONE', #7294, #10905, #4842, .T. ) ;
#2911=DIRECTION ( 'NONE',  ( 0.000000000000000000, 0.000000000000000000, -1.000000000000000000 ) ) ;
#2913=CARTESIAN_POINT ( 'NONE',  ( -1.059188295049996231, 27.97290950744599769, 17.25000000000000000 ) ) ;
#2914=EDGE_CURVE ( 'NONE', #936, #8353, #11637, .T. ) ;
#2917=CIRCLE ( 'NONE', #3575, 4.250000000000003553 ) ;
#2921=DIRECTION ( 'NONE',  ( -0.4528443260392609471, -0.8915896008669277339, 0.000000000000000000 ) ) ;
#2922=ADVANCED_FACE ( 'NONE', ( #8821 ), #443, .T. ) ;
#2923=CARTESIAN_POINT ( 'NONE',  ( -20.29752877034432146, 30.25218297742089035, 60.87931115570677321 ) ) ;
#2924=DIRECTION ( 'NONE',  ( -1.000000000000000000, 0.000000000000000000, 0.000000000000000000 ) ) ;
#2925=CARTESIAN_POINT ( 'NONE',  ( -22.64501676333060232, -4.028726038184999858, 63.45000000000000284 ) ) ;
#2930=EDGE_CURVE ( 'NONE', #1821, #12100, #13082, .T. ) ;
#2931=AXIS2_PLACEMENT_3D ( 'NONE', #13507, #4029, #7010 ) ;
#2932=ORIENTED_EDGE ( 'NONE', *, *, #10775, .F. ) ;
#2933=DIRECTION ( 'NONE',  ( 0.6615960714621564875, -0.7498604124941129490, 0.000000000000000000 ) ) ;
#2935=VERTEX_POINT ( 'NONE', #1351 ) ;
#2936=DIRECTION ( 'NONE',  ( 0.000000000000000000, 0.000000000000000000, -1.000000000000000000 ) ) ;
#2937=CARTESIAN_POINT ( 'NONE',  ( -35.05918829505000645, 27.97290950744599769, 7.250000000000000000 ) ) ;
#2939=AXIS2_PLACEMENT_3D ( 'NONE', #9303, #7250, #9507 ) ;
#2941=LINE ( 'NONE', #4875, #10546 ) ;
#2946=DIRECTION ( 'NONE',  ( 0.000000000000000000, 0.000000000000000000, -1.000000000000000000 ) ) ;
#2947=DIRECTION ( 'NONE',  ( 1.000000000000000000, 0.000000000000000000, 0.000000000000000000 ) ) ;
#2949=AXIS2_PLACEMENT_3D ( 'NONE', #1624, #8770, #3406 ) ;
#2950=AXIS2_PLACEMENT_3D ( 'NONE', #9856, #9918, #2390 ) ;
#2960=CARTESIAN_POINT ( 'NONE',  ( -18.05918829504999934, 10.97290950744599947, 6.250000000000000000 ) ) ;
#2961=DIRECTION ( 'NONE',  ( 1.000000000000000000, 0.000000000000000000, 0.000000000000000000 ) ) ;
#2963=FACE_OUTER_BOUND ( 'NONE', #9811, .T. ) ;
#2966=ADVANCED_FACE ( 'NONE', ( #5606, #9890 ), #4636, .T. ) ;
#2967=EDGE_LOOP ( 'NONE', ( #12494, #12349 ) ) ;
#2968=EDGE_CURVE ( 'NONE', #8660, #6154, #203, .T. ) ;
#2969=AXIS2_PLACEMENT_3D ( 'NONE', #9702, #2173, #11667 ) ;
#2970=CARTESIAN_POINT ( 'NONE',  ( -15.42197072176424122, 30.21012672847304614, 60.50206344250329238 ) ) ;
#2971=EDGE_CURVE ( 'NONE', #6126, #10507, #4716, .T. ) ;
#2973=LINE ( 'NONE', #6140, #5709 ) ;
#2975=CARTESIAN_POINT ( 'NONE',  ( -18.05918829504999934, 2.872909508741170015, 63.35000000000700027 ) ) ;
#2976=ORIENTED_EDGE ( 'NONE', *, *, #5277, .F. ) ;
#2978=DIRECTION ( 'NONE',  ( -1.000000000000000000, 0.000000000000000000, 0.000000000000000000 ) ) ;
#2979=DIRECTION ( 'NONE',  ( 0.000000000000000000, 0.000000000000000000, -1.000000000000000000 ) ) ;
#2991=CARTESIAN_POINT ( 'NONE',  ( -25.86749127492454647, -8.860076549334127805, 83.57661607529820458 ) ) ;
#2994=CARTESIAN_POINT ( 'NONE',  ( -18.59029969833234475, 30.35571874317119168, 61.67763804039374520 ) ) ;
#3000=VERTEX_POINT ( 'NONE', #2839 ) ;
#3001=EDGE_CURVE ( 'NONE', #349, #4986, #5116, .T. ) ;
#3003=DIRECTION ( 'NONE',  ( 0.4528443260392608916, 0.8915896008669279560, 0.000000000000000000 ) ) ;
#3005=VERTEX_POINT ( 'NONE', #8263 ) ;
#3008=EDGE_CURVE ( 'NONE', #11514, #7434, #2917, .T. ) ;
#3009=CIRCLE ( 'NONE', #7202, 16.95000000000000284 ) ;
#3010=DIRECTION ( 'NONE',  ( 0.000000000000000000, 0.000000000000000000, -1.000000000000000000 ) ) ;
#3013=CARTESIAN_POINT ( 'NONE',  ( -18.05918829504999934, 10.97290950744599947, 61.72253826518770836 ) ) ;
#3014=DIRECTION ( 'NONE',  ( 0.000000000000000000, 0.000000000000000000, -1.000000000000000000 ) ) ;
#3016=DIRECTION ( 'NONE',  ( 0.000000000000000000, 0.000000000000000000, 1.000000000000000000 ) ) ;
#3018=EDGE_CURVE ( 'NONE', #12033, #11479, #11373, .T. ) ;
#3021=ORIENTED_EDGE ( 'NONE', *, *, #9218, .T. ) ;
#3023=ORIENTED_EDGE ( 'NONE', *, *, #8616, .F. ) ;
#3024=ORIENTED_EDGE ( 'NONE', *, *, #4670, .F. ) ;
#3025=DIRECTION ( 'NONE',  ( 0.000000000000000000, 0.000000000000000000, -1.000000000000000000 ) ) ;
#3026=EDGE_CURVE ( 'NONE', #10962, #1000, #1099, .T. ) ;
#3027=COLOUR_RGB ( '', 0.09019608, 0.27058824, 0.51372549) ;
#3029=CARTESIAN_POINT ( 'NONE',  ( -39.80918829504999934, -6.027090492554000534, 64.85000000000000853 ) ) ;
#3032=ORIENTED_EDGE ( 'NONE', *, *, #9599, .T. ) ;
#3033=CARTESIAN_POINT ( 'NONE',  ( -15.47476843086678677, 30.21612105669994364, 60.55881087961125075 ) ) ;
#3035=DIRECTION ( 'NONE',  ( 0.9496839325805418452, -0.3132098788326394545, 0.000000000000000000 ) ) ;
#3036=AXIS2_PLACEMENT_3D ( 'NONE', #4492, #8746, #11960 ) ;
#3037=DIRECTION ( 'NONE',  ( 0.000000000000000000, 1.000000000000000000, 0.000000000000000000 ) ) ;
#3038=VERTEX_POINT ( 'NONE', #5039 ) ;
#3041=DIRECTION ( 'NONE',  ( 0.000000000000000000, 0.000000000000000000, -1.000000000000000000 ) ) ;
#3043=CARTESIAN_POINT ( 'NONE',  ( -18.45035643575574014, 27.96940014844277300, 58.81168696388461825 ) ) ;
#3044=EDGE_CURVE ( 'NONE', #5798, #1784, #1987, .T. ) ;
#3045=FACE_OUTER_BOUND ( 'NONE', #6658, .T. ) ;
#3046=VERTEX_POINT ( 'NONE', #6018 ) ;
#3047=EDGE_LOOP ( 'NONE', ( #398, #4815, #9826, #2976 ) ) ;
#3048=ORIENTED_EDGE ( 'NONE', *, *, #10549, .F. ) ;
#3053=LINE ( 'NONE', #2991, #160 ) ;
#3054=VECTOR ( 'NONE', #10800, 1000.000000000000000 ) ;
#3055=CARTESIAN_POINT ( 'NONE',  ( -19.00868903206585259, 30.34086823226316909, 61.57150343037032059 ) ) ;
#3056=CARTESIAN_POINT ( 'NONE',  ( -18.94953701706641525, 26.94812814264477652, 56.14277197085647231 ) ) ;
#3059=EDGE_CURVE ( 'NONE', #12910, #4496, #9360, .T. ) ;
#3060=CARTESIAN_POINT ( 'NONE',  ( -5.789834139046019956, -5.598733283342819611, 7.250000000000000000 ) ) ;
#3067=ORIENTED_EDGE ( 'NONE', *, *, #2971, .T. ) ;
#3068=EDGE_LOOP ( 'NONE', ( #12650, #3380, #7473, #3172 ) ) ;
#3070=DIRECTION ( 'NONE',  ( 0.000000000000000000, 0.000000000000000000, 1.000000000000000000 ) ) ;
#3074=DIRECTION ( 'NONE',  ( 0.4528443260392610026, 0.8915896008669278450, 0.000000000000000000 ) ) ;
#3076=EDGE_CURVE ( 'NONE', #11380, #9897, #8936, .T. ) ;
#3078=DIRECTION ( 'NONE',  ( 1.000000000000000000, 0.000000000000000000, 0.000000000000000000 ) ) ;
#3080=EDGE_LOOP ( 'NONE', ( #8248, #300 ) ) ;
#3081=ADVANCED_FACE ( 'NONE', ( #7132 ), #8125, .T. ) ;
#3083=CARTESIAN_POINT ( 'NONE',  ( -20.76614708744390470, 15.25248827153688680, 68.78616702919012482 ) ) ;
#3084=EDGE_LOOP ( 'NONE', ( #11686, #5598, #11497, #3914 ) ) ;
#3086=CARTESIAN_POINT ( 'NONE',  ( -11.91335496205000055, 10.97290950744599947, 60.60999999999999943 ) ) ;
#3087=DIRECTION ( 'NONE',  ( 1.000000000000000000, 0.000000000000000000, 0.000000000000000000 ) ) ;
#3088=EDGE_CURVE ( 'NONE', #12241, #8398, #12389, .T. ) ;
#3089=DIRECTION ( 'NONE',  ( -0.4528443260392609471, -0.8915896008669278450, 0.000000000000000000 ) ) ;
#3093=ORIENTED_EDGE ( 'NONE', *, *, #8691, .T. ) ;
#3094=CARTESIAN_POINT ( 'NONE',  ( -14.66438022474483382, 30.11090903182021705, 55.34105990772840045 ) ) ;
#3095=AXIS2_PLACEMENT_3D ( 'NONE', #13480, #3988, #7380 ) ;
#3096=ORIENTED_EDGE ( 'NONE', *, *, #2244, .T. ) ;
#3097=ORIENTED_EDGE ( 'NONE', *, *, #2344, .T. ) ;
#3101=DIRECTION ( 'NONE',  ( -1.000000000000000000, 0.000000000000000000, 0.000000000000000000 ) ) ;
#3102=ORIENTED_EDGE ( 'NONE', *, *, #8920, .F. ) ;
#3106=CARTESIAN_POINT ( 'NONE',  ( -18.05918829504999223, 2.660265422445993622, 63.26601075299999621 ) ) ;
#3108=CIRCLE ( 'NONE', #8665, 7.833333332999988130 ) ;
#3111=CIRCLE ( 'NONE', #12235, 7.166108729582679970 ) ;
#3112=VERTEX_POINT ( 'NONE', #7449 ) ;
#3115=ORIENTED_EDGE ( 'NONE', *, *, #10827, .T. ) ;
#3116=ADVANCED_FACE ( 'NONE', ( #6305 ), #4485, .F. ) ;
#3117=ORIENTED_EDGE ( 'NONE', *, *, #6995, .F. ) ;
#3120=CIRCLE ( 'NONE', #13128, 24.92993838181874722 ) ;
#3121=CARTESIAN_POINT ( 'NONE',  ( -18.05918829504999934, 10.97290950744599947, 31.09999999999999787 ) ) ;
#3123=AXIS2_PLACEMENT_3D ( 'NONE', #7561, #5271, #3333 ) ;
#3125=CARTESIAN_POINT ( 'NONE',  ( -18.19085538481590447, 26.97290194241137584, 55.85005112132051863 ) ) ;
#3126=DIRECTION ( 'NONE',  ( 0.000000000000000000, 0.000000000000000000, -1.000000000000000000 ) ) ;
#3129=AXIS2_PLACEMENT_3D ( 'NONE', #12848, #9579, #5378 ) ;
#3132=AXIS2_PLACEMENT_3D ( 'NONE', #3203, #6534, #10801 ) ;
#3137=LINE ( 'NONE', #6334, #1124 ) ;
#3138=CARTESIAN_POINT ( 'NONE',  ( -38.38077571930826082, -0.4981161769137699147, 83.57661607529820458 ) ) ;
#3139=CARTESIAN_POINT ( 'NONE',  ( -25.05563313235659706, -2.802149825948039741, 60.65000000000000568 ) ) ;
#3141=VERTEX_POINT ( 'NONE', #12731 ) ;
#3143=CARTESIAN_POINT ( 'NONE',  ( -35.05918829505000645, -6.027090492554000534, 58.85000000000000142 ) ) ;
#3145=ORIENTED_EDGE ( 'NONE', *, *, #5943, .F. ) ;
#3147=ORIENTED_EDGE ( 'NONE', *, *, #9899, .T. ) ;
#3148=VECTOR ( 'NONE', #13453, 1000.000000000000000 ) ;
#3149=LINE ( 'NONE', #3419, #2150 ) ;
#3150=ORIENTED_EDGE ( 'NONE', *, *, #10856, .F. ) ;
#3152=CIRCLE ( 'NONE', #8267, 10.00000000000000178 ) ;
#3155=ORIENTED_EDGE ( 'NONE', *, *, #13454, .F. ) ;
#3156=ORIENTED_EDGE ( 'NONE', *, *, #6086, .T. ) ;
#3157=DIRECTION ( 'NONE',  ( 0.4528443260392610026, 0.8915896008669278450, 0.000000000000000000 ) ) ;
#3158=ORIENTED_EDGE ( 'NONE', *, *, #10760, .T. ) ;
#3162=ADVANCED_FACE ( 'NONE', ( #9794 ), #1118, .F. ) ;
#3164=AXIS2_PLACEMENT_3D ( 'NONE', #777, #5033, #9305 ) ;
#3165=AXIS2_PLACEMENT_3D ( 'NONE', #13386, #4743, #11033 ) ;
#3166=AXIS2_PLACEMENT_3D ( 'NONE', #12823, #2446, #1295 ) ;
#3167=VERTEX_POINT ( 'NONE', #12 ) ;
#3168=EDGE_CURVE ( 'NONE', #8341, #8660, #9140, .T. ) ;
#3169=FACE_OUTER_BOUND ( 'NONE', #13474, .T. ) ;
#3170=ORIENTED_EDGE ( 'NONE', *, *, #11254, .F. ) ;
#3172=ORIENTED_EDGE ( 'NONE', *, *, #4934, .F. ) ;
#3174=DIRECTION ( 'NONE',  ( 0.000000000000000000, 0.000000000000000000, -1.000000000000000000 ) ) ;
#3175=MECHANICAL_DESIGN_GEOMETRIC_PRESENTATION_REPRESENTATION('',(#6501),#11190);
#3177=CONICAL_SURFACE ( 'NONE', #12081, 6.419999999999999929, 0.2165503049760889864 ) ;
#3178=CYLINDRICAL_SURFACE ( 'NONE', #12308, 24.92993838181874722 ) ;
#3179=AXIS2_PLACEMENT_3D ( 'NONE', #238, #5458, #1139 ) ;
#3183=ADVANCED_FACE ( 'NONE', ( #4350 ), #4455, .T. ) ;
#3187=EDGE_LOOP ( 'NONE', ( #1198, #10556 ) ) ;
#3188=EDGE_LOOP ( 'NONE', ( #3720, #11391, #585, #6231 ) ) ;
#3189=ORIENTED_EDGE ( 'NONE', *, *, #847, .T. ) ;
#3190=ORIENTED_EDGE ( 'NONE', *, *, #9452, .F. ) ;
#3191=LINE ( 'NONE', #2136, #3972 ) ;
#3192=CARTESIAN_POINT ( 'NONE',  ( -18.05918829504999934, 10.97290950744599947, 61.85000000000000142 ) ) ;
#3195=PLANE ( 'NONE',  #9184 ) ;
#3199=DIRECTION ( 'NONE',  ( 0.000000000000000000, 0.000000000000000000, 1.000000000000000000 ) ) ;
#3202=ORIENTED_EDGE ( 'NONE', *, *, #3026, .F. ) ;
#3203=CARTESIAN_POINT ( 'NONE',  ( -18.05918829504999934, 10.97290950744599947, 6.250000000000000000 ) ) ;
#3204=DIRECTION ( 'NONE',  ( -0.2000659497483225358, 0.000000000000000000, 0.9797824328652262604 ) ) ;
#3205=DIRECTION ( 'NONE',  ( 0.000000000000000000, 0.000000000000000000, 1.000000000000000000 ) ) ;
#3206=CARTESIAN_POINT ( 'NONE',  ( -20.43440950813489465, 30.23850757514860987, 53.93886540776640715 ) ) ;
#3207=PRESENTATION_STYLE_ASSIGNMENT (( #5270 ) ) ;
#3209=LINE ( 'NONE', #4583, #12902 ) ;
#3212=DIRECTION ( 'NONE',  ( -1.000000000000000000, 0.000000000000000000, 0.000000000000000000 ) ) ;
#3213=EDGE_CURVE ( 'NONE', #2573, #6884, #6509, .T. ) ;
#3214=ADVANCED_FACE ( 'NONE', ( #9720 ), #1027, .T. ) ;
#3215=B_SPLINE_CURVE_WITH_KNOTS ( 'NONE', 3,
 ( #7559, #7636, #42, #10731, #12958, #1217, #4315, #11919, #1153, #2371, #11980, #6596, #5470, #2155, #4377, #4242, #1291, #9832, #254, #8772, #4519, #9614, #13027, #6336, #8490, #5410, #171, #9747, #6538, #10659, #12759, #11846, #3206, #3270, #9686, #7422, #11711, #7479, #6392, #8622, #5338, #11771, #12884, #2301, #13301, #12264, #13094, #8983, #456, #324, #7916, #3615, #4788, #9114, #5620, #8908, #6745, #3740, #7777, #12190, #10037, #10948, #383, #2575, #11018, #4580, #13239, #13369, #7850, #11218, #1366, #11142, #5677, #3678, #6804, #4725, #9043, #12126, #3813, #2641, #4854, #7990, #4654, #6873, #1570, #9900, #13167, #5821, #10107, #5890, #527, #2716, #8833, #10173, #6943, #592, #11078, #8066, #1495, #12052, #2441, #5750, #1641, #6670, #9957, #2506, #3541, #1433, #12467, #11283, #8343, #5949, #4024, #1705, #942, #2923, #1858, #11421, #2850, #11482, #9465, #8131, #3885, #10433, #1920, #6095, #12340, #12540, #10367, #9320, #5051, #866, #8196, #3055, #11550, #7270, #7070, #4095, #2994, #7146, #10243 ),
 .UNSPECIFIED., .F., .F.,
 ( 4, 2, 1, 1, 2, 2, 2, 2, 1, 1, 2, 2, 2, 2, 1, 1, 1, 2, 2, 2, 2, 2, 2, 2, 1, 1, 2, 2, 2, 2, 1, 1, 2, 2, 2, 2, 1, 2, 2, 2, 2, 2, 1, 1, 2, 2, 2, 2, 1, 1, 2, 2, 2, 2, 1, 1, 1, 1, 2, 2, 2, 2, 1, 1, 2, 2, 2, 2, 1, 1, 2, 2, 2, 2, 1, 1, 2, 2, 2, 2, 1, 2, 2, 4 ),
 ( 0.000000000000000000, 0.03124999999999248518, 0.04687499999998832878, 0.05468749999998662875, 0.05859374999998540057, 0.06249999999998417932, 0.09374999999997543632, 0.1093749999999707873, 0.1171874999999681366, 0.1210937499999661798, 0.1230468749999651668, 0.1249999999999641537, 0.1562499999999368283, 0.1718749999999231726, 0.1796874999999160116, 0.1835937499999121536, 0.1855468749999106548, 0.1865234374999094891, 0.1874999999999083233, 0.2031249999998842315, 0.2109374999998713529, 0.2187499999998585021, 0.2343749999998327449, 0.2421874999998198941, 0.2460937499998124556, 0.2480468749998095412, 0.2490234374998080702, 0.2499999999998066269, 0.2812499999997721267, 0.2968749999997541966, 0.3046874999997454814, 0.3085937499997403743, 0.3105468749997369882, 0.3124999999997335465, 0.3437499999996858069, 0.3593749999996613265, 0.3671874999996497246, 0.3710937499996447286, 0.3749999999996397881, 0.4999999999995009548, 0.5624999999994307887, 0.5937499999993955946, 0.6093749999993778310, 0.6171874999993681721, 0.6210937499993626210, 0.6249999999993569588, 0.6562499999993113287, 0.6718749999992886801, 0.6796874999992780220, 0.6835937499992728039, 0.6855468749992702504, 0.6874999999992676969, 0.7187499999992266186, 0.7343749999992060795, 0.7421874999991949773, 0.7460937499991895372, 0.7480468749991875388, 0.7490234374991859845, 0.7495117187491852073, 0.7499999999991844302, 0.7656249999992359445, 0.7734374999992611466, 0.7773437499992736921, 0.7792968749992797983, 0.7802734374992826849, 0.7812499999992855715, 0.7968749999993441913, 0.8046874999993740563, 0.8085937499993888222, 0.8105468749993962607, 0.8115234374994000355, 0.8124999999994038102, 0.8437499999995105027, 0.8593749999995646816, 0.8671874999995913269, 0.8710937499996049826, 0.8730468749996114219, 0.8749999999996178612, 0.9062499999997141176, 0.9218749999997626343, 0.9296874999997862821, 0.9335937499997979394, 0.9374999999998094857, 1.000000000000000000 ),
 .UNSPECIFIED. ) ;
#3221=ORIENTED_EDGE ( 'NONE', *, *, #4950, .T. ) ;
#3223=CARTESIAN_POINT ( 'NONE',  ( -13.37752337641431133, 8.435598762370004167, 68.52507220045593783 ) ) ;
#3227=EDGE_CURVE ( 'NONE', #11675, #8158, #2254, .T. ) ;
#3228=CARTESIAN_POINT ( 'NONE',  ( -26.45502162804999813, 10.97290950744599947, 60.75000000000000000 ) ) ;
#3230=ADVANCED_FACE ( 'NONE', ( #1404 ), #7744, .F. ) ;
#3231=UNCERTAINTY_MEASURE_WITH_UNIT (LENGTH_MEASURE( 1.000000000000000082E-05 ), #8984, 'distance_accuracy_value', 'NONE');
#3233=CARTESIAN_POINT ( 'NONE',  ( -15.72734351507429018, 30.24295657546931437, 53.90012880255799388 ) ) ;
#3234=ORIENTED_EDGE ( 'NONE', *, *, #7822, .T. ) ;
#3235=EDGE_LOOP ( 'NONE', ( #6189, #6441, #9842, #9712, #11213, #11229 ) ) ;
#3236=DIRECTION ( 'NONE',  ( 0.000000000000000000, 0.000000000000000000, 1.000000000000000000 ) ) ;
#3239=ORIENTED_EDGE ( 'NONE', *, *, #7622, .T. ) ;
#3240=DIRECTION ( 'NONE',  ( 0.000000000000000000, 0.000000000000000000, -1.000000000000000000 ) ) ;
#3243=EDGE_CURVE ( 'NONE', #12583, #6548, #5565, .T. ) ;
#3244=CARTESIAN_POINT ( 'NONE',  ( -18.05918829504999934, 7.130333642789880244, 7.250000000000000000 ) ) ;
#3245=ORIENTED_EDGE ( 'NONE', *, *, #12256, .T. ) ;
#3246=ORIENTED_EDGE ( 'NONE', *, *, #10760, .F. ) ;
#3247=ADVANCED_FACE ( 'NONE', ( #2411 ), #7954, .T. ) ;
#3248=AXIS2_PLACEMENT_3D ( 'NONE', #6575, #5518, #17 ) ;
#3249=CARTESIAN_POINT ( 'NONE',  ( -4.640588396653431147, -14.07073191448199978, 7.250000000000000000 ) ) ;
#3252=VERTEX_POINT ( 'NONE', #502 ) ;
#3254=CARTESIAN_POINT ( 'NONE',  ( -25.86749127492454647, -8.860076549334124252, 17.25000000000000000 ) ) ;
#3257=DIRECTION ( 'NONE',  ( -1.000000000000000000, -1.792228749776982873E-15, 0.000000000000000000 ) ) ;
#3258=DIRECTION ( 'NONE',  ( -1.000000000000000000, 0.000000000000000000, 0.000000000000000000 ) ) ;
#3266=VERTEX_POINT ( 'NONE', #4620 ) ;
#3267=DIRECTION ( 'NONE',  ( -1.000000000000000000, 0.000000000000000000, 0.000000000000000000 ) ) ;
#3269=LINE ( 'NONE', #8832, #11329 ) ;
#3270=CARTESIAN_POINT ( 'NONE',  ( -20.46141587662859607, 30.23571878071122399, 53.96345633405123721 ) ) ;
#3271=( LENGTH_UNIT ( ) NAMED_UNIT ( * ) SI_UNIT ( .MILLI., .METRE. ) );
#3272=ORIENTED_EDGE ( 'NONE', *, *, #9094, .F. ) ;
#3273=CARTESIAN_POINT ( 'NONE',  ( -5.631644894983189431, 10.97290950744599947, 5.250000000000000000 ) ) ;
#3281=ORIENTED_EDGE ( 'NONE', *, *, #3801, .F. ) ;
#3282=DIRECTION ( 'NONE',  ( 0.000000000000000000, 0.000000000000000000, 1.000000000000000000 ) ) ;
#3283=AXIS2_PLACEMENT_3D ( 'NONE', #762, #2042, #3157 ) ;
#3286=CARTESIAN_POINT ( 'NONE',  ( -16.81378748857474292, 5.403809379663265133, 68.16287202337919382 ) ) ;
#3288=DIRECTION ( 'NONE',  ( 0.000000000000000000, 0.000000000000000000, -1.000000000000000000 ) ) ;
#3289=DIRECTION ( 'NONE',  ( 0.000000000000000000, 0.000000000000000000, 1.000000000000000000 ) ) ;
#3290=ADVANCED_FACE ( 'NONE', ( #1542 ), #12997, .T. ) ;
#3291=ORIENTED_EDGE ( 'NONE', *, *, #7389, .T. ) ;
#3292=DIRECTION ( 'NONE',  ( 0.000000000000000000, 0.000000000000000000, -1.000000000000000000 ) ) ;
#3293=DIRECTION ( 'NONE',  ( 0.6615960714621565986, -0.7498604124941127269, 0.000000000000000000 ) ) ;
#3297=VECTOR ( 'NONE', #11433, 1000.000000000000000 ) ;
#3299=CARTESIAN_POINT ( 'NONE',  ( -1.059188295049996231, 27.97290950744599769, 58.85000000000000142 ) ) ;
#3301=AXIS2_PLACEMENT_3D ( 'NONE', #12280, #1061, #12411 ) ;
#3303=FACE_OUTER_BOUND ( 'NONE', #1929, .T. ) ;
#3305=ADVANCED_FACE ( 'NONE', ( #5862 ), #6778, .F. ) ;
#3307=ORIENTED_EDGE ( 'NONE', *, *, #50, .T. ) ;
#3310=ORIENTED_EDGE ( 'NONE', *, *, #10363, .T. ) ;
#3311=FACE_OUTER_BOUND ( 'NONE', #2766, .T. ) ;
#3316=CIRCLE ( 'NONE', #11348, 16.95000000000000284 ) ;
#3319=EDGE_CURVE ( 'NONE', #12272, #5077, #3444, .T. ) ;
#3322=CONICAL_SURFACE ( 'NONE', #13339, 2.500000000000000000, 0.7853981633974532750 ) ;
#3326=ORIENTED_EDGE ( 'NONE', *, *, #11763, .F. ) ;
#3329=CARTESIAN_POINT ( 'NONE',  ( -5.789834139046009298, 27.54455229823479812, 68.85549045786049760 ) ) ;
#3331=DIRECTION ( 'NONE',  ( -1.000000000000000000, 0.000000000000000000, 0.000000000000000000 ) ) ;
#3333=DIRECTION ( 'NONE',  ( -1.000000000000000000, 0.000000000000000000, 0.000000000000000000 ) ) ;
#3339=VECTOR ( 'NONE', #12815, 1000.000000000000000 ) ;
#3340=ORIENTED_EDGE ( 'NONE', *, *, #5418, .F. ) ;
#3345=EDGE_LOOP ( 'NONE', ( #11250, #12664 ) ) ;
#3346=ORIENTED_EDGE ( 'NONE', *, *, #9820, .F. ) ;
#3347=PLANE ( 'NONE',  #1722 ) ;
#3351=SURFACE_STYLE_USAGE ( .BOTH. , #58 ) ;
#3353=CARTESIAN_POINT ( 'NONE',  ( -5.309188295050000228, 27.97290950744599769, 64.35000000000000853 ) ) ;
#3354=ADVANCED_FACE ( 'NONE', ( #5997 ), #3858, .F. ) ;
#3355=CARTESIAN_POINT ( 'NONE',  ( -35.05918829505000645, 27.97290950744599769, 64.35000000000000853 ) ) ;
#3356=DIRECTION ( 'NONE',  ( 0.000000000000000000, 0.000000000000000000, -1.000000000000000000 ) ) ;
#3357=B_SPLINE_CURVE_WITH_KNOTS ( 'NONE', 3,
 ( #4616, #5857, #2678, #7883 ),
 .UNSPECIFIED., .F., .F.,
 ( 4, 4 ),
 ( 0.000000000000000000, 1.000000000000000000 ),
 .UNSPECIFIED. ) ;
#3360=AXIS2_PLACEMENT_3D ( 'NONE', #9891, #649, #4783 ) ;
#3362=CARTESIAN_POINT ( 'NONE',  ( -15.26746632920534807, 30.19191053447994832, 54.37610708475375532 ) ) ;
#3363=ORIENTED_EDGE ( 'NONE', *, *, #8433, .F. ) ;
#3365=CARTESIAN_POINT ( 'NONE',  ( -25.86749127492454647, -8.860076549334127805, 5.250000000000000000 ) ) ;
#3371=CIRCLE ( 'NONE', #5132, 15.45000000000000462 ) ;
#3373=VECTOR ( 'NONE', #2193, 1000.000000000000000 ) ;
#3375=CARTESIAN_POINT ( 'NONE',  ( -5.631644894983189431, 10.97290950744599947, 83.57661607529820458 ) ) ;
#3377=EDGE_CURVE ( 'NONE', #9938, #10214, #4465, .T. ) ;
#3378=ORIENTED_EDGE ( 'NONE', *, *, #5201, .F. ) ;
#3379=AXIS2_PLACEMENT_3D ( 'NONE', #6076, #3931, #3101 ) ;
#3380=ORIENTED_EDGE ( 'NONE', *, *, #2226, .T. ) ;
#3382=AXIS2_PLACEMENT_3D ( 'NONE', #8294, #12689, #5545 ) ;
#3383=CIRCLE ( 'NONE', #5158, 4.749999999999997335 ) ;
#3384=ORIENTED_EDGE ( 'NONE', *, *, #8868, .T. ) ;
#3385=ORIENTED_EDGE ( 'NONE', *, *, #12200, .F. ) ;
#3387=CARTESIAN_POINT ( 'NONE',  ( -32.35918829505000360, -6.027090492554000534, 64.85000000000000853 ) ) ;
#3389=VERTEX_POINT ( 'NONE', #6069 ) ;
#3390=DIRECTION ( 'NONE',  ( 0.000000000000000000, -1.000000000000000000, 2.732534507816519619E-15 ) ) ;
#3391=CARTESIAN_POINT ( 'NONE',  ( -5.631644894983189431, 10.97290950744599947, 17.25000000000000000 ) ) ;
#3394=PLANE ( 'NONE',  #7794 ) ;
#3395=CONICAL_SURFACE ( 'NONE', #1141, 16.00000000000000000, 0.7853981633974476129 ) ;
#3397=EDGE_LOOP ( 'NONE', ( #10408, #8059, #549, #7608 ) ) ;
#3398=AXIS2_PLACEMENT_3D ( 'NONE', #4732, #8987, #658 ) ;
#3400=ORIENTED_EDGE ( 'NONE', *, *, #12092, .T. ) ;
#3402=COLOUR_RGB ( '', 0.09019608, 0.27058824, 0.51372549) ;
#3403=CARTESIAN_POINT ( 'NONE',  ( -5.631644894983189431, 10.97290950744599947, 17.25000000000000000 ) ) ;
#3405=ORIENTED_EDGE ( 'NONE', *, *, #4813, .F. ) ;
#3406=DIRECTION ( 'NONE',  ( 1.000000000000000000, 0.000000000000000000, 0.000000000000000000 ) ) ;
#3408=CARTESIAN_POINT ( 'NONE',  ( -28.87730642030694739, 29.81324547859995278, 83.57661607529820458 ) ) ;
#3409=ORIENTED_EDGE ( 'NONE', *, *, #5244, .F. ) ;
#3410=CARTESIAN_POINT ( 'NONE',  ( -18.05918829504999934, 10.97290950744599947, 61.10999999999999943 ) ) ;
#3414=ADVANCED_FACE ( 'NONE', ( #769 ), #9364, .T. ) ;
#3416=ADVANCED_FACE ( 'NONE', ( #3921 ), #8108, .F. ) ;
#3419=CARTESIAN_POINT ( 'NONE',  ( -28.87730642030694739, 29.81324547859995278, 5.250000000000000000 ) ) ;
#3421=ORIENTED_EDGE ( 'NONE', *, *, #6752, .T. ) ;
#3425=AXIS2_PLACEMENT_3D ( 'NONE', #4992, #593, #1787 ) ;
#3426=DIRECTION ( 'NONE',  ( 0.000000000000000000, 0.000000000000000000, -1.000000000000000000 ) ) ;
#3427=DIRECTION ( 'NONE',  ( -0.3132098788326400096, -0.9496839325805418452, 0.000000000000000000 ) ) ;
#3431=DIRECTION ( 'NONE',  ( -1.000000000000000000, 0.000000000000000000, 0.000000000000000000 ) ) ;
#3432=CARTESIAN_POINT ( 'NONE',  ( -18.05918829504999934, 10.97290950744599947, 64.54999999999999716 ) ) ;
#3433=EDGE_CURVE ( 'NONE', #6919, #10012, #9381, .T. ) ;
#3436=ADVANCED_FACE ( 'NONE', ( #3783 ), #5347, .F. ) ;
#3437=CARTESIAN_POINT ( 'NONE',  ( -16.76578548723817974, 30.32455137611084339, 53.24728338428077734 ) ) ;
#3438=ORIENTED_EDGE ( 'NONE', *, *, #12712, .F. ) ;
#3439=DIRECTION ( 'NONE',  ( -1.000000000000000000, 0.000000000000000000, 0.000000000000000000 ) ) ;
#3444=LINE ( 'NONE', #293, #2479 ) ;
#3446=VERTEX_POINT ( 'NONE', #4899 ) ;
#3448=EDGE_LOOP ( 'NONE', ( #9481, #9079 ) ) ;
#3451=VERTEX_POINT ( 'NONE', #1750 ) ;
#3453=ORIENTED_EDGE ( 'NONE', *, *, #1091, .F. ) ;
#3461=CARTESIAN_POINT ( 'NONE',  ( -18.05918829504999934, 10.97290950744599947, 62.14999999999999858 ) ) ;
#3465=CARTESIAN_POINT ( 'NONE',  ( -11.74835982676941981, -4.028726038184999858, 63.45000000000000284 ) ) ;
#3467=ORIENTED_EDGE ( 'NONE', *, *, #865, .F. ) ;
#3468=DIRECTION ( 'NONE',  ( -1.000000000000000000, 0.000000000000000000, 0.000000000000000000 ) ) ;
#3469=EDGE_CURVE ( 'NONE', #722, #3590, #4964, .T. ) ;
#3471=CIRCLE ( 'NONE', #8577, 2.700000000000000178 ) ;
#3472=PLANE ( 'NONE',  #5823 ) ;
#3473=FACE_OUTER_BOUND ( 'NONE', #5597, .T. ) ;
#3475=CARTESIAN_POINT ( 'NONE',  ( -22.02876472382295248, 15.47207198241065029, 68.84999999999999432 ) ) ;
#3476=CARTESIAN_POINT ( 'NONE',  ( -0.05918829504999999908, 10.97290950744599947, 63.54999999999999716 ) ) ;
#3477=ADVANCED_FACE ( 'NONE', ( #5837 ), #397, .T. ) ;
#3478=FACE_OUTER_BOUND ( 'NONE', #7672, .T. ) ;
#3480=AXIS2_PLACEMENT_3D ( 'NONE', #11448, #10542, #7103 ) ;
#3481=EDGE_LOOP ( 'NONE', ( #13585, #6359, #8115, #13699 ) ) ;
#3482=ORIENTED_EDGE ( 'NONE', *, *, #13758, .F. ) ;
#3483=DIRECTION ( 'NONE',  ( -0.6615960714621564875, 0.7498604124941129490, 0.000000000000000000 ) ) ;
#3484=ORIENTED_EDGE ( 'NONE', *, *, #12002, .F. ) ;
#3485=CARTESIAN_POINT ( 'NONE',  ( -25.73489962141550080, -4.139534227248430120, 57.54999999999999716 ) ) ;
#3486=ADVANCED_FACE ( 'NONE', ( #2455, #5899 ), #13181, .F. ) ;
#3491=ORIENTED_EDGE ( 'NONE', *, *, #8319, .F. ) ;
#3492=CYLINDRICAL_SURFACE ( 'NONE', #10668, 8.395833332999997012 ) ;
#3493=DIRECTION ( 'NONE',  ( 0.000000000000000000, 0.000000000000000000, 1.000000000000000000 ) ) ;
#3497=EDGE_CURVE ( 'NONE', #6884, #5387, #7565, .T. ) ;
#3499=ORIENTED_EDGE ( 'NONE', *, *, #2064, .F. ) ;
#3500=CARTESIAN_POINT ( 'NONE',  ( -18.05918829504999934, 30.47290950744599769, 57.35000000000000142 ) ) ;
#3501=ADVANCED_FACE ( 'NONE', ( #4738, #4869 ), #10184, .F. ) ;
#3502=ORIENTED_EDGE ( 'NONE', *, *, #6345, .T. ) ;
#3503=DIRECTION ( 'NONE',  ( -0.6615960714621564875, 0.7498604124941129490, 0.000000000000000000 ) ) ;
#3504=CARTESIAN_POINT ( 'NONE',  ( -18.05918829504999934, 10.97290950744599947, 57.35000000000000142 ) ) ;
#3506=DIRECTION ( 'NONE',  ( -0.4678190685372686231, 0.5302313826179265721, 0.7071067811865505703 ) ) ;
#3507=DIRECTION ( 'NONE',  ( 0.6615960714621574867, -0.7498604124941119498, 0.000000000000000000 ) ) ;
#3508=AXIS2_PLACEMENT_3D ( 'NONE', #9288, #4063, #13476 ) ;
#3511=ORIENTED_EDGE ( 'NONE', *, *, #5834, .T. ) ;
#3518=ORIENTED_EDGE ( 'NONE', *, *, #7957, .F. ) ;
#3520=DIRECTION ( 'NONE',  ( -0.6615960714621569316, 0.7498604124941123938, 0.000000000000000000 ) ) ;
#3522=ORIENTED_EDGE ( 'NONE', *, *, #2424, .F. ) ;
#3523=CYLINDRICAL_SURFACE ( 'NONE', #2744, 6.850000000000002309 ) ;
#3525=CARTESIAN_POINT ( 'NONE',  ( -25.73489962141544751, -4.139534227248430120, 57.35000000000000142 ) ) ;
#3526=EDGE_CURVE ( 'NONE', #4562, #12584, #10967, .T. ) ;
#3529=CIRCLE ( 'NONE', #6414, 4.250000000000003553 ) ;
#3532=ORIENTED_EDGE ( 'NONE', *, *, #10071, .F. ) ;
#3534=LINE ( 'NONE', #2572, #11967 ) ;
#3536=CIRCLE ( 'NONE', #2880, 33.00000000000000000 ) ;
#3537=PRESENTATION_STYLE_ASSIGNMENT (( #12443 ) ) ;
#3538=VECTOR ( 'NONE', #8912, 1000.000000000000000 ) ;
#3539=VECTOR ( 'NONE', #13114, 1000.000000000000000 ) ;
#3541=CARTESIAN_POINT ( 'NONE',  ( -20.59415145364857835, 30.22157476193357439, 60.60836344892124572 ) ) ;
#3542=SURFACE_STYLE_FILL_AREA ( #2643 ) ;
#3546=DIRECTION ( 'NONE',  ( 0.4528443260392608916, 0.8915896008669279560, 0.000000000000000000 ) ) ;
#3547=DIRECTION ( 'NONE',  ( 1.000000000000000000, 0.000000000000000000, 0.000000000000000000 ) ) ;
#3549=ORIENTED_EDGE ( 'NONE', *, *, #10332, .F. ) ;
#3550=EDGE_CURVE ( 'NONE', #5721, #1952, #7129, .T. ) ;
#3554=CIRCLE ( 'NONE', #1536, 7.618085573000000110 ) ;
#3555=ORIENTED_EDGE ( 'NONE', *, *, #767, .T. ) ;
#3564=DIRECTION ( 'NONE',  ( -1.000000000000000000, 0.000000000000000000, 0.000000000000000000 ) ) ;
#3568=CARTESIAN_POINT ( 'NONE',  ( -35.05918829505000645, 10.97290950744599947, 57.35000000000000142 ) ) ;
#3570=CONICAL_SURFACE ( 'NONE', #11362, 2.500000000000000000, 0.7853981633974532750 ) ;
#3571=LINE ( 'NONE', #13257, #1754 ) ;
#3572=EDGE_CURVE ( 'NONE', #952, #533, #13310, .T. ) ;
#3574=EDGE_LOOP ( 'NONE', ( #6516, #2015 ) ) ;
#3575=AXIS2_PLACEMENT_3D ( 'NONE', #9248, #1775, #4010 ) ;
#3576=DIRECTION ( 'NONE',  ( 1.000000000000000000, 0.000000000000000000, 0.000000000000000000 ) ) ;
#3578=CIRCLE ( 'NONE', #6677, 17.50000000000000355 ) ;
#3579=ORIENTED_EDGE ( 'NONE', *, *, #12811, .T. ) ;
#3587=ADVANCED_FACE ( 'NONE', ( #8923 ), #13105, .F. ) ;
#3589=CARTESIAN_POINT ( 'NONE',  ( -16.66803132855381619, 30.31858837286686637, 61.40807488358109367 ) ) ;
#3590=VERTEX_POINT ( 'NONE', #4797 ) ;
#3598=AXIS2_PLACEMENT_3D ( 'NONE', #9773, #197, #679 ) ;
#3599=CARTESIAN_POINT ( 'NONE',  ( -18.05918829505001355, 3.364325185446006117, 61.98378871700002435 ) ) ;
#3600=DIRECTION ( 'NONE',  ( -0.4678190685372707325, 0.5302313826179287926, 0.7071067811865475727 ) ) ;
#3604=FACE_OUTER_BOUND ( 'NONE', #11042, .T. ) ;
#3606=AXIS2_PLACEMENT_3D ( 'NONE', #4445, #5930, #13348 ) ;
#3607=AXIS2_PLACEMENT_3D ( 'NONE', #57, #12979, #7498 ) ;
#3614=ORIENTED_EDGE ( 'NONE', *, *, #4766, .F. ) ;
#3615=CARTESIAN_POINT ( 'NONE',  ( -21.25220226754673547, 30.13979931660498579, 54.95335517942023529 ) ) ;
#3617=AXIS2_PLACEMENT_3D ( 'NONE', #6240, #10513, #9256 ) ;
#3618=( NAMED_UNIT ( * ) SI_UNIT ( $, .STERADIAN. ) SOLID_ANGLE_UNIT ( ) );
#3619=DIRECTION ( 'NONE',  ( 0.000000000000000000, 0.000000000000000000, -1.000000000000000000 ) ) ;
#3620=VECTOR ( 'NONE', #6750, 1000.000000000000000 ) ;
#3621=PLANE ( 'NONE',  #6436 ) ;
#3623=FACE_OUTER_BOUND ( 'NONE', #476, .T. ) ;
#3630=CARTESIAN_POINT ( 'NONE',  ( -18.05918829504999934, 10.97290950744599947, 63.35000000000000142 ) ) ;
#3632=FILL_AREA_STYLE_COLOUR ( '', #1501 ) ;
#3634=DIRECTION ( 'NONE',  ( 1.000000000000000000, 0.000000000000000000, 0.000000000000000000 ) ) ;
#3635=FACE_OUTER_BOUND ( 'NONE', #6512, .T. ) ;
#3636=EDGE_CURVE ( 'NONE', #6678, #12858, #13108, .T. ) ;
#3637=DIRECTION ( 'NONE',  ( 0.000000000000000000, 0.000000000000000000, -1.000000000000000000 ) ) ;
#3638=CARTESIAN_POINT ( 'NONE',  ( -10.25088531517539714, 30.80589556422609832, 5.250000000000000000 ) ) ;
#3641=AXIS2_PLACEMENT_3D ( 'NONE', #12885, #8423, #1020 ) ;
#3642=DIRECTION ( 'NONE',  ( 0.000000000000000000, -1.000000000000000000, 0.000000000000000000 ) ) ;
#3650=CARTESIAN_POINT ( 'NONE',  ( -35.05918829505000645, -6.027090492554000534, 68.85549045786049760 ) ) ;
#3651=DIRECTION ( 'NONE',  ( 0.000000000000000000, 0.000000000000000000, -1.000000000000000000 ) ) ;
#3655=AXIS2_PLACEMENT_3D ( 'NONE', #8643, #9311, #5492 ) ;
#3658=DIRECTION ( 'NONE',  ( 0.000000000000000000, 0.000000000000000000, 1.000000000000000000 ) ) ;
#3667=EDGE_LOOP ( 'NONE', ( #819, #8424 ) ) ;
#3668=DIRECTION ( 'NONE',  ( 0.000000000000000000, 0.000000000000000000, -1.000000000000000000 ) ) ;
#3670=FACE_OUTER_BOUND ( 'NONE', #1712, .T. ) ;
#3673=ORIENTED_EDGE ( 'NONE', *, *, #523, .F. ) ;
#3674=VERTEX_POINT ( 'NONE', #272 ) ;
#3678=CARTESIAN_POINT ( 'NONE',  ( -21.66168941035279971, 30.07924626547317715, 58.82219030866655629 ) ) ;
#3679=( NAMED_UNIT ( * ) SI_UNIT ( $, .STERADIAN. ) SOLID_ANGLE_UNIT ( ) );
#3681=CARTESIAN_POINT ( 'NONE',  ( -10.78334210919089919, -7.245613863947199640, 68.85549045786049760 ) ) ;
#3682=CARTESIAN_POINT ( 'NONE',  ( -9.663354962050000552, 10.97290950744599947, 60.04999999999999716 ) ) ;
#3683=CARTESIAN_POINT ( 'NONE',  ( -21.29702522623070138, 4.598043861247458786, 64.85000000000000853 ) ) ;
#3688=LINE ( 'NONE', #3485, #1802 ) ;
#3689=LINE ( 'NONE', #6686, #7276 ) ;
#3694=DIRECTION ( 'NONE',  ( -0.9496839325805427334, -0.3132098788326367345, 0.000000000000000000 ) ) ;
#3695=DIRECTION ( 'NONE',  ( -1.000000000000000000, 0.000000000000000000, 0.000000000000000000 ) ) ;
#3702=ORIENTED_EDGE ( 'NONE', *, *, #11265, .T. ) ;
#3703=CYLINDRICAL_SURFACE ( 'NONE', #9266, 0.9499999999999995115 ) ;
#3704=ORIENTED_EDGE ( 'NONE', *, *, #13261, .T. ) ;
#3706=AXIS2_PLACEMENT_3D ( 'NONE', #10377, #8351, #3003 ) ;
#3707=CARTESIAN_POINT ( 'NONE',  ( -1.059188295049996231, -6.027090492554000534, 64.85000000000000853 ) ) ;
#3710=DIRECTION ( 'NONE',  ( 0.000000000000000000, 0.000000000000000000, 1.000000000000000000 ) ) ;
#3711=DIRECTION ( 'NONE',  ( 0.000000000000000000, 0.000000000000000000, 1.000000000000000000 ) ) ;
#3712=AXIS2_PLACEMENT_3D ( 'NONE', #12049, #4648, #5674 ) ;
#3714=EDGE_CURVE ( 'NONE', #5137, #12100, #3688, .T. ) ;
#3715=ORIENTED_EDGE ( 'NONE', *, *, #10117, .F. ) ;
#3716=CARTESIAN_POINT ( 'NONE',  ( -18.05918829504999934, 19.07290950615085023, 63.35000000000700027 ) ) ;
#3719=ORIENTED_EDGE ( 'NONE', *, *, #1244, .F. ) ;
#3720=ORIENTED_EDGE ( 'NONE', *, *, #12377, .F. ) ;
#3722=FACE_OUTER_BOUND ( 'NONE', #12896, .T. ) ;
#3723=DIRECTION ( 'NONE',  ( 0.000000000000000000, 0.000000000000000000, -1.000000000000000000 ) ) ;
#3725=CARTESIAN_POINT ( 'NONE',  ( -18.05918829504998868, 19.27290950775476475, 63.26715728756898471 ) ) ;
#3726=EDGE_CURVE ( 'NONE', #12649, #3976, #1115, .T. ) ;
#3727=DIRECTION ( 'NONE',  ( 0.000000000000000000, 0.000000000000000000, -1.000000000000000000 ) ) ;
#3728=DIRECTION ( 'NONE',  ( -0.4528443260392610026, -0.8915896008669278450, 0.000000000000000000 ) ) ;
#3729=DIRECTION ( 'NONE',  ( 0.000000000000000000, 0.000000000000000000, 1.000000000000000000 ) ) ;
#3732=ADVANCED_FACE ( 'NONE', ( #9764 ), #477, .T. ) ;
#3734=ORIENTED_EDGE ( 'NONE', *, *, #9533, .F. ) ;
#3740=CARTESIAN_POINT ( 'NONE',  ( -21.43229256600465149, 30.11415384995645894, 55.29115902660671367 ) ) ;
#3742=DIRECTION ( 'NONE',  ( 0.000000000000000000, 0.000000000000000000, 1.000000000000000000 ) ) ;
#3745=CARTESIAN_POINT ( 'NONE',  ( -0.05918829504999999908, 10.97290950744599947, 63.45000000000000284 ) ) ;
#3751=AXIS2_PLACEMENT_3D ( 'NONE', #1512, #9978, #12070 ) ;
#3755=CARTESIAN_POINT ( 'NONE',  ( -5.173045190668890569, -15.68519459986890041, 17.25000000000000000 ) ) ;
#3756=SURFACE_SIDE_STYLE ('',( #5696 ) ) ;
#3757=ADVANCED_FACE ( 'NONE', ( #5633 ), #4706, .T. ) ;
#3758=DIRECTION ( 'NONE',  ( 0.000000000000000000, 0.000000000000000000, 1.000000000000000000 ) ) ;
#3760=CYLINDRICAL_SURFACE ( 'NONE', #5801, 2.700000000000001066 ) ;
#3762=DIRECTION ( 'NONE',  ( -1.000000000000000000, 0.000000000000000000, 0.000000000000000000 ) ) ;
#3763=LINE ( 'NONE', #4602, #1069 ) ;
#3764=CARTESIAN_POINT ( 'NONE',  ( -18.05918829504999934, 10.97290950744599947, 27.09999999999999787 ) ) ;
#3768=VECTOR ( 'NONE', #2338, 1000.000000000000000 ) ;
#3771=ORIENTED_EDGE ( 'NONE', *, *, #753, .F. ) ;
#3772=CARTESIAN_POINT ( 'NONE',  ( -30.48673169511680214, 10.97290950744599947, 68.85549045786049760 ) ) ;
#3773=AXIS2_PLACEMENT_3D ( 'NONE', #4607, #11240, #9062 ) ;
#3774=VECTOR ( 'NONE', #9752, 1000.000000000000000 ) ;
#3780=CARTESIAN_POINT ( 'NONE',  ( -5.809188295050001116, -6.027090492554000534, 68.85549045786049760 ) ) ;
#3783=FACE_OUTER_BOUND ( 'NONE', #8065, .T. ) ;
#3784=DIRECTION ( 'NONE',  ( 0.000000000000000000, 0.000000000000000000, -1.000000000000000000 ) ) ;
#3788=DIRECTION ( 'NONE',  ( -0.6615960714621568206, 0.7498604124941127269, 0.000000000000000000 ) ) ;
#3789=ORIENTED_EDGE ( 'NONE', *, *, #5785, .T. ) ;
#3790=FACE_OUTER_BOUND ( 'NONE', #3448, .T. ) ;
#3791=ORIENTED_EDGE ( 'NONE', *, *, #9309, .T. ) ;
#3793=VERTEX_POINT ( 'NONE', #7087 ) ;
#3795=DIRECTION ( 'NONE',  ( 0.000000000000000000, 0.000000000000000000, -1.000000000000000000 ) ) ;
#3796=VERTEX_POINT ( 'NONE', #2731 ) ;
#3797=CARTESIAN_POINT ( 'NONE',  ( -10.25088531517540069, -8.860076549334102936, 17.25000000000000000 ) ) ;
#3798=VECTOR ( 'NONE', #5693, 1000.000000000000000 ) ;
#3799=CARTESIAN_POINT ( 'NONE',  ( -7.241070169793059286, -7.867426463707969830, 5.250000000000000000 ) ) ;
#3801=EDGE_CURVE ( 'NONE', #11171, #7594, #11387, .T. ) ;
#3802=CARTESIAN_POINT ( 'NONE',  ( -35.05918829505000645, -6.027090492554000534, 58.85000000000000142 ) ) ;
#3804=DIRECTION ( 'NONE',  ( 0.000000000000000000, 0.000000000000000000, -1.000000000000000000 ) ) ;
#3805=AXIS2_PLACEMENT_3D ( 'NONE', #5839, #2936, #6108 ) ;
#3807=AXIS2_PLACEMENT_3D ( 'NONE', #1646, #13373, #9119 ) ;
#3810=EDGE_LOOP ( 'NONE', ( #4497, #4575, #9698, #12334 ) ) ;
#3811=ORIENTED_EDGE ( 'NONE', *, *, #9817, .T. ) ;
#3813=CARTESIAN_POINT ( 'NONE',  ( -21.53500198183446557, 30.09884447264290941, 59.17606103016743191 ) ) ;
#3815=EDGE_CURVE ( 'NONE', #6126, #898, #805, .T. ) ;
#3817=CARTESIAN_POINT ( 'NONE',  ( -13.40033457972183939, -4.525318844826149878, 63.45000000000000284 ) ) ;
#3818=ADVANCED_FACE ( 'NONE', ( #9130 ), #7344, .T. ) ;
#3819=FACE_OUTER_BOUND ( 'NONE', #9545, .T. ) ;
#3827=CIRCLE ( 'NONE', #2726, 17.66282263685195275 ) ;
#3831=AXIS2_PLACEMENT_3D ( 'NONE', #6585, #10860, #12944 ) ;
#3832=ORIENTED_EDGE ( 'NONE', *, *, #13306, .T. ) ;
#3833=LINE ( 'NONE', #5067, #11836 ) ;
#3834=DIRECTION ( 'NONE',  ( 1.000000000000000000, 0.000000000000000000, 0.000000000000000000 ) ) ;
#3835=DIRECTION ( 'NONE',  ( 0.000000000000000000, 0.000000000000000000, 1.000000000000000000 ) ) ;
#3836=CARTESIAN_POINT ( 'NONE',  ( -36.05918829505000645, 10.97290950744599947, 63.54999999999999716 ) ) ;
#3838=DIRECTION ( 'NONE',  ( -1.000000000000000000, 0.000000000000000000, 0.000000000000000000 ) ) ;
#3841=EDGE_CURVE ( 'NONE', #194, #2105, #10282, .T. ) ;
#3842=FACE_BOUND ( 'NONE', #4628, .T. ) ;
#3846=CIRCLE ( 'NONE', #12059, 0.9499999999999995115 ) ;
#3847=EDGE_CURVE ( 'NONE', #4952, #1042, #2658, .T. ) ;
#3849=ORIENTED_EDGE ( 'NONE', *, *, #5686, .F. ) ;
#3850=DIRECTION ( 'NONE',  ( 0.000000000000000000, 0.000000000000000000, 1.000000000000000000 ) ) ;
#3851=ORIENTED_EDGE ( 'NONE', *, *, #9817, .F. ) ;
#3852=DIRECTION ( 'NONE',  ( -1.000000000000000000, 0.000000000000000000, 0.000000000000000000 ) ) ;
#3853=VECTOR ( 'NONE', #12690, 1000.000000000000000 ) ;
#3854=CARTESIAN_POINT ( 'NONE',  ( -7.241070169793063727, -7.867426463707971607, 17.25000000000000000 ) ) ;
#3856=EDGE_CURVE ( 'NONE', #10151, #1164, #8033, .T. ) ;
#3857=DIRECTION ( 'NONE',  ( 0.000000000000000000, 0.000000000000000000, -1.000000000000000000 ) ) ;
#3858=CYLINDRICAL_SURFACE ( 'NONE', #9145, 2.700000000000000178 ) ;
#3859=DIRECTION ( 'NONE',  ( 0.6615960714621567096, -0.7498604124941127269, 0.000000000000000000 ) ) ;
#3860=EDGE_CURVE ( 'NONE', #5017, #3252, #3833, .T. ) ;
#3861=AXIS2_PLACEMENT_3D ( 'NONE', #10368, #727, #12265 ) ;
#3863=EDGE_LOOP ( 'NONE', ( #3438, #2485, #13202, #6991 ) ) ;
#3864=CARTESIAN_POINT ( 'NONE',  ( -15.88770235650742002, 30.25856101889280225, 60.93332845326816027 ) ) ;
#3868=CARTESIAN_POINT ( 'NONE',  ( -18.05918829358019906, 3.806800778008990083, 61.72253826514069885 ) ) ;
#3870=CARTESIAN_POINT ( 'NONE',  ( -33.29928216905001648, 3.352862570445993562, 61.63595870799996845 ) ) ;
#3871=FACE_OUTER_BOUND ( 'NONE', #12511, .T. ) ;
#3872=VERTEX_POINT ( 'NONE', #8080 ) ;
#3874=VECTOR ( 'NONE', #2327, 1000.000000000000114 ) ;
#3875=CARTESIAN_POINT ( 'NONE',  ( -25.86749127492454647, -8.860076549334127805, 17.25000000000000000 ) ) ;
#3877=DIRECTION ( 'NONE',  ( -0.000000000000000000, -0.000000000000000000, 1.000000000000000000 ) ) ;
#3878=ORIENTED_EDGE ( 'NONE', *, *, #13017, .T. ) ;
#3879=AXIS2_PLACEMENT_3D ( 'NONE', #12214, #13116, #10979 ) ;
#3880=ORIENTED_EDGE ( 'NONE', *, *, #10237, .T. ) ;
#3881=ADVANCED_FACE ( 'NONE', ( #8214 ), #1588, .T. ) ;
#3885=CARTESIAN_POINT ( 'NONE',  ( -19.81655147050198451, 30.29372715545316908, 61.21836758686404067 ) ) ;
#3892=ORIENTED_EDGE ( 'NONE', *, *, #4255, .F. ) ;
#3893=EDGE_CURVE ( 'NONE', #898, #13375, #5967, .T. ) ;
#3894=VERTEX_POINT ( 'NONE', #742 ) ;
#3896=DIRECTION ( 'NONE',  ( 0.9496839325805427334, 0.3132098788326367345, 0.000000000000000000 ) ) ;
#3898=CARTESIAN_POINT ( 'NONE',  ( -18.05918829504999934, 10.97290950744599947, 60.04999999999999716 ) ) ;
#3899=DIRECTION ( 'NONE',  ( 0.000000000000000000, 0.000000000000000000, 1.000000000000000000 ) ) ;
#3900=DIRECTION ( 'NONE',  ( 0.000000000000000000, 0.000000000000000000, -1.000000000000000000 ) ) ;
#3903=CARTESIAN_POINT ( 'NONE',  ( -36.21615338608749823, 23.36596564213564875, 68.85549045786049760 ) ) ;
#3905=DIRECTION ( 'NONE',  ( 0.000000000000000000, 0.000000000000000000, 1.000000000000000000 ) ) ;
#3907=CARTESIAN_POINT ( 'NONE',  ( -18.05918829504999934, 10.97290950744599947, 64.85000000000000853 ) ) ;
#3910=EDGE_CURVE ( 'NONE', #11645, #7929, #9838, .T. ) ;
#3911=ORIENTED_EDGE ( 'NONE', *, *, #11943, .T. ) ;
#3914=ORIENTED_EDGE ( 'NONE', *, *, #3213, .F. ) ;
#3917=DIRECTION ( 'NONE',  ( -0.9496839325805416232, -0.3132098788326400096, 0.000000000000000000 ) ) ;
#3918=ADVANCED_FACE ( 'NONE', ( #5001 ), #11610, .F. ) ;
#3919=AXIS2_PLACEMENT_3D ( 'NONE', #10082, #697, #3859 ) ;
#3921=FACE_OUTER_BOUND ( 'NONE', #9301, .T. ) ;
#3923=VERTEX_POINT ( 'NONE', #12479 ) ;
#3924=ADVANCED_FACE ( 'NONE', ( #9053 ), #11153, .T. ) ;
#3925=CIRCLE ( 'NONE', #13061, 4.750000000000000888 ) ;
#3927=CARTESIAN_POINT ( 'NONE',  ( -15.26929014322137945, 30.19213140065401646, 60.32611073319715445 ) ) ;
#3929=ORIENTED_EDGE ( 'NONE', *, *, #6306, .F. ) ;
#3931=DIRECTION ( 'NONE',  ( 0.000000000000000000, 0.000000000000000000, -1.000000000000000000 ) ) ;
#3932=ORIENTED_EDGE ( 'NONE', *, *, #13287, .T. ) ;
#3933=CARTESIAN_POINT ( 'NONE',  ( -18.05918829504999934, 7.130333642789880244, 17.25000000000000000 ) ) ;
#3934=DIRECTION ( 'NONE',  ( -1.000000000000000000, 0.000000000000000000, 0.000000000000000000 ) ) ;
#3935=EDGE_CURVE ( 'NONE', #10398, #11868, #6888, .T. ) ;
#3936=LINE ( 'NONE', #12327, #10725 ) ;
#3937=DIRECTION ( 'NONE',  ( 0.000000000000000000, 0.000000000000000000, 1.000000000000000000 ) ) ;
#3938=DIRECTION ( 'NONE',  ( 0.4528443260392607250, 0.8915896008669278450, 0.000000000000000000 ) ) ;
#3940=LINE ( 'NONE', #520, #11838 ) ;
#3942=ORIENTED_EDGE ( 'NONE', *, *, #5729, .T. ) ;
#3943=AXIS2_PLACEMENT_3D ( 'NONE', #12017, #9866, #9713 ) ;
#3945=ORIENTED_EDGE ( 'NONE', *, *, #847, .F. ) ;
#3946=ORIENTED_EDGE ( 'NONE', *, *, #12646, .T. ) ;
#3955=ORIENTED_EDGE ( 'NONE', *, *, #1329, .T. ) ;
#3956=ORIENTED_EDGE ( 'NONE', *, *, #3856, .F. ) ;
#3958=CARTESIAN_POINT ( 'NONE',  ( -16.07440008066354764, 8.723328269963658954, 24.10000000000000142 ) ) ;
#3959=ORIENTED_EDGE ( 'NONE', *, *, #5440, .T. ) ;
#3960=DIRECTION ( 'NONE',  ( 0.000000000000000000, 0.000000000000000000, 1.000000000000000000 ) ) ;
#3963=CARTESIAN_POINT ( 'NONE',  ( -18.05918829504999934, 10.97290950744599947, 5.250000000000000000 ) ) ;
#3965=DIRECTION ( 'NONE',  ( -1.000000000000000000, -2.649577643422789356E-15, 0.000000000000000000 ) ) ;
#3966=DIRECTION ( 'NONE',  ( -1.000000000000000000, 0.000000000000000000, 0.000000000000000000 ) ) ;
#3968=FACE_BOUND ( 'NONE', #13406, .T. ) ;
#3969=EDGE_CURVE ( 'NONE', #7909, #5579, #1576, .T. ) ;
#3971=AXIS2_PLACEMENT_3D ( 'NONE', #8030, #2758, #11257 ) ;
#3972=VECTOR ( 'NONE', #12741, 1000.000000000000000 ) ;
#3973=EDGE_CURVE ( 'NONE', #11479, #12033, #3371, .T. ) ;
#3975=ORIENTED_EDGE ( 'NONE', *, *, #10464, .T. ) ;
#3976=VERTEX_POINT ( 'NONE', #40 ) ;
#3978=ORIENTED_EDGE ( 'NONE', *, *, #2016, .F. ) ;
#3979=VERTEX_POINT ( 'NONE', #8488 ) ;
#3982=DIRECTION ( 'NONE',  ( 0.000000000000000000, 0.000000000000000000, 1.000000000000000000 ) ) ;
#3983=VECTOR ( 'NONE', #9644, 1000.000000000000000 ) ;
#3984=AXIS2_PLACEMENT_3D ( 'NONE', #10417, #6220, #845 ) ;
#3985=VECTOR ( 'NONE', #13317, 1000.000000000000000 ) ;
#3987=VECTOR ( 'NONE', #13501, 1000.000000000000114 ) ;
#3988=DIRECTION ( 'NONE',  ( 0.000000000000000000, 0.000000000000000000, -1.000000000000000000 ) ) ;
#3989=CARTESIAN_POINT ( 'NONE',  ( -18.05918829504999934, 14.81548537210212046, 68.85549045786049760 ) ) ;
#3991=EDGE_CURVE ( 'NONE', #9550, #12241, #957, .T. ) ;
#3994=CIRCLE ( 'NONE', #7098, 7.833333332999988130 ) ;
#3995=ORIENTED_EDGE ( 'NONE', *, *, #11318, .T. ) ;
#3996=AXIS2_PLACEMENT_3D ( 'NONE', #9378, #5934, #7970 ) ;
#3997=EDGE_CURVE ( 'NONE', #6107, #9550, #9541, .T. ) ;
#3999=CARTESIAN_POINT ( 'NONE',  ( -15.09142106175067788, 30.16999431241942276, 54.60426940283544184 ) ) ;
#4005=CARTESIAN_POINT ( 'NONE',  ( -18.05918829504999934, 10.97290950744599947, 62.85000000000000142 ) ) ;
#4007=ORIENTED_EDGE ( 'NONE', *, *, #5747, .F. ) ;
#4008=DIRECTION ( 'NONE',  ( 0.000000000000000000, 0.000000000000000000, -1.000000000000000000 ) ) ;
#4010=DIRECTION ( 'NONE',  ( -1.000000000000000000, 0.000000000000000000, 0.000000000000000000 ) ) ;
#4013=AXIS2_PLACEMENT_3D ( 'NONE', #4213, #4288, #8531 ) ;
#4015=ORIENTED_EDGE ( 'NONE', *, *, #2127, .T. ) ;
#4019=EDGE_LOOP ( 'NONE', ( #4370, #13382 ) ) ;
#4020=AXIS2_PLACEMENT_3D ( 'NONE', #1423, #10099, #8051 ) ;
#4021=AXIS2_PLACEMENT_3D ( 'NONE', #176, #7428, #7364 ) ;
#4024=CARTESIAN_POINT ( 'NONE',  ( -20.36713024065852551, 30.24535125755222609, 60.82066359492309005 ) ) ;
#4025=DIRECTION ( 'NONE',  ( 0.000000000000000000, 1.672022627447524993E-15, 1.000000000000000000 ) ) ;
#4026=CARTESIAN_POINT ( 'NONE',  ( -4.284128961655960133, 3.976464670139415070, 60.65000000000000568 ) ) ;
#4029=DIRECTION ( 'NONE',  ( 0.000000000000000000, 0.000000000000000000, -1.000000000000000000 ) ) ;
#4034=CARTESIAN_POINT ( 'NONE',  ( -34.55918829505000645, 10.97290950744599947, 57.35000000000000142 ) ) ;
#4037=DIRECTION ( 'NONE',  ( 0.000000000000000000, 0.000000000000000000, -1.000000000000000000 ) ) ;
#4038=CARTESIAN_POINT ( 'NONE',  ( -34.72201093190195564, 10.97290950744599947, 17.25000000000000000 ) ) ;
#4040=AXIS2_PLACEMENT_3D ( 'NONE', #10321, #13383, #1720 ) ;
#4041=CIRCLE ( 'NONE', #8477, 6.000000000000002665 ) ;
#4042=AXIS2_PLACEMENT_3D ( 'NONE', #13498, #3729, #7976 ) ;
#4043=DIRECTION ( 'NONE',  ( 1.000000000000000000, 0.000000000000000000, 0.000000000000000000 ) ) ;
#4045=CONICAL_SURFACE ( 'NONE', #6251, 3.800000000000001155, 0.7853981633974476129 ) ;
#4046=DIRECTION ( 'NONE',  ( 0.000000000000000000, 0.000000000000000000, -1.000000000000000000 ) ) ;
#4047=CARTESIAN_POINT ( 'NONE',  ( -23.57208814848684852, -7.366404416634599883, 62.14999999999999858 ) ) ;
#4048=CARTESIAN_POINT ( 'NONE',  ( -18.05918829504999934, 10.97290950744599947, 57.54999999999999716 ) ) ;
#4049=PRESENTATION_STYLE_ASSIGNMENT (( #7170 ) ) ;
#4051=ORIENTED_EDGE ( 'NONE', *, *, #2178, .F. ) ;
#4052=AXIS2_PLACEMENT_3D ( 'NONE', #5108, #2903, #13554 ) ;
#4053=CONICAL_SURFACE ( 'NONE', #5142, 6.049999999999999822, 0.1357715569457985105 ) ;
#4054=APPLICATION_CONTEXT ( 'automotive_design' ) ;
#4056=CIRCLE ( 'NONE', #2729, 2.700000000000000178 ) ;
#4058=CARTESIAN_POINT ( 'NONE',  ( -5.789834139046009298, 27.54455229823479812, 7.250000000000000000 ) ) ;
#4060=EDGE_CURVE ( 'NONE', #2748, #3674, #11398, .T. ) ;
#4061=ORIENTED_EDGE ( 'NONE', *, *, #13177, .T. ) ;
#4063=DIRECTION ( 'NONE',  ( 0.000000000000000000, 0.000000000000000000, -1.000000000000000000 ) ) ;
#4064=DIRECTION ( 'NONE',  ( -0.6615960714621565986, 0.7498604124941128379, 0.000000000000000000 ) ) ;
#4068=CIRCLE ( 'NONE', #9406, 4.750000000000000000 ) ;
#4069=LINE ( 'NONE', #12578, #13771 ) ;
#4072=( GEOMETRIC_REPRESENTATION_CONTEXT ( 3 ) GLOBAL_UNCERTAINTY_ASSIGNED_CONTEXT ( ( #10614 ) ) GLOBAL_UNIT_ASSIGNED_CONTEXT ( ( #5489, #9807, #11787 ) ) REPRESENTATION_CONTEXT ( 'NONE', 'WORKASPACE' ) );
#4073=CARTESIAN_POINT ( 'NONE',  ( -14.22962324644737286, 30.04243591129733559, 57.08230891415405495 ) ) ;
#4074=ORIENTED_EDGE ( 'NONE', *, *, #1770, .T. ) ;
#4075=EDGE_CURVE ( 'NONE', #7400, #5675, #3137, .T. ) ;
#4076=ORIENTED_EDGE ( 'NONE', *, *, #7438, .T. ) ;
#4078=DIRECTION ( 'NONE',  ( 0.000000000000000000, 0.000000000000000000, -1.000000000000000000 ) ) ;
#4079=VERTEX_POINT ( 'NONE', #2088 ) ;
#4081=CARTESIAN_POINT ( 'NONE',  ( -19.71317847370539766, 12.84756053868127879, 67.84999999999999432 ) ) ;
#4083=DIRECTION ( 'NONE',  ( 0.000000000000000000, 0.000000000000000000, 1.000000000000000000 ) ) ;
#4084=DIRECTION ( 'NONE',  ( 0.000000000000000000, 0.000000000000000000, -1.000000000000000000 ) ) ;
#4086=CYLINDRICAL_SURFACE ( 'NONE', #6925, 34.70000000000000284 ) ;
#4089=ORIENTED_EDGE ( 'NONE', *, *, #8957, .T. ) ;
#4091=ORIENTED_EDGE ( 'NONE', *, *, #1329, .F. ) ;
#4092=AXIS2_PLACEMENT_3D ( 'NONE', #8275, #2787, #6096 ) ;
#4094=CARTESIAN_POINT ( 'NONE',  ( -18.05918829504999934, 10.97290950744599947, 63.35000000000000142 ) ) ;
#4095=CARTESIAN_POINT ( 'NONE',  ( -18.87229898793585292, 30.34604302011655363, 61.60856125853900522 ) ) ;
#4097=CARTESIAN_POINT ( 'NONE',  ( -18.05918829504999934, 10.97290950744599947, 60.04999999999999716 ) ) ;
#4099=EDGE_CURVE ( 'NONE', #2443, #4079, #8953, .T. ) ;
#4104=AXIS2_PLACEMENT_3D ( 'NONE', #5880, #10159, #4841 ) ;
#4105=ADVANCED_FACE ( 'NONE', ( #5803 ), #6990, .T. ) ;
#4112=CARTESIAN_POINT ( 'NONE',  ( -18.05918829504999934, 10.97290950744599947, 27.09999999999999787 ) ) ;
#4113=CARTESIAN_POINT ( 'NONE',  ( -18.05918829504999934, 10.97290950744599947, 61.65955166399999854 ) ) ;
#4114=VERTEX_POINT ( 'NONE', #6926 ) ;
#4116=DIRECTION ( 'NONE',  ( 0.000000000000000000, 0.000000000000000000, -1.000000000000000000 ) ) ;
#4118=EDGE_CURVE ( 'NONE', #2746, #3005, #8491, .T. ) ;
#4119=DIRECTION ( 'NONE',  ( 1.000000000000000000, 0.000000000000000000, 0.000000000000000000 ) ) ;
#4121=ORIENTED_EDGE ( 'NONE', *, *, #6752, .F. ) ;
#4122=ORIENTED_EDGE ( 'NONE', *, *, #6634, .T. ) ;
#4123=DIRECTION ( 'NONE',  ( 0.000000000000000000, 0.000000000000000000, 1.000000000000000000 ) ) ;
#4126=CARTESIAN_POINT ( 'NONE',  ( -20.10273234482015425, 15.83781399370707810, 68.57331103393035221 ) ) ;
#4129=DIRECTION ( 'NONE',  ( 0.000000000000000000, 0.000000000000000000, -1.000000000000000000 ) ) ;
#4130=ADVANCED_FACE ( 'NONE', ( #4775 ), #252, .F. ) ;
#4132=CARTESIAN_POINT ( 'NONE',  ( -15.27375731803826397, 30.19267137862248163, 60.33151965850841236 ) ) ;
#4134=ORIENTED_EDGE ( 'NONE', *, *, #10568, .F. ) ;
#4135=CARTESIAN_POINT ( 'NONE',  ( -18.05918829504999934, 3.354823934416959919, 61.65955166408550525 ) ) ;
#4136=CIRCLE ( 'NONE', #12391, 4.000000000000000888 ) ;
#4138=CARTESIAN_POINT ( 'NONE',  ( -20.37477454516755060, 13.59742095117539940, 68.84999999999999432 ) ) ;
#4139=EDGE_LOOP ( 'NONE', ( #3239, #1181, #8565 ) ) ;
#4141=CARTESIAN_POINT ( 'NONE',  ( -35.05918829505000645, 27.97290950744599769, 17.25000000000000000 ) ) ;
#4142=FACE_OUTER_BOUND ( 'NONE', #4149, .T. ) ;
#4143=DIRECTION ( 'NONE',  ( 0.4528443260392608916, 0.8915896008669277339, 0.000000000000000000 ) ) ;
#4144=DIRECTION ( 'NONE',  ( 0.000000000000000000, 0.000000000000000000, -1.000000000000000000 ) ) ;
#4145=EDGE_CURVE ( 'NONE', #6343, #2296, #914, .T. ) ;
#4146=ADVANCED_FACE ( 'NONE', ( #11916 ), #13025, .T. ) ;
#4147=ORIENTED_EDGE ( 'NONE', *, *, #8220, .F. ) ;
#4148=ORIENTED_EDGE ( 'NONE', *, *, #5670, .F. ) ;
#4149=EDGE_LOOP ( 'NONE', ( #9955, #5235, #5665, #2283 ) ) ;
#4154=ORIENTED_EDGE ( 'NONE', *, *, #3008, .F. ) ;
#4155=VECTOR ( 'NONE', #2587, 1000.000000000000114 ) ;
#4157=CARTESIAN_POINT ( 'NONE',  ( -18.78165555769320960, 26.95724247477075153, 56.02363196900555664 ) ) ;
#4160=CARTESIAN_POINT ( 'NONE',  ( -1.059188295049996231, 27.97290950744599769, 7.250000000000000000 ) ) ;
#4163=EDGE_CURVE ( 'NONE', #10962, #13429, #2300, .T. ) ;
#4164=CIRCLE ( 'NONE', #5262, 6.419999999999999929 ) ;
#4169=CARTESIAN_POINT ( 'NONE',  ( -1.059188295049996231, 10.97290950744599947, 57.35000000000000142 ) ) ;
#4171=DIRECTION ( 'NONE',  ( 0.000000000000000000, 0.000000000000000000, -1.000000000000000000 ) ) ;
#4174=CARTESIAN_POINT ( 'NONE',  ( -11.91335496205000055, 10.97290950744599947, 61.10999999999999943 ) ) ;
#4178=AXIS2_PLACEMENT_3D ( 'NONE', #10473, #9492, #9700 ) ;
#4180=EDGE_CURVE ( 'NONE', #11456, #1687, #10222, .T. ) ;
#4181=ORIENTED_EDGE ( 'NONE', *, *, #7644, .F. ) ;
#4184=AXIS2_PLACEMENT_3D ( 'NONE', #1800, #10322, #743 ) ;
#4185=EDGE_CURVE ( 'NONE', #10997, #467, #9161, .T. ) ;
#4187=ORIENTED_EDGE ( 'NONE', *, *, #4163, .T. ) ;
#4190=CARTESIAN_POINT ( 'NONE',  ( -20.08917107840481009, 15.84977899470587559, 68.56751079857853881 ) ) ;
#4191=ORIENTED_EDGE ( 'NONE', *, *, #12377, .T. ) ;
#4192=DIRECTION ( 'NONE',  ( 0.000000000000000000, 0.000000000000000000, 1.000000000000000000 ) ) ;
#4197=VECTOR ( 'NONE', #10661, 1000.000000000000000 ) ;
#4199=ORIENTED_EDGE ( 'NONE', *, *, #13592, .F. ) ;
#4200=EDGE_CURVE ( 'NONE', #10920, #1852, #705, .T. ) ;
#4201=CARTESIAN_POINT ( 'NONE',  ( -14.79170389260510277, 30.12932847815346094, 55.08659537360541947 ) ) ;
#4203=EDGE_LOOP ( 'NONE', ( #7036, #6742, #13782, #5248 ) ) ;
#4204=CIRCLE ( 'NONE', #1507, 6.000000000000000888 ) ;
#4206=FACE_OUTER_BOUND ( 'NONE', #7374, .T. ) ;
#4207=CIRCLE ( 'NONE', #625, 6.449999999999997513 ) ;
#4208=PLANE ( 'NONE',  #9279 ) ;
#4210=DIRECTION ( 'NONE',  ( 0.000000000000000000, 0.000000000000000000, -1.000000000000000000 ) ) ;
#4213=CARTESIAN_POINT ( 'NONE',  ( -1.059188295049996231, 27.97290950744599769, 64.85000000000000853 ) ) ;
#4216=CIRCLE ( 'NONE', #12018, 17.50000000000000355 ) ;
#4217=VERTEX_POINT ( 'NONE', #8178 ) ;
#4218=ORIENTED_EDGE ( 'NONE', *, *, #4853, .F. ) ;
#4222=EDGE_CURVE ( 'NONE', #10012, #12272, #2721, .T. ) ;
#4224=DIRECTION ( 'NONE',  ( 0.6615960714621574867, -0.7498604124941119498, 0.000000000000000000 ) ) ;
#4225=EDGE_CURVE ( 'NONE', #11449, #7400, #5155, .T. ) ;
#4227=AXIS2_PLACEMENT_3D ( 'NONE', #6395, #8494, #12761 ) ;
#4231=DIRECTION ( 'NONE',  ( 0.000000000000000000, 0.000000000000000000, 1.000000000000000000 ) ) ;
#4232=CARTESIAN_POINT ( 'NONE',  ( -37.75918829505000218, -6.027090492554000534, 58.85000000000000142 ) ) ;
#4236=DIRECTION ( 'NONE',  ( -0.9496839325805428444, -0.3132098788326364569, 0.000000000000000000 ) ) ;
#4237=ORIENTED_EDGE ( 'NONE', *, *, #3935, .T. ) ;
#4238=CARTESIAN_POINT ( 'NONE',  ( -18.05918829504999934, 28.64232754551664684, 55.84999999999999432 ) ) ;
#4242=CARTESIAN_POINT ( 'NONE',  ( -19.55384571722024489, 30.31214524169468660, 53.34041679414971782 ) ) ;
#4243=DIRECTION ( 'NONE',  ( 0.000000000000000000, 0.000000000000000000, -1.000000000000000000 ) ) ;
#4244=CYLINDRICAL_SURFACE ( 'NONE', #4227, 6.450000000000001066 ) ;
#4245=ADVANCED_FACE ( 'NONE', ( #1981 ), #8324, .F. ) ;
#4247=PLANE ( 'NONE',  #12737 ) ;
#4249=DIRECTION ( 'NONE',  ( 0.7071067811865474617, 0.000000000000000000, 0.7071067811865474617 ) ) ;
#4250=AXIS2_PLACEMENT_3D ( 'NONE', #5764, #8993, #474 ) ;
#4252=SHAPE_REPRESENTATION_RELATIONSHIP ( 'NONE' , 'NONE' ,  #13195, #8750 ) ;
#4255=EDGE_CURVE ( 'NONE', #8825, #12804, #10503, .T. ) ;
#4256=ORIENTED_EDGE ( 'NONE', *, *, #1488, .T. ) ;
#4257=ORIENTED_EDGE ( 'NONE', *, *, #9679, .T. ) ;
#4259=DIRECTION ( 'NONE',  ( 0.000000000000000000, 0.000000000000000000, -1.000000000000000000 ) ) ;
#4260=CIRCLE ( 'NONE', #2939, 34.69999999999999574 ) ;
#4262=VECTOR ( 'NONE', #7724, 1000.000000000000227 ) ;
#4263=EDGE_LOOP ( 'NONE', ( #1856, #13471, #10481, #6404 ) ) ;
#4264=ORIENTED_EDGE ( 'NONE', *, *, #130, .F. ) ;
#4265=ADVANCED_FACE ( 'NONE', ( #8118 ), #10415, .F. ) ;
#4266=CARTESIAN_POINT ( 'NONE',  ( -14.33236984630097588, 7.593145069921623858, 68.84999999999999432 ) ) ;
#4267=CARTESIAN_POINT ( 'NONE',  ( -1.059188295049996231, -6.027090492554000534, 17.25000000000000000 ) ) ;
#4269=CARTESIAN_POINT ( 'NONE',  ( -17.23821357112329977, 5.029341513162310484, 67.84999999999999432 ) ) ;
#4270=FACE_OUTER_BOUND ( 'NONE', #12951, .T. ) ;
#4274=AXIS2_PLACEMENT_3D ( 'NONE', #10193, #7938, #7026 ) ;
#4276=CARTESIAN_POINT ( 'NONE',  ( -15.51133711870873455, 30.22015921542349304, 54.10466577694464263 ) ) ;
#4277=ORIENTED_EDGE ( 'NONE', *, *, #9228, .F. ) ;
#4278=VERTEX_POINT ( 'NONE', #4138 ) ;
#4279=EDGE_CURVE ( 'NONE', #3112, #6060, #6712, .T. ) ;
#4280=DIRECTION ( 'NONE',  ( 1.000000000000000000, 0.000000000000000000, 0.000000000000000000 ) ) ;
#4281=AXIS2_PLACEMENT_3D ( 'NONE', #4112, #12557, #807 ) ;
#4282=FACE_OUTER_BOUND ( 'NONE', #13057, .T. ) ;
#4283=AXIS2_PLACEMENT_3D ( 'NONE', #5257, #8611, #3258 ) ;
#4285=CARTESIAN_POINT ( 'NONE',  ( -30.48673169511680214, 10.97290950744599947, 83.57661607529820458 ) ) ;
#4286=CARTESIAN_POINT ( 'NONE',  ( -24.37001676333060018, -4.028726038184999858, 62.14999999999999858 ) ) ;
#4287=ADVANCED_FACE ( 'NONE', ( #12518 ), #11331, .T. ) ;
#4288=DIRECTION ( 'NONE',  ( 0.000000000000000000, 0.000000000000000000, 1.000000000000000000 ) ) ;
#4290=ORIENTED_EDGE ( 'NONE', *, *, #3319, .F. ) ;
#4293=ORIENTED_EDGE ( 'NONE', *, *, #8878, .F. ) ;
#4294=CYLINDRICAL_SURFACE ( 'NONE', #5013, 6.145833333000002341 ) ;
#4295=ORIENTED_EDGE ( 'NONE', *, *, #11747, .T. ) ;
#4296=ORIENTED_EDGE ( 'NONE', *, *, #13427, .T. ) ;
#4300=DIRECTION ( 'NONE',  ( 0.000000000000000000, 0.000000000000000000, 1.000000000000000000 ) ) ;
#4302=DIRECTION ( 'NONE',  ( 0.000000000000000000, 0.000000000000000000, -1.000000000000000000 ) ) ;
#4304=CARTESIAN_POINT ( 'NONE',  ( -36.21615338608749823, -1.420146627243662030, 7.250000000000000000 ) ) ;
#4307=VERTEX_POINT ( 'NONE', #10561 ) ;
#4310=ORIENTED_EDGE ( 'NONE', *, *, #5440, .F. ) ;
#4311=CARTESIAN_POINT ( 'NONE',  ( -18.05918829504999934, 10.97290950744599947, 57.35000000000000142 ) ) ;
#4315=CARTESIAN_POINT ( 'NONE',  ( -18.79031867479901408, 30.34876749365192339, 53.07200068921699909 ) ) ;
#4318=CARTESIAN_POINT ( 'NONE',  ( -38.38077571930825371, -0.4981161769137670281, 5.250000000000000000 ) ) ;
#4324=EDGE_CURVE ( 'NONE', #6154, #8674, #241, .T. ) ;
#4325=VERTEX_POINT ( 'NONE', #12916 ) ;
#4328=ORIENTED_EDGE ( 'NONE', *, *, #4987, .T. ) ;
#4331=CARTESIAN_POINT ( 'NONE',  ( -18.05918829504999934, 10.97290950744599947, 30.59999999999999787 ) ) ;
#4333=CARTESIAN_POINT ( 'NONE',  ( -3.759188295049999518, -6.027090492554000534, 7.250000000000000000 ) ) ;
#4334=DIRECTION ( 'NONE',  ( 0.000000000000000000, 0.000000000000000000, -1.000000000000000000 ) ) ;
#4336=DIRECTION ( 'NONE',  ( 2.612535355386759959E-17, 0.000000000000000000, 1.000000000000000000 ) ) ;
#4337=DIRECTION ( 'NONE',  ( -0.6615960714621565986, 0.7498604124941128379, 0.000000000000000000 ) ) ;
#4343=ORIENTED_EDGE ( 'NONE', *, *, #8576, .F. ) ;
#4346=ADVANCED_FACE ( 'NONE', ( #4282 ), #3178, .T. ) ;
#4348=CARTESIAN_POINT ( 'NONE',  ( -34.05918829504999934, 10.97290950744599947, 64.85000000000000853 ) ) ;
#4350=FACE_OUTER_BOUND ( 'NONE', #1427, .T. ) ;
#4351=CYLINDRICAL_SURFACE ( 'NONE', #10505, 23.22993838181875148 ) ;
#4352=MANIFOLD_SOLID_BREP ( 'NONE', #5065 ) ;
#4356=CARTESIAN_POINT ( 'NONE',  ( -18.05918829504999934, 10.97290950744599947, 118.8499999999999943 ) ) ;
#4358=ORIENTED_EDGE ( 'NONE', *, *, #6716, .T. ) ;
#4360=ADVANCED_FACE ( 'NONE', ( #134 ), #5305, .F. ) ;
#4361=ORIENTED_EDGE ( 'NONE', *, *, #7245, .T. ) ;
#4362=DIRECTION ( 'NONE',  ( 0.000000000000000000, 0.000000000000000000, 1.000000000000000000 ) ) ;
#4365=DIRECTION ( 'NONE',  ( 0.000000000000000000, 0.000000000000000000, -1.000000000000000000 ) ) ;
#4366=CARTESIAN_POINT ( 'NONE',  ( -19.11830548702882737, 26.93836225865674194, 56.28610618890476047 ) ) ;
#4369=CARTESIAN_POINT ( 'NONE',  ( -9.759188295050000406, 10.97290950744599947, 61.86500000000000199 ) ) ;
#4370=ORIENTED_EDGE ( 'NONE', *, *, #2519, .F. ) ;
#4372=CIRCLE ( 'NONE', #123, 6.000000000000000888 ) ;
#4375=DIRECTION ( 'NONE',  ( 0.000000000000000000, 0.000000000000000000, -1.000000000000000000 ) ) ;
#4377=CARTESIAN_POINT ( 'NONE',  ( -19.49808753468298406, 30.31569702816738854, 53.31359561727821017 ) ) ;
#4378=DIRECTION ( 'NONE',  ( -1.000000000000000000, 0.000000000000000000, 0.000000000000000000 ) ) ;
#4379=CARTESIAN_POINT ( 'NONE',  ( -2.842019651049983331, 18.58149382944601058, 61.98378871700000303 ) ) ;
#4383=AXIS2_PLACEMENT_3D ( 'NONE', #12186, #2639, #4578 ) ;
#4385=DIRECTION ( 'NONE',  ( 0.000000000000000000, 0.000000000000000000, -1.000000000000000000 ) ) ;
#4390=CIRCLE ( 'NONE', #5486, 7.166108729582679970 ) ;
#4395=EDGE_CURVE ( 'NONE', #8370, #665, #5505, .T. ) ;
#4396=DIRECTION ( 'NONE',  ( 1.000000000000000000, 0.000000000000000000, 0.000000000000000000 ) ) ;
#4397=FACE_OUTER_BOUND ( 'NONE', #5542, .T. ) ;
#4399=EDGE_CURVE ( 'NONE', #13003, #13286, #8587, .T. ) ;
#4400=EDGE_LOOP ( 'NONE', ( #6215, #12337 ) ) ;
#4401=CARTESIAN_POINT ( 'NONE',  ( -16.49880428525771237, 30.30780693225702294, 53.37335251291963090 ) ) ;
#4402=CARTESIAN_POINT ( 'NONE',  ( -18.05918829504999934, 10.97290950744599947, 5.250000000000000000 ) ) ;
#4404=FILL_AREA_STYLE_COLOUR ( '', #2290 ) ;
#4405=DIRECTION ( 'NONE',  ( -0.9496839325805428444, -0.3132098788326364569, 0.000000000000000000 ) ) ;
#4407=EDGE_CURVE ( 'NONE', #2401, #13684, #11633, .T. ) ;
#4408=AXIS2_PLACEMENT_3D ( 'NONE', #2937, #7162, #11499 ) ;
#4412=EDGE_CURVE ( 'NONE', #6343, #10722, #10696, .T. ) ;
#4418=CIRCLE ( 'NONE', #13566, 1.500000000000001332 ) ;
#4420=ORIENTED_EDGE ( 'NONE', *, *, #11486, .T. ) ;
#4421=ORIENTED_EDGE ( 'NONE', *, *, #8106, .T. ) ;
#4423=DIRECTION ( 'NONE',  ( 0.000000000000000000, 0.000000000000000000, -1.000000000000000000 ) ) ;
#4424=EDGE_CURVE ( 'NONE', #703, #2353, #12530, .T. ) ;
#4426=CIRCLE ( 'NONE', #6198, 6.049999999999999822 ) ;
#4427=CARTESIAN_POINT ( 'NONE',  ( -17.56406670600707187, 26.96510319970443348, 55.93198005405052697 ) ) ;
#4429=DIRECTION ( 'NONE',  ( -0.6615960714621569316, 0.7498604124941123938, 0.000000000000000000 ) ) ;
#4430=AXIS2_PLACEMENT_3D ( 'NONE', #8722, #6350, #7500 ) ;
#4432=AXIS2_PLACEMENT_3D ( 'NONE', #10058, #8932, #13389 ) ;
#4434=LINE ( 'NONE', #4717, #2038 ) ;
#4436=EDGE_CURVE ( 'NONE', #7400, #6357, #10981, .T. ) ;
#4438=ORIENTED_EDGE ( 'NONE', *, *, #3815, .T. ) ;
#4440=AXIS2_PLACEMENT_3D ( 'NONE', #13727, #2028, #6266 ) ;
#4441=EDGE_LOOP ( 'NONE', ( #2750, #8320 ) ) ;
#4442=VECTOR ( 'NONE', #6146, 1000.000000000000000 ) ;
#4443=DIRECTION ( 'NONE',  ( 0.3202092937642124215, 0.6304490528084107925, -0.7071067811865487940 ) ) ;
#4445=CARTESIAN_POINT ( 'NONE',  ( -5.631644894983189431, 10.97290950744599947, 7.250000000000000000 ) ) ;
#4450=CARTESIAN_POINT ( 'NONE',  ( -18.05918829504999934, 18.13068114044600065, 61.70038048199999281 ) ) ;
#4451=DIRECTION ( 'NONE',  ( 0.000000000000000000, 0.000000000000000000, -1.000000000000000000 ) ) ;
#4453=DIRECTION ( 'NONE',  ( 0.000000000000000000, 0.000000000000000000, -1.000000000000000000 ) ) ;
#4455=CONICAL_SURFACE ( 'NONE', #214, 16.95000000000000284, 0.7853981633974447263 ) ;
#4456=EDGE_CURVE ( 'NONE', #8158, #11675, #13636, .T. ) ;
#4461=ORIENTED_EDGE ( 'NONE', *, *, #2344, .F. ) ;
#4465=CIRCLE ( 'NONE', #13377, 0.9499999999999995115 ) ;
#4466=AXIS2_PLACEMENT_3D ( 'NONE', #7921, #6751, #6601 ) ;
#4467=DIRECTION ( 'NONE',  ( 0.000000000000000000, 0.000000000000000000, -1.000000000000000000 ) ) ;
#4468=CARTESIAN_POINT ( 'NONE',  ( -30.30918829504999934, 27.97290950744599769, 68.85549045786049760 ) ) ;
#4470=LINE ( 'NONE', #7588, #1743 ) ;
#4475=ADVANCED_FACE ( 'NONE', ( #12305, #12225 ), #10073, .T. ) ;
#4476=CARTESIAN_POINT ( 'NONE',  ( -15.26283791438578419, 30.19135017472695637, 54.38173404877133521 ) ) ;
#4477=ORIENTED_EDGE ( 'NONE', *, *, #5536, .F. ) ;
#4483=CIRCLE ( 'NONE', #8940, 4.000000000000000888 ) ;
#4484=CIRCLE ( 'NONE', #677, 2.700000000000001066 ) ;
#4485=CYLINDRICAL_SURFACE ( 'NONE', #8682, 0.9499999999999995115 ) ;
#4486=CARTESIAN_POINT ( 'NONE',  ( -38.38077571930825371, -0.4981161769137670281, 17.25000000000000000 ) ) ;
#4489=ADVANCED_FACE ( 'NONE', ( #4694 ), #9870, .T. ) ;
#4492=CARTESIAN_POINT ( 'NONE',  ( -1.059188295049996231, -6.027090492554000534, 7.250000000000000000 ) ) ;
#4494=CIRCLE ( 'NONE', #12312, 5.999999999999997335 ) ;
#4496=VERTEX_POINT ( 'NONE', #291 ) ;
#4497=ORIENTED_EDGE ( 'NONE', *, *, #1394, .T. ) ;
#4498=LINE ( 'NONE', #6728, #1991 ) ;
#4499=LINE ( 'NONE', #13010, #13777 ) ;
#4501=DIRECTION ( 'NONE',  ( -0.4528443260392611136, -0.8915896008669277339, 0.000000000000000000 ) ) ;
#4502=CARTESIAN_POINT ( 'NONE',  ( -17.48907183174917890, 26.96265924644433198, 55.96010560725802918 ) ) ;
#4503=DIRECTION ( 'NONE',  ( -1.000000000000000000, 0.000000000000000000, 0.000000000000000000 ) ) ;
#4504=LINE ( 'NONE', #13016, #8961 ) ;
#4509=ORIENTED_EDGE ( 'NONE', *, *, #4436, .T. ) ;
#4513=AXIS2_PLACEMENT_3D ( 'NONE', #5699, #12209, #7868 ) ;
#4514=DIRECTION ( 'NONE',  ( 0.4528443260392610026, 0.8915896008669278450, 0.000000000000000000 ) ) ;
#4515=CARTESIAN_POINT ( 'NONE',  ( -15.34212233881444831, 16.32244711264754855, 57.35000000000000142 ) ) ;
#4516=CARTESIAN_POINT ( 'NONE',  ( -18.05918829504999934, 10.97290950744599947, 56.84999999999999432 ) ) ;
#4519=CARTESIAN_POINT ( 'NONE',  ( -19.81805515243290472, 30.29381900190004018, 53.48032518229263843 ) ) ;
#4520=( NAMED_UNIT ( * ) PLANE_ANGLE_UNIT ( ) SI_UNIT ( $, .RADIAN. ) );
#4522=CARTESIAN_POINT ( 'NONE',  ( -18.05918829504999934, 3.352862570446000223, 61.63595870800000398 ) ) ;
#4523=CARTESIAN_POINT ( 'NONE',  ( -18.05918829504999934, 10.97290950744599947, 61.86500000000000199 ) ) ;
#4524=DIRECTION ( 'NONE',  ( -1.000000000000000000, 0.000000000000000000, 0.000000000000000000 ) ) ;
#4525=CARTESIAN_POINT ( 'NONE',  ( 3.190811704950004657, -6.027090492554000534, 64.85000000000000853 ) ) ;
#4530=ORIENTED_EDGE ( 'NONE', *, *, #10067, .T. ) ;
#4531=ORIENTED_EDGE ( 'NONE', *, *, #2343, .T. ) ;
#4539=CARTESIAN_POINT ( 'NONE',  ( -4.640588396653431147, -14.07073191448199978, 68.85549045786049760 ) ) ;
#4540=ADVANCED_FACE ( 'NONE', ( #12501 ), #3395, .F. ) ;
#4542=CARTESIAN_POINT ( 'NONE',  ( -5.309188295050000228, -6.027090492554000534, 64.35000000000000853 ) ) ;
#4544=CARTESIAN_POINT ( 'NONE',  ( -18.05918829504999934, 10.97290950744599947, 64.85000000000000853 ) ) ;
#4547=EDGE_LOOP ( 'NONE', ( #13328, #5944, #6642, #6790 ) ) ;
#4548=CARTESIAN_POINT ( 'NONE',  ( -17.15591940245453273, 30.34273348207011622, 53.11510484006901578 ) ) ;
#4551=FACE_OUTER_BOUND ( 'NONE', #6276, .T. ) ;
#4555=EDGE_CURVE ( 'NONE', #1146, #3112, #3827, .T. ) ;
#4558=EDGE_LOOP ( 'NONE', ( #7366, #11473, #7569, #12734 ) ) ;
#4561=ORIENTED_EDGE ( 'NONE', *, *, #6820, .T. ) ;
#4562=VERTEX_POINT ( 'NONE', #3029 ) ;
#4563=VERTEX_POINT ( 'NONE', #13478 ) ;
#4565=CARTESIAN_POINT ( 'NONE',  ( 3.190811704950004657, 27.97290950744599769, 64.35000000000000853 ) ) ;
#4566=EDGE_LOOP ( 'NONE', ( #4076, #11754 ) ) ;
#4567=CARTESIAN_POINT ( 'NONE',  ( -30.32854245105399826, -5.598733283342819611, 64.85000000000000853 ) ) ;
#4569=EDGE_CURVE ( 'NONE', #3894, #2730, #5371, .T. ) ;
#4575=ORIENTED_EDGE ( 'NONE', *, *, #10812, .T. ) ;
#4578=DIRECTION ( 'NONE',  ( 0.4528443260392608916, 0.8915896008669277339, 0.000000000000000000 ) ) ;
#4579=VECTOR ( 'NONE', #5724, 1000.000000000000000 ) ;
#4580=CARTESIAN_POINT ( 'NONE',  ( -21.80975557129390907, 30.05623439618504023, 56.30605713593833173 ) ) ;
#4581=DIRECTION ( 'NONE',  ( -0.7071067811865505703, 8.659560562354931626E-17, 0.7071067811865444641 ) ) ;
#4582=DIRECTION ( 'NONE',  ( -1.000000000000000000, 0.000000000000000000, 0.000000000000000000 ) ) ;
#4583=CARTESIAN_POINT ( 'NONE',  ( -30.32854245105399826, -5.598733283342819611, 68.85549045786049760 ) ) ;
#4584=CARTESIAN_POINT ( 'NONE',  ( -18.05918829504999579, 18.25739707232493103, 61.99499741802014796 ) ) ;
#4585=ADVANCED_FACE ( 'NONE', ( #10277 ), #690, .T. ) ;
#4589=EDGE_CURVE ( 'NONE', #3872, #3046, #265, .T. ) ;
#4591=VECTOR ( 'NONE', #9283, 1000.000000000000000 ) ;
#4592=CARTESIAN_POINT ( 'NONE',  ( -10.25088531517539714, 30.80589556422609832, 83.57661607529820458 ) ) ;
#4594=ORIENTED_EDGE ( 'NONE', *, *, #4685, .T. ) ;
#4596=EDGE_LOOP ( 'NONE', ( #2791, #7136, #2642, #9318 ) ) ;
#4598=DIRECTION ( 'NONE',  ( 0.000000000000000000, 0.000000000000000000, 1.000000000000000000 ) ) ;
#4601=MANIFOLD_SOLID_BREP ( 'NONE', #2135 ) ;
#4602=CARTESIAN_POINT ( 'NONE',  ( -10.47404583389237942, 25.90703532196704728, 58.54999999999999716 ) ) ;
#4604=EDGE_CURVE ( 'NONE', #10154, #318, #10820, .T. ) ;
#4605=CIRCLE ( 'NONE', #7695, 3.500000000000000888 ) ;
#4607=CARTESIAN_POINT ( 'NONE',  ( -1.059188295049996231, -6.027090492554000534, 58.85000000000000142 ) ) ;
#4609=ADVANCED_FACE ( 'NONE', ( #5289, #8640 ), #2248, .T. ) ;
#4610=ORIENTED_EDGE ( 'NONE', *, *, #11933, .T. ) ;
#4611=CIRCLE ( 'NONE', #7046, 6.449999999999997513 ) ;
#4613=CARTESIAN_POINT ( 'NONE',  ( -24.37001676333060018, -4.028726038184999858, 62.14999999999999858 ) ) ;
#4614=EDGE_LOOP ( 'NONE', ( #9688, #8963, #3032, #756 ) ) ;
#4615=ORIENTED_EDGE ( 'NONE', *, *, #3726, .F. ) ;
#4616=CARTESIAN_POINT ( 'NONE',  ( -16.64497473267689998, 26.91028695795525039, 56.84999999999999432 ) ) ;
#4617=DIRECTION ( 'NONE',  ( 0.000000000000000000, 0.000000000000000000, -1.000000000000000000 ) ) ;
#4620=CARTESIAN_POINT ( 'NONE',  ( -10.25088531517542023, -8.860076549334110041, 5.250000000000000000 ) ) ;
#4621=AXIS2_PLACEMENT_3D ( 'NONE', #11803, #12914, #2262 ) ;
#4623=ADVANCED_FACE ( 'NONE', ( #2044 ), #6485, .F. ) ;
#4624=ORIENTED_EDGE ( 'NONE', *, *, #5706, .T. ) ;
#4625=ORIENTED_EDGE ( 'NONE', *, *, #7940, .F. ) ;
#4626=CARTESIAN_POINT ( 'NONE',  ( -17.49469255251400313, 30.35356550733773062, 61.66211139510344452 ) ) ;
#4627=VERTEX_POINT ( 'NONE', #6284 ) ;
#4628=EDGE_LOOP ( 'NONE', ( #1876, #3246 ) ) ;
#4629=STYLED_ITEM ( 'NONE', ( #11094 ), #9410 ) ;
#4632=DIRECTION ( 'NONE',  ( 0.000000000000000000, 0.000000000000000000, 1.000000000000000000 ) ) ;
#4633=ORIENTED_EDGE ( 'NONE', *, *, #12966, .F. ) ;
#4635=CARTESIAN_POINT ( 'NONE',  ( -27.15409092487699994, 0.3335619008453594714, 62.14999999999999858 ) ) ;
#4636=PLANE ( 'NONE',  #5781 ) ;
#4638=VECTOR ( 'NONE', #11220, 1000.000000000000114 ) ;
#4639=AXIS2_PLACEMENT_3D ( 'NONE', #173, #1220, #9689 ) ;
#4641=EDGE_LOOP ( 'NONE', ( #6738, #116, #2433, #741 ) ) ;
#4642=ORIENTED_EDGE ( 'NONE', *, *, #4456, .F. ) ;
#4644=ORIENTED_EDGE ( 'NONE', *, *, #4953, .F. ) ;
#4648=DIRECTION ( 'NONE',  ( 0.000000000000000000, 0.000000000000000000, -1.000000000000000000 ) ) ;
#4649=AXIS2_PLACEMENT_3D ( 'NONE', #1455, #1597, #10132 ) ;
#4650=CIRCLE ( 'NONE', #7747, 16.72262947720610171 ) ;
#4651=VERTEX_POINT ( 'NONE', #9495 ) ;
#4652=CARTESIAN_POINT ( 'NONE',  ( -37.75918829505000218, 27.97290950744599769, 64.85000000000000853 ) ) ;
#4654=CARTESIAN_POINT ( 'NONE',  ( -21.35558781198856337, 30.12521254561496775, 59.55915808916093113 ) ) ;
#4655=DIRECTION ( 'NONE',  ( -0.6615960714621569316, 0.7498604124941125049, 0.000000000000000000 ) ) ;
#4656=DIRECTION ( 'NONE',  ( 0.000000000000000000, 0.000000000000000000, -1.000000000000000000 ) ) ;
#4657=DIRECTION ( 'NONE',  ( 0.000000000000000000, 0.000000000000000000, -1.000000000000000000 ) ) ;
#4659=CARTESIAN_POINT ( 'NONE',  ( -18.05918829504999934, 10.97290950744599947, 64.85000000000000853 ) ) ;
#4664=CIRCLE ( 'NONE', #4440, 4.250000000000000000 ) ;
#4666=ORIENTED_EDGE ( 'NONE', *, *, #12732, .F. ) ;
#4669=CARTESIAN_POINT ( 'NONE',  ( -18.05918829504999934, 10.97290950744599947, 63.64999999999999858 ) ) ;
#4670=EDGE_CURVE ( 'NONE', #6829, #9069, #943, .T. ) ;
#4677=CARTESIAN_POINT ( 'NONE',  ( -35.05918829505000645, 10.97290950744599947, 57.35000000000000142 ) ) ;
#4678=CARTESIAN_POINT ( 'NONE',  ( -35.05918829505000645, -6.027090492554000534, 64.35000000000000853 ) ) ;
#4684=ORIENTED_EDGE ( 'NONE', *, *, #10549, .T. ) ;
#4685=EDGE_CURVE ( 'NONE', #10154, #5017, #1236, .T. ) ;
#4687=AXIS2_PLACEMENT_3D ( 'NONE', #9527, #10719, #7411 ) ;
#4689=CARTESIAN_POINT ( 'NONE',  ( -18.05918829504999934, 10.97290950744599947, 62.14999999999999858 ) ) ;
#4690=CIRCLE ( 'NONE', #5331, 34.69999999999999574 ) ;
#4691=EDGE_LOOP ( 'NONE', ( #7048, #788, #13802, #13735, #10900 ) ) ;
#4692=CARTESIAN_POINT ( 'NONE',  ( -18.05918829504999934, 10.97290950744599947, 64.85000000000000853 ) ) ;
#4694=FACE_OUTER_BOUND ( 'NONE', #3188, .T. ) ;
#4695=PLANE ( 'NONE',  #8666 ) ;
#4702=ORIENTED_EDGE ( 'NONE', *, *, #2361, .T. ) ;
#4703=CARTESIAN_POINT ( 'NONE',  ( -18.05918829504999934, 10.97290950744599947, 27.30000000000000071 ) ) ;
#4705=ORIENTED_EDGE ( 'NONE', *, *, #5867, .F. ) ;
#4706=CONICAL_SURFACE ( 'NONE', #10723, 16.75000000000000355, 0.7853981633974461696 ) ;
#4709=VECTOR ( 'NONE', #1405, 1000.000000000000000 ) ;
#4711=CARTESIAN_POINT ( 'NONE',  ( -30.80918829504999934, -6.027090492554000534, 64.35000000000000853 ) ) ;
#4712=LINE ( 'NONE', #1269, #7295 ) ;
#4715=DIRECTION ( 'NONE',  ( 0.000000000000000000, 0.000000000000000000, -1.000000000000000000 ) ) ;
#4716=LINE ( 'NONE', #12527, #13364 ) ;
#4717=CARTESIAN_POINT ( 'NONE',  ( 1.640811704950000172, -6.027090492554000534, 64.85000000000000853 ) ) ;
#4718=CIRCLE ( 'NONE', #9850, 16.66282263685194920 ) ;
#4719=ORIENTED_EDGE ( 'NONE', *, *, #6603, .T. ) ;
#4720=CIRCLE ( 'NONE', #11620, 18.00000000000000000 ) ;
#4721=ORIENTED_EDGE ( 'NONE', *, *, #13638, .T. ) ;
#4722=ORIENTED_EDGE ( 'NONE', *, *, #5194, .T. ) ;
#4725=CARTESIAN_POINT ( 'NONE',  ( -21.63433128315409348, 30.08351321291810621, 58.90474581060517067 ) ) ;
#4727=AXIS2_PLACEMENT_3D ( 'NONE', #5125, #9399, #4991 ) ;
#4728=PRESENTATION_STYLE_ASSIGNMENT (( #5621 ) ) ;
#4729=PLANE ( 'NONE',  #7773 ) ;
#4731=CARTESIAN_POINT ( 'NONE',  ( -18.05918829358019906, 3.806800778008990083, 61.72253826514069885 ) ) ;
#4732=CARTESIAN_POINT ( 'NONE',  ( -35.05918829505000645, 27.97290950744599769, 64.85000000000000853 ) ) ;
#4733=DIRECTION ( 'NONE',  ( 0.000000000000000000, 0.000000000000000000, 1.000000000000000000 ) ) ;
#4734=ADVANCED_FACE ( 'NONE', ( #2391 ), #11640, .T. ) ;
#4735=AXIS2_PLACEMENT_3D ( 'NONE', #4539, #3427, #340 ) ;
#4738=FACE_BOUND ( 'NONE', #9437, .T. ) ;
#4739=ORIENTED_EDGE ( 'NONE', *, *, #9499, .F. ) ;
#4741=DIRECTION ( 'NONE',  ( 1.000000000000000000, 0.000000000000000000, 0.000000000000000000 ) ) ;
#4742=DIRECTION ( 'NONE',  ( 0.000000000000000000, 0.000000000000000000, -1.000000000000000000 ) ) ;
#4743=DIRECTION ( 'NONE',  ( 0.000000000000000000, 0.000000000000000000, -1.000000000000000000 ) ) ;
#4744=DIRECTION ( 'NONE',  ( 0.000000000000000000, 0.000000000000000000, 1.000000000000000000 ) ) ;
#4745=CARTESIAN_POINT ( 'NONE',  ( -12.87735031270726083, -6.265087914666309210, 62.14999999999999858 ) ) ;
#4746=LINE ( 'NONE', #3568, #3539 ) ;
#4748=AXIS2_PLACEMENT_3D ( 'NONE', #13589, #8295, #4043 ) ;
#4752=ORIENTED_EDGE ( 'NONE', *, *, #9264, .F. ) ;
#4753=EDGE_LOOP ( 'NONE', ( #13039, #3467 ) ) ;
#4754=CARTESIAN_POINT ( 'NONE',  ( -3.759188295049999518, 27.97290950744599769, 7.250000000000000000 ) ) ;
#4757=CARTESIAN_POINT ( 'NONE',  ( -5.309188295050000228, 27.97290950744599769, 64.35000000000000853 ) ) ;
#4759=CARTESIAN_POINT ( 'NONE',  ( -18.05918829504999934, 10.97290950744599947, 58.54999999999999716 ) ) ;
#4760=CARTESIAN_POINT ( 'NONE',  ( -13.16523020061520022, -5.307421391215619622, 62.14999999999999858 ) ) ;
#4766=EDGE_CURVE ( 'NONE', #6439, #12616, #2297, .T. ) ;
#4767=ORIENTED_EDGE ( 'NONE', *, *, #7843, .F. ) ;
#4769=CARTESIAN_POINT ( 'NONE',  ( -18.05918829504999934, 10.97290950744599947, 63.14999999999999858 ) ) ;
#4771=ORIENTED_EDGE ( 'NONE', *, *, #9115, .F. ) ;
#4774=ORIENTED_EDGE ( 'NONE', *, *, #10824, .F. ) ;
#4775=FACE_OUTER_BOUND ( 'NONE', #13295, .T. ) ;
#4776=CARTESIAN_POINT ( 'NONE',  ( -33.29928216905001648, 18.59295644444599915, 61.63595870799996845 ) ) ;
#4777=DIRECTION ( 'NONE',  ( 1.000000000000000000, 0.000000000000000000, 0.000000000000000000 ) ) ;
#4778=ORIENTED_EDGE ( 'NONE', *, *, #8616, .T. ) ;
#4780=FACE_OUTER_BOUND ( 'NONE', #84, .T. ) ;
#4781=CARTESIAN_POINT ( 'NONE',  ( -25.29804148384604900, -2.574630058508220021, 63.45000000000000284 ) ) ;
#4783=DIRECTION ( 'NONE',  ( -1.000000000000000000, 0.000000000000000000, 0.000000000000000000 ) ) ;
#4784=EDGE_CURVE ( 'NONE', #10025, #10920, #10307, .T. ) ;
#4785=DIRECTION ( 'NONE',  ( -0.9496839325805417342, -0.3132098788326399541, 0.000000000000000000 ) ) ;
#4786=ORIENTED_EDGE ( 'NONE', *, *, #5831, .T. ) ;
#4787=DIRECTION ( 'NONE',  ( -0.6615960714621569316, 0.7498604124941123938, 0.000000000000000000 ) ) ;
#4788=CARTESIAN_POINT ( 'NONE',  ( -21.27752276159345968, 30.13625835399255593, 54.99767865737477734 ) ) ;
#4789=CARTESIAN_POINT ( 'NONE',  ( -35.05918829505000645, 27.97290950744599769, 58.85000000000000142 ) ) ;
#4793=CARTESIAN_POINT ( 'NONE',  ( -34.05918829504999934, 10.97290950744599947, 56.84999999999999432 ) ) ;
#4794=EDGE_CURVE ( 'NONE', #7262, #6072, #5637, .T. ) ;
#4795=AXIS2_PLACEMENT_3D ( 'NONE', #12375, #564, #10281 ) ;
#4797=CARTESIAN_POINT ( 'NONE',  ( -10.82033510625394079, -2.574630058508199593, 63.45000000000000284 ) ) ;
#4798=ORIENTED_EDGE ( 'NONE', *, *, #8003, .F. ) ;
#4799=DIRECTION ( 'NONE',  ( -0.4528443260392611136, -0.8915896008669277339, 0.000000000000000000 ) ) ;
#4800=( NAMED_UNIT ( * ) PLANE_ANGLE_UNIT ( ) SI_UNIT ( $, .RADIAN. ) );
#4803=DIRECTION ( 'NONE',  ( 0.000000000000000000, 0.000000000000000000, -1.000000000000000000 ) ) ;
#4806=FACE_OUTER_BOUND ( 'NONE', #4019, .T. ) ;
#4807=DIRECTION ( 'NONE',  ( 1.000000000000000000, 0.000000000000000000, 0.000000000000000000 ) ) ;
#4809=ADVANCED_FACE ( 'NONE', ( #3635 ), #9919, .T. ) ;
#4810=ORIENTED_EDGE ( 'NONE', *, *, #6387, .T. ) ;
#4811=ORIENTED_EDGE ( 'NONE', *, *, #3969, .F. ) ;
#4813=EDGE_CURVE ( 'NONE', #322, #10451, #2754, .T. ) ;
#4815=ORIENTED_EDGE ( 'NONE', *, *, #1738, .T. ) ;
#4816=ORIENTED_EDGE ( 'NONE', *, *, #3841, .T. ) ;
#4817=CARTESIAN_POINT ( 'NONE',  ( -18.05918829504999934, 10.97290950744599947, 62.85000000000000142 ) ) ;
#4821=CARTESIAN_POINT ( 'NONE',  ( -18.05918829504999934, 10.97290950744599947, 27.09999999999999787 ) ) ;
#4822=DIRECTION ( 'NONE',  ( 1.000000000000000000, 0.000000000000000000, 0.000000000000000000 ) ) ;
#4823=CARTESIAN_POINT ( 'NONE',  ( -1.059188295049996231, -6.027090492554000534, 58.85000000000000142 ) ) ;
#4824=CIRCLE ( 'NONE', #2846, 16.66282263685194920 ) ;
#4826=ORIENTED_EDGE ( 'NONE', *, *, #1528, .T. ) ;
#4830=EDGE_LOOP ( 'NONE', ( #11463, #11345 ) ) ;
#4831=DIRECTION ( 'NONE',  ( 0.000000000000000000, 0.000000000000000000, 1.000000000000000000 ) ) ;
#4832=ORIENTED_EDGE ( 'NONE', *, *, #4222, .F. ) ;
#4836=DIRECTION ( 'NONE',  ( 0.000000000000000000, 0.000000000000000000, 1.000000000000000000 ) ) ;
#4838=AXIS2_PLACEMENT_3D ( 'NONE', #7237, #1960, #6194 ) ;
#4839=ADVANCED_FACE ( 'NONE', ( #10324 ), #49, .F. ) ;
#4841=DIRECTION ( 'NONE',  ( 1.000000000000000000, 0.000000000000000000, 0.000000000000000000 ) ) ;
#4842=LINE ( 'NONE', #12329, #13152 ) ;
#4843=DIRECTION ( 'NONE',  ( 0.000000000000000000, 0.000000000000000000, 1.000000000000000000 ) ) ;
#4844=EDGE_LOOP ( 'NONE', ( #8143, #7144, #8830, #11108, #12047 ) ) ;
#4845=AXIS2_PLACEMENT_3D ( 'NONE', #13455, #3899, #12410 ) ;
#4847=ORIENTED_EDGE ( 'NONE', *, *, #10569, .T. ) ;
#4849=EDGE_LOOP ( 'NONE', ( #9696, #82, #5965, #9368 ) ) ;
#4850=CARTESIAN_POINT ( 'NONE',  ( 8.157609394192110841, 24.73469418910620021, 5.250000000000000000 ) ) ;
#4852=DIRECTION ( 'NONE',  ( 0.000000000000000000, 1.672022627447524993E-15, 1.000000000000000000 ) ) ;
#4853=EDGE_CURVE ( 'NONE', #11902, #4325, #8979, .T. ) ;
#4854=CARTESIAN_POINT ( 'NONE',  ( -21.42523896548032880, 30.11514052156897847, 59.42030264396898787 ) ) ;
#4857=CARTESIAN_POINT ( 'NONE',  ( -39.30918829504999934, -6.027090492554000534, 64.35000000000000853 ) ) ;
#4859=CIRCLE ( 'NONE', #7076, 1.725000000000000755 ) ;
#4863=ORIENTED_EDGE ( 'NONE', *, *, #12315, .T. ) ;
#4866=ORIENTED_EDGE ( 'NONE', *, *, #9195, .T. ) ;
#4867=AXIS2_PLACEMENT_3D ( 'NONE', #2422, #9809, #4632 ) ;
#4869=FACE_OUTER_BOUND ( 'NONE', #11493, .T. ) ;
#4872=DIRECTION ( 'NONE',  ( 0.000000000000000000, 0.000000000000000000, -1.000000000000000000 ) ) ;
#4873=DIRECTION ( 'NONE',  ( 0.000000000000000000, 0.000000000000000000, 1.000000000000000000 ) ) ;
#4874=DIRECTION ( 'NONE',  ( -0.000000000000000000, -0.000000000000000000, -1.000000000000000000 ) ) ;
#4875=CARTESIAN_POINT ( 'NONE',  ( -34.78181777225609750, 10.00028003023991907, 62.14999999999999858 ) ) ;
#4878=CARTESIAN_POINT ( 'NONE',  ( -18.05918829504999934, 10.97290950744599947, 7.250000000000000000 ) ) ;
#4881=DIRECTION ( 'NONE',  ( 0.000000000000000000, 0.000000000000000000, -1.000000000000000000 ) ) ;
#4883=CIRCLE ( 'NONE', #1523, 3.450000000000001510 ) ;
#4885=VECTOR ( 'NONE', #2061, 1000.000000000000000 ) ;
#4886=ORIENTED_EDGE ( 'NONE', *, *, #12780, .F. ) ;
#4887=ORIENTED_EDGE ( 'NONE', *, *, #2326, .T. ) ;
#4891=AXIS2_PLACEMENT_3D ( 'NONE', #1157, #1021, #6469 ) ;
#4893=CARTESIAN_POINT ( 'NONE',  ( 1.640811704950000172, 27.97290950744599769, 58.85000000000000142 ) ) ;
#4894=AXIS2_PLACEMENT_3D ( 'NONE', #6181, #6053, #747 ) ;
#4896=DIRECTION ( 'NONE',  ( 0.000000000000000000, 0.000000000000000000, 1.000000000000000000 ) ) ;
#4898=DIRECTION ( 'NONE',  ( -1.000000000000000000, 0.000000000000000000, 0.000000000000000000 ) ) ;
#4899=CARTESIAN_POINT ( 'NONE',  ( -17.23821357112329977, 5.029341513162310484, 67.84999999999999432 ) ) ;
#4900=CARTESIAN_POINT ( 'NONE',  ( -1.396365658198039927, 10.97290950744599947, 17.25000000000000000 ) ) ;
#4901=EDGE_CURVE ( 'NONE', #7761, #1281, #12933, .T. ) ;
#4903=AXIS2_PLACEMENT_3D ( 'NONE', #5551, #532, #12195 ) ;
#4905=FACE_OUTER_BOUND ( 'NONE', #13073, .T. ) ;
#4907=ORIENTED_EDGE ( 'NONE', *, *, #3469, .F. ) ;
#4913=AXIS2_PLACEMENT_3D ( 'NONE', #4669, #601, #7862 ) ;
#4914=DIRECTION ( 'NONE',  ( 1.000000000000000000, 0.000000000000000000, 0.000000000000000000 ) ) ;
#4915=AXIS2_PLACEMENT_3D ( 'NONE', #10791, #1206, #5460 ) ;
#4916=DIRECTION ( 'NONE',  ( -1.000000000000000000, 0.000000000000000000, 0.000000000000000000 ) ) ;
#4918=EDGE_CURVE ( 'NONE', #1530, #6060, #7177, .T. ) ;
#4922=DIRECTION ( 'NONE',  ( -0.4528443260392609471, -0.8915896008669278450, 0.000000000000000000 ) ) ;
#4926=DIRECTION ( 'NONE',  ( -1.000000000000000000, 0.000000000000000000, 0.000000000000000000 ) ) ;
#4928=VECTOR ( 'NONE', #3204, 1000.000000000000227 ) ;
#4932=EDGE_LOOP ( 'NONE', ( #142, #6301, #12927, #2197 ) ) ;
#4934=EDGE_CURVE ( 'NONE', #5535, #1130, #1657, .T. ) ;
#4935=CARTESIAN_POINT ( 'NONE',  ( -19.47340185742309870, 26.91028695795525039, 56.84999999999999432 ) ) ;
#4936=AXIS2_PLACEMENT_3D ( 'NONE', #10531, #11574, #671 ) ;
#4937=ORIENTED_EDGE ( 'NONE', *, *, #2064, .T. ) ;
#4939=VERTEX_POINT ( 'NONE', #5905 ) ;
#4940=DIRECTION ( 'NONE',  ( -0.7071067811865474617, 8.659560562354903276E-17, 0.7071067811865474617 ) ) ;
#4942=DIRECTION ( 'NONE',  ( 1.000000000000000000, -1.679942734630170865E-14, 0.000000000000000000 ) ) ;
#4945=CARTESIAN_POINT ( 'NONE',  ( -1.336558817843898073, 10.00028003023991907, 62.14999999999999858 ) ) ;
#4946=LINE ( 'NONE', #13462, #9798 ) ;
#4947=CARTESIAN_POINT ( 'NONE',  ( -18.88016301897669891, 16.91647750172969822, 67.84999999999999432 ) ) ;
#4948=CARTESIAN_POINT ( 'NONE',  ( -18.05918829504999934, 10.00028003023991907, 63.45000000000000284 ) ) ;
#4949=( LENGTH_UNIT ( ) NAMED_UNIT ( * ) SI_UNIT ( .MILLI., .METRE. ) );
#4950=EDGE_CURVE ( 'NONE', #2935, #7296, #2941, .T. ) ;
#4952=VERTEX_POINT ( 'NONE', #9135 ) ;
#4953=EDGE_CURVE ( 'NONE', #7844, #5689, #5071, .T. ) ;
#4957=ORIENTED_EDGE ( 'NONE', *, *, #10912, .F. ) ;
#4958=ORIENTED_EDGE ( 'NONE', *, *, #7488, .F. ) ;
#4959=DIRECTION ( 'NONE',  ( 1.000000000000000000, 0.000000000000000000, 0.000000000000000000 ) ) ;
#4960=AXIS2_PLACEMENT_3D ( 'NONE', #2372, #8774, #4655 ) ;
#4961=DIRECTION ( 'NONE',  ( 0.9496839325805427334, 0.3132098788326367345, 0.000000000000000000 ) ) ;
#4964=LINE ( 'NONE', #10280, #5795 ) ;
#4967=ORIENTED_EDGE ( 'NONE', *, *, #12273, .T. ) ;
#4969=ORIENTED_EDGE ( 'NONE', *, *, #986, .T. ) ;
#4970=CARTESIAN_POINT ( 'NONE',  ( -15.30684414934278337, 30.19664696495205902, 60.37107827764424428 ) ) ;
#4971=ORIENTED_EDGE ( 'NONE', *, *, #3572, .F. ) ;
#4972=DIRECTION ( 'NONE',  ( 0.000000000000000000, 0.000000000000000000, -1.000000000000000000 ) ) ;
#4973=ORIENTED_EDGE ( 'NONE', *, *, #13674, .F. ) ;
#4975=CARTESIAN_POINT ( 'NONE',  ( -18.05918829504999934, 10.97290950744599947, 61.72253826518770836 ) ) ;
#4976=ORIENTED_EDGE ( 'NONE', *, *, #3526, .F. ) ;
#4977=DIRECTION ( 'NONE',  ( 0.4528443260392608916, 0.8915896008669277339, 0.000000000000000000 ) ) ;
#4978=AXIS2_PLACEMENT_3D ( 'NONE', #13354, #12328, #2775 ) ;
#4979=DIRECTION ( 'NONE',  ( -1.000000000000000000, 0.000000000000000000, 0.000000000000000000 ) ) ;
#4980=CARTESIAN_POINT ( 'NONE',  ( -24.37001676333060018, -4.028726038184999858, 63.45000000000000284 ) ) ;
#4984=ORIENTED_EDGE ( 'NONE', *, *, #11704, .F. ) ;
#4986=VERTEX_POINT ( 'NONE', #9209 ) ;
#4987=EDGE_CURVE ( 'NONE', #87, #6052, #13459, .T. ) ;
#4991=DIRECTION ( 'NONE',  ( 0.000000000000000000, 1.000000000000000000, 2.202823461557851130E-15 ) ) ;
#4992=CARTESIAN_POINT ( 'NONE',  ( -18.05918829504999934, 10.97290950744599947, 60.65000000000000568 ) ) ;
#4993=DIRECTION ( 'NONE',  ( 1.000000000000000000, 0.000000000000000000, 0.000000000000000000 ) ) ;
#4997=VERTEX_POINT ( 'NONE', #10532 ) ;
#4998=ORIENTED_EDGE ( 'NONE', *, *, #10096, .T. ) ;
#5001=FACE_OUTER_BOUND ( 'NONE', #11172, .T. ) ;
#5002=EDGE_CURVE ( 'NONE', #12622, #3976, #9201, .T. ) ;
#5003=CARTESIAN_POINT ( 'NONE',  ( -24.20502162805000168, 10.97290950744599947, 61.10999999999999943 ) ) ;
#5004=PLANE ( 'NONE',  #4281 ) ;
#5005=ORIENTED_EDGE ( 'NONE', *, *, #10479, .F. ) ;
#5006=DIRECTION ( 'NONE',  ( 0.000000000000000000, 0.000000000000000000, -1.000000000000000000 ) ) ;
#5007=CARTESIAN_POINT ( 'NONE',  ( -18.05918829504999934, 10.97290950744599947, 60.04999999999999716 ) ) ;
#5013=AXIS2_PLACEMENT_3D ( 'NONE', #8534, #1195, #2348 ) ;
#5017=VERTEX_POINT ( 'NONE', #4174 ) ;
#5020=CARTESIAN_POINT ( 'NONE',  ( -0.3963656581980404825, 10.97290950744599947, 7.250000000000000000 ) ) ;
#5021=DIRECTION ( 'NONE',  ( 0.000000000000000000, 0.000000000000000000, -1.000000000000000000 ) ) ;
#5024=DIRECTION ( 'NONE',  ( 1.000000000000000000, 0.000000000000000000, 0.000000000000000000 ) ) ;
#5025=EDGE_CURVE ( 'NONE', #11045, #4627, #2302, .T. ) ;
#5027=EDGE_LOOP ( 'NONE', ( #1358, #6130, #5340, #12715 ) ) ;
#5028=CIRCLE ( 'NONE', #9723, 2.800000000000000266 ) ;
#5029=ORIENTED_EDGE ( 'NONE', *, *, #9844, .T. ) ;
#5030=CARTESIAN_POINT ( 'NONE',  ( -14.93961223533927729, 30.15001770392374070, 54.82814931419168403 ) ) ;
#5031=ORIENTED_EDGE ( 'NONE', *, *, #9459, .F. ) ;
#5033=DIRECTION ( 'NONE',  ( 0.000000000000000000, 0.000000000000000000, -1.000000000000000000 ) ) ;
#5034=EDGE_LOOP ( 'NONE', ( #9608, #5463, #1029, #1123 ) ) ;
#5035=CARTESIAN_POINT ( 'NONE',  ( -41.50918829505000218, 27.97290950744599769, 5.250000000000000000 ) ) ;
#5036=PLANE ( 'NONE',  #3996 ) ;
#5037=DIRECTION ( 'NONE',  ( 0.9496839325805410681, 0.3132098788326420080, 0.000000000000000000 ) ) ;
#5038=DIRECTION ( 'NONE',  ( -1.000000000000000000, 0.000000000000000000, 0.000000000000000000 ) ) ;
#5039=CARTESIAN_POINT ( 'NONE',  ( -5.309188295050000228, -6.027090492554000534, 58.85000000000000142 ) ) ;
#5048=ORIENTED_EDGE ( 'NONE', *, *, #1465, .T. ) ;
#5049=EDGE_LOOP ( 'NONE', ( #1304, #3911, #5591, #1634 ) ) ;
#5051=CARTESIAN_POINT ( 'NONE',  ( -19.35259110363697488, 30.32455137612451068, 61.45271661549876541 ) ) ;
#5052=DIRECTION ( 'NONE',  ( 0.000000000000000000, 0.000000000000000000, 1.000000000000000000 ) ) ;
#5054=CARTESIAN_POINT ( 'NONE',  ( -18.05918829504999934, 10.97290950744599947, 62.14999999999999858 ) ) ;
#5058=VERTEX_POINT ( 'NONE', #103 ) ;
#5059=VECTOR ( 'NONE', #4872, 1000.000000000000000 ) ;
#5060=ADVANCED_FACE ( 'NONE', ( #9480 ), #6740, .F. ) ;
#5061=EDGE_CURVE ( 'NONE', #3451, #665, #5846, .T. ) ;
#5063=CARTESIAN_POINT ( 'NONE',  ( -10.25088531517539892, 30.80589556422609832, 17.25000000000000000 ) ) ;
#5065=CLOSED_SHELL ( 'NONE', ( #139, #1106, #8862, #11505, #13732, #4287, #13440, #2673, #6378, #4489, #6270, #2742, #7506, #5401, #10149, #13359, #9282, #6736, #10796, #7694, #6156, #1923, #12386, #11917, #10833, #6836, #7818, #7661, #12926, #7671, #2847, #3416, #2650, #1013, #3354, #4245, #6456, #5779, #521, #7582, #5577, #2094, #13208, #13464, #11511, #9551, #6968, #10720, #8743, #2129, #2794, #1739, #632, #7127, #7063, #12830, #5426, #7896, #1426, #13032, #2055, #7670, #5741, #4540, #12546, #3486, #10423, #4839, #3081, #7801, #5184, #3414, #4809, #9003, #9293, #6691, #7135, #7044, #7065, #7755, #8724, #8781, #3587, #1665, #7762, #1543, #4623, #1761, #5494, #3162, #2217, #3116, #9350, #13291, #13683, #7784, #3305, #1936, #7887 ) ) ;
#5066=ORIENTED_EDGE ( 'NONE', *, *, #2914, .F. ) ;
#5067=CARTESIAN_POINT ( 'NONE',  ( -11.91335496205000055, 10.97290950744599947, 61.10999999999999943 ) ) ;
#5069=AXIS2_PLACEMENT_3D ( 'NONE', #10973, #6819, #10052 ) ;
#5070=CARTESIAN_POINT ( 'NONE',  ( -24.40502162805000097, 10.97290950744599947, 60.40999999999999659 ) ) ;
#5071=LINE ( 'NONE', #10190, #8076 ) ;
#5072=DIRECTION ( 'NONE',  ( 0.000000000000000000, 0.000000000000000000, 1.000000000000000000 ) ) ;
#5076=DIRECTION ( 'NONE',  ( 0.000000000000000000, 0.000000000000000000, -1.000000000000000000 ) ) ;
#5077=VERTEX_POINT ( 'NONE', #8623 ) ;
#5080=EDGE_CURVE ( 'NONE', #12858, #13546, #1389, .T. ) ;
#5081=ORIENTED_EDGE ( 'NONE', *, *, #10536, .F. ) ;
#5082=ORIENTED_EDGE ( 'NONE', *, *, #12419, .T. ) ;
#5084=ORIENTED_EDGE ( 'NONE', *, *, #12372, .F. ) ;
#5085=ORIENTED_EDGE ( 'NONE', *, *, #8157, .T. ) ;
#5086=DIRECTION ( 'NONE',  ( 1.000000000000000000, 0.000000000000000000, 0.000000000000000000 ) ) ;
#5088=AXIS2_PLACEMENT_3D ( 'NONE', #125, #1241, #4337 ) ;
#5090=CIRCLE ( 'NONE', #9109, 5.000000000000000888 ) ;
#5091=AXIS2_PLACEMENT_3D ( 'NONE', #8239, #12502, #2961 ) ;
#5092=CARTESIAN_POINT ( 'NONE',  ( -24.37001676333060018, -4.028726038184999858, 63.45000000000000284 ) ) ;
#5094=PLANE ( 'NONE',  #6419 ) ;
#5095=CARTESIAN_POINT ( 'NONE',  ( -1.059188295049996231, 27.97290950744599769, 64.85000000000000853 ) ) ;
#5097=( GEOMETRIC_REPRESENTATION_CONTEXT ( 3 ) GLOBAL_UNCERTAINTY_ASSIGNED_CONTEXT ( ( #6416 ) ) GLOBAL_UNIT_ASSIGNED_CONTEXT ( ( #4949, #11717, #48 ) ) REPRESENTATION_CONTEXT ( 'NONE', 'WORKASPACE' ) );
#5098=CONICAL_SURFACE ( 'NONE', #11789, 4.250000000000000000, 0.7853981633974518317 ) ;
#5102=CARTESIAN_POINT ( 'NONE',  ( -14.74723118919472853, 30.12306837293317230, 59.53343286463421435 ) ) ;
#5103=ORIENTED_EDGE ( 'NONE', *, *, #10027, .T. ) ;
#5105=CARTESIAN_POINT ( 'NONE',  ( -24.47918829505000105, 10.97290950744599947, 64.85000000000000853 ) ) ;
#5108=CARTESIAN_POINT ( 'NONE',  ( -1.059188295049996231, 27.97290950744599769, 64.85000000000000853 ) ) ;
#5109=ORIENTED_EDGE ( 'NONE', *, *, #7436, .T. ) ;
#5112=CARTESIAN_POINT ( 'NONE',  ( -5.309188295050000228, 27.97290950744599769, 64.85000000000000853 ) ) ;
#5115=CARTESIAN_POINT ( 'NONE',  ( -5.631644894983189431, 10.97290950744599947, 17.25000000000000000 ) ) ;
#5116=CIRCLE ( 'NONE', #12707, 0.9499999999999995115 ) ;
#5118=ORIENTED_EDGE ( 'NONE', *, *, #616, .T. ) ;
#5119=ORIENTED_EDGE ( 'NONE', *, *, #11520, .T. ) ;
#5122=VECTOR ( 'NONE', #2588, 1000.000000000000000 ) ;
#5124=DIRECTION ( 'NONE',  ( -1.000000000000000000, 0.000000000000000000, 0.000000000000000000 ) ) ;
#5125=CARTESIAN_POINT ( 'NONE',  ( -18.05918829504999934, 10.97290950744599947, 61.86500000000000199 ) ) ;
#5132=AXIS2_PLACEMENT_3D ( 'NONE', #5207, #2023, #12816 ) ;
#5135=CARTESIAN_POINT ( 'NONE',  ( -41.50918829505000218, 27.97290950744599769, 17.25000000000000000 ) ) ;
#5137=VERTEX_POINT ( 'NONE', #8493 ) ;
#5142=AXIS2_PLACEMENT_3D ( 'NONE', #763, #824, #12500 ) ;
#5144=ORIENTED_EDGE ( 'NONE', *, *, #2829, .F. ) ;
#5145=CARTESIAN_POINT ( 'NONE',  ( -1.059188295049996231, 10.97290950744599947, 62.14999999999999858 ) ) ;
#5147=MANIFOLD_SOLID_BREP ( 'NONE', #12653 ) ;
#5148=CARTESIAN_POINT ( 'NONE',  ( -18.05918829504999934, 10.97290950744599947, 62.14999999999999858 ) ) ;
#5149=EDGE_CURVE ( 'NONE', #722, #13003, #6522, .T. ) ;
#5150=CARTESIAN_POINT ( 'NONE',  ( -18.05918829504999934, 10.00028003023991907, 62.14999999999999858 ) ) ;
#5153=ORIENTED_EDGE ( 'NONE', *, *, #1161, .F. ) ;
#5155=CIRCLE ( 'NONE', #7356, 1.500000000000001332 ) ;
#5158=AXIS2_PLACEMENT_3D ( 'NONE', #13793, #3014, #3966 ) ;
#5160=EDGE_CURVE ( 'NONE', #4325, #11902, #9435, .T. ) ;
#5165=CARTESIAN_POINT ( 'NONE',  ( -18.05918829504999934, 2.872909508741170015, 63.35000000000700027 ) ) ;
#5167=CIRCLE ( 'NONE', #13420, 6.000000000000000888 ) ;
#5168=CARTESIAN_POINT ( 'NONE',  ( -41.50918829505000218, -6.027090492554000534, 5.250000000000000000 ) ) ;
#5169=AXIS2_PLACEMENT_3D ( 'NONE', #5054, #13506, #4926 ) ;
#5171=CARTESIAN_POINT ( 'NONE',  ( -14.48404530696549841, 30.08351321291744185, 55.79525418935277514 ) ) ;
#5172=ORIENTED_EDGE ( 'NONE', *, *, #13461, .T. ) ;
#5175=CYLINDRICAL_SURFACE ( 'NONE', #8840, 6.450000000000019718 ) ;
#5178=ORIENTED_EDGE ( 'NONE', *, *, #7879, .F. ) ;
#5180=CYLINDRICAL_SURFACE ( 'NONE', #8668, 6.449999999999997513 ) ;
#5182=CARTESIAN_POINT ( 'NONE',  ( -18.05918829504999934, 10.97290950744599947, 61.65955166399999854 ) ) ;
#5183=LINE ( 'NONE', #9643, #9678 ) ;
#5184=ADVANCED_FACE ( 'NONE', ( #3473 ), #11079, .T. ) ;
#5185=CARTESIAN_POINT ( 'NONE',  ( -16.55945684168713683, 27.90662751739518654, 57.54990028585785922 ) ) ;
#5187=CARTESIAN_POINT ( 'NONE',  ( -18.05918829504999934, 10.97290950744599947, 60.60999999999999943 ) ) ;
#5189=EDGE_LOOP ( 'NONE', ( #6093, #9371 ) ) ;
#5191=EDGE_LOOP ( 'NONE', ( #3405, #4702, #10938, #7876 ) ) ;
#5192=CARTESIAN_POINT ( 'NONE',  ( -10.38347696868452097, 26.08535324214045303, 58.35000000000000142 ) ) ;
#5194=EDGE_CURVE ( 'NONE', #11380, #10426, #12331, .T. ) ;
#5196=CARTESIAN_POINT ( 'NONE',  ( -19.05204298599095480, 26.94232003179371304, 56.22521585200335181 ) ) ;
#5198=CARTESIAN_POINT ( 'NONE',  ( -1.059188295049996231, -6.027090492554000534, 68.85549045786049760 ) ) ;
#5200=SHAPE_DEFINITION_REPRESENTATION ( #5684, #13195 ) ;
#5201=EDGE_CURVE ( 'NONE', #1818, #3446, #1496, .T. ) ;
#5202=AXIS2_PLACEMENT_3D ( 'NONE', #13495, #3937, #644 ) ;
#5207=CARTESIAN_POINT ( 'NONE',  ( -18.05918829504999934, 10.97290950744599947, 58.54999999999999716 ) ) ;
#5208=PLANE ( 'NONE',  #13313 ) ;
#5212=MANIFOLD_SOLID_BREP ( 'NONE', #110 ) ;
#5213=CARTESIAN_POINT ( 'NONE',  ( -1.059188295049996231, 27.97290950744599769, 7.250000000000000000 ) ) ;
#5214=CARTESIAN_POINT ( 'NONE',  ( -18.05918829504999934, 10.97290950744599947, 30.59999999999999787 ) ) ;
#5217=EDGE_CURVE ( 'NONE', #7297, #7051, #10873, .T. ) ;
#5219=VERTEX_POINT ( 'NONE', #1292 ) ;
#5222=ORIENTED_EDGE ( 'NONE', *, *, #5332, .T. ) ;
#5224=CARTESIAN_POINT ( 'NONE',  ( -10.82033510625394079, -2.574630058508199593, 62.14999999999999858 ) ) ;
#5226=LINE ( 'NONE', #2885, #13120 ) ;
#5227=DIRECTION ( 'NONE',  ( 0.000000000000000000, 0.000000000000000000, 1.000000000000000000 ) ) ;
#5232=ADVANCED_FACE ( 'NONE', ( #9192, #6947 ), #9044, .T. ) ;
#5233=CARTESIAN_POINT ( 'NONE',  ( -14.76278877871134299, 30.12521254568601847, 55.14084190974008237 ) ) ;
#5235=ORIENTED_EDGE ( 'NONE', *, *, #9946, .T. ) ;
#5238=DIRECTION ( 'NONE',  ( -1.000000000000000000, 0.000000000000000000, 0.000000000000000000 ) ) ;
#5240=DIRECTION ( 'NONE',  ( -1.000000000000000000, 0.000000000000000000, 0.000000000000000000 ) ) ;
#5241=DIRECTION ( 'NONE',  ( 3.441911658684139926E-17, 0.000000000000000000, 1.000000000000000000 ) ) ;
#5242=LINE ( 'NONE', #9513, #4709 ) ;
#5244=EDGE_CURVE ( 'NONE', #10600, #13687, #10554, .T. ) ;
#5246=ORIENTED_EDGE ( 'NONE', *, *, #8102, .T. ) ;
#5248=ORIENTED_EDGE ( 'NONE', *, *, #1348, .T. ) ;
#5251=VERTEX_POINT ( 'NONE', #12399 ) ;
#5253=CARTESIAN_POINT ( 'NONE',  ( -35.05918829505000645, -6.027090492554000534, 5.250000000000000000 ) ) ;
#5254=EDGE_CURVE ( 'NONE', #5356, #10337, #13436, .T. ) ;
#5255=DIRECTION ( 'NONE',  ( 0.000000000000000000, 0.000000000000000000, 1.000000000000000000 ) ) ;
#5257=CARTESIAN_POINT ( 'NONE',  ( -5.631644894983189431, 10.97290950744599947, 5.250000000000000000 ) ) ;
#5260=ORIENTED_EDGE ( 'NONE', *, *, #7142, .F. ) ;
#5261=EDGE_CURVE ( 'NONE', #95, #1822, #8090, .T. ) ;
#5262=AXIS2_PLACEMENT_3D ( 'NONE', #11464, #2710, #588 ) ;
#5263=ORIENTED_EDGE ( 'NONE', *, *, #7719, .F. ) ;
#5264=LINE ( 'NONE', #7417, #13739 ) ;
#5267=CARTESIAN_POINT ( 'NONE',  ( -18.05918829504999934, 10.97290950744599947, 56.84999999999999432 ) ) ;
#5270=SURFACE_STYLE_USAGE ( .BOTH. , #10591 ) ;
#5271=DIRECTION ( 'NONE',  ( 0.000000000000000000, 0.000000000000000000, -1.000000000000000000 ) ) ;
#5272=CARTESIAN_POINT ( 'NONE',  ( -18.05918829504999934, 7.130333642789880244, 17.25000000000000000 ) ) ;
#5275=FACE_OUTER_BOUND ( 'NONE', #13225, .T. ) ;
#5277=EDGE_CURVE ( 'NONE', #9433, #7877, #11224, .T. ) ;
#5278=ORIENTED_EDGE ( 'NONE', *, *, #10317, .T. ) ;
#5279=ORIENTED_EDGE ( 'NONE', *, *, #6877, .F. ) ;
#5280=AXIS2_PLACEMENT_3D ( 'NONE', #1654, #9131, #12204 ) ;
#5282=ORIENTED_EDGE ( 'NONE', *, *, #3726, .T. ) ;
#5283=VERTEX_POINT ( 'NONE', #13302 ) ;
#5284=ORIENTED_EDGE ( 'NONE', *, *, #6306, .T. ) ;
#5286=CARTESIAN_POINT ( 'NONE',  ( -13.44794508215399453, 8.373466233319598828, 68.55654520525476414 ) ) ;
#5288=LINE ( 'NONE', #11453, #8034 ) ;
#5289=FACE_BOUND ( 'NONE', #6849, .T. ) ;
#5293=CONICAL_SURFACE ( 'NONE', #6448, 17.00000000000000000, 0.7853981633974476129 ) ;
#5299=AXIS2_PLACEMENT_3D ( 'NONE', #5840, #11032, #2660 ) ;
#5301=ORIENTED_EDGE ( 'NONE', *, *, #6271, .T. ) ;
#5305=CYLINDRICAL_SURFACE ( 'NONE', #10518, 2.500000000000000000 ) ;
#5308=ADVANCED_FACE ( 'NONE', ( #12341 ), #8198, .F. ) ;
#5309=FACE_OUTER_BOUND ( 'NONE', #11026, .T. ) ;
#5311=CIRCLE ( 'NONE', #10019, 17.00000000000000355 ) ;
#5313=AXIS2_PLACEMENT_3D ( 'NONE', #2268, #5439, #8528 ) ;
#5314=ORIENTED_EDGE ( 'NONE', *, *, #11858, .T. ) ;
#5315=CARTESIAN_POINT ( 'NONE',  ( -12.69835982676941910, -4.028726038184999858, 62.14999999999999858 ) ) ;
#5317=ORIENTED_EDGE ( 'NONE', *, *, #10146, .F. ) ;
#5319=DIRECTION ( 'NONE',  ( 0.000000000000000000, 0.000000000000000000, -1.000000000000000000 ) ) ;
#5322=ORIENTED_EDGE ( 'NONE', *, *, #12335, .F. ) ;
#5323=DIRECTION ( 'NONE',  ( 1.000000000000000000, -9.130123557772668088E-16, 0.000000000000000000 ) ) ;
#5325=FACE_OUTER_BOUND ( 'NONE', #7219, .T. ) ;
#5326=CARTESIAN_POINT ( 'NONE',  ( 2.262399129208275017, -0.4981161769137599782, 5.250000000000000000 ) ) ;
#5327=EDGE_CURVE ( 'NONE', #8057, #506, #10245, .T. ) ;
#5330=CIRCLE ( 'NONE', #6676, 16.75000000000000355 ) ;
#5331=AXIS2_PLACEMENT_3D ( 'NONE', #5476, #4453, #3212 ) ;
#5332=EDGE_CURVE ( 'NONE', #13079, #1264, #56, .T. ) ;
#5333=DIRECTION ( 'NONE',  ( 0.4528443260392608360, 0.8915896008669278450, 0.000000000000000000 ) ) ;
#5336=CARTESIAN_POINT ( 'NONE',  ( -24.20502162805000168, 10.97290950744599947, 61.10999999999999943 ) ) ;
#5337=CARTESIAN_POINT ( 'NONE',  ( -18.05918829504999934, 10.97290950744599947, 60.04999999999999716 ) ) ;
#5338=CARTESIAN_POINT ( 'NONE',  ( -20.81153244793331325, 30.19664696409543581, 54.32892173082856857 ) ) ;
#5339=FILL_AREA_STYLE ('',( #2091 ) ) ;
#5340=ORIENTED_EDGE ( 'NONE', *, *, #4604, .T. ) ;
#5341=DIRECTION ( 'NONE',  ( -0.9496839325805421783, 0.3132098788326385663, 0.000000000000000000 ) ) ;
#5343=DIRECTION ( 'NONE',  ( 0.000000000000000000, 0.000000000000000000, -1.000000000000000000 ) ) ;
#5345=ORIENTED_EDGE ( 'NONE', *, *, #12034, .F. ) ;
#5346=CARTESIAN_POINT ( 'NONE',  ( -27.61808667955315144, -3.085093966544995236, 62.14999999999999858 ) ) ;
#5347=CONICAL_SURFACE ( 'NONE', #1333, 7.618085573000000110, 0.1329427246665018103 ) ;
#5348=CIRCLE ( 'NONE', #3360, 4.750000000000000888 ) ;
#5349=EDGE_CURVE ( 'NONE', #6678, #918, #5629, .T. ) ;
#5352=CARTESIAN_POINT ( 'NONE',  ( -35.05918829505000645, -6.027090492554000534, 64.85000000000000853 ) ) ;
#5353=VECTOR ( 'NONE', #13137, 1000.000000000000114 ) ;
#5354=VECTOR ( 'NONE', #9213, 1000.000000000000000 ) ;
#5356=VERTEX_POINT ( 'NONE', #11143 ) ;
#5357=ORIENTED_EDGE ( 'NONE', *, *, #3001, .T. ) ;
#5358=DIRECTION ( 'NONE',  ( 0.1325514707600310149, 0.000000000000000000, -0.9911761234005551646 ) ) ;
#5365=AXIS2_PLACEMENT_3D ( 'NONE', #11221, #6808, #1574 ) ;
#5366=ADVANCED_FACE ( 'NONE', ( #1571 ), #10110, .F. ) ;
#5368=DIRECTION ( 'NONE',  ( 0.000000000000000000, 0.000000000000000000, 1.000000000000000000 ) ) ;
#5371=CIRCLE ( 'NONE', #5590, 6.000000000000000888 ) ;
#5372=DIRECTION ( 'NONE',  ( 0.000000000000000000, 0.000000000000000000, 1.000000000000000000 ) ) ;
#5373=CIRCLE ( 'NONE', #3382, 17.00000000000000355 ) ;
#5374=SURFACE_STYLE_USAGE ( .BOTH. , #6427 ) ;
#5375=AXIS2_PLACEMENT_3D ( 'NONE', #13098, #2514, #3546 ) ;
#5376=CARTESIAN_POINT ( 'NONE',  ( -10.38347696868452097, 26.08535324214045303, 57.54999999999999716 ) ) ;
#5377=PLANE ( 'NONE',  #6655 ) ;
#5378=DIRECTION ( 'NONE',  ( 1.000000000000000000, 0.000000000000000000, 0.000000000000000000 ) ) ;
#5379=DIRECTION ( 'NONE',  ( -1.000000000000000000, 0.000000000000000000, 0.000000000000000000 ) ) ;
#5385=LINE ( 'NONE', #3249, #2819 ) ;
#5386=ORIENTED_EDGE ( 'NONE', *, *, #12966, .T. ) ;
#5387=VERTEX_POINT ( 'NONE', #9598 ) ;
#5392=DIRECTION ( 'NONE',  ( -0.3202092937642119774, -0.6304490528084089052, 0.7071067811865507924 ) ) ;
#5393=CARTESIAN_POINT ( 'NONE',  ( -18.05918829504999934, 10.97290950744599947, 61.25000000000000000 ) ) ;
#5395=DIRECTION ( 'NONE',  ( 0.000000000000000000, 0.000000000000000000, -1.000000000000000000 ) ) ;
#5396=DIRECTION ( 'NONE',  ( 0.000000000000000000, 0.000000000000000000, -1.000000000000000000 ) ) ;
#5401=ADVANCED_FACE ( 'NONE', ( #28 ), #1137, .T. ) ;
#5402=ORIENTED_EDGE ( 'NONE', *, *, #7719, .T. ) ;
#5403=ORIENTED_EDGE ( 'NONE', *, *, #998, .F. ) ;
#5405=LINE ( 'NONE', #6331, #3054 ) ;
#5410=CARTESIAN_POINT ( 'NONE',  ( -20.23067423319998426, 30.25856101892194872, 53.76667154643602231 ) ) ;
#5413=CARTESIAN_POINT ( 'NONE',  ( -19.91165729514404603, 13.07251866242952154, 23.90000000000000213 ) ) ;
#5414=DIRECTION ( 'NONE',  ( 0.000000000000000000, 0.000000000000000000, -1.000000000000000000 ) ) ;
#5416=CARTESIAN_POINT ( 'NONE',  ( -12.54628844161313950, -7.366404416634599883, 62.14999999999999858 ) ) ;
#5418=EDGE_CURVE ( 'NONE', #11380, #11449, #9400, .T. ) ;
#5419=ORIENTED_EDGE ( 'NONE', *, *, #5080, .T. ) ;
#5422=ORIENTED_EDGE ( 'NONE', *, *, #12998, .F. ) ;
#5424=ORIENTED_EDGE ( 'NONE', *, *, #13194, .T. ) ;
#5425=CYLINDRICAL_SURFACE ( 'NONE', #388, 4.750000000000000888 ) ;
#5426=ADVANCED_FACE ( 'NONE', ( #12745 ), #7209, .F. ) ;
#5432=DIRECTION ( 'NONE',  ( 0.000000000000000000, 0.000000000000000000, -1.000000000000000000 ) ) ;
#5435=CARTESIAN_POINT ( 'NONE',  ( -15.95913914146609613, 30.26546654951570048, 53.70790935732234317 ) ) ;
#5438=CARTESIAN_POINT ( 'NONE',  ( -21.16117192841894834, 4.865520741507539881, 64.54999999999999716 ) ) ;
#5439=DIRECTION ( 'NONE',  ( 0.000000000000000000, 0.000000000000000000, 1.000000000000000000 ) ) ;
#5440=EDGE_CURVE ( 'NONE', #8353, #5838, #8773, .T. ) ;
#5442=DIRECTION ( 'NONE',  ( 0.000000000000000000, 0.000000000000000000, -1.000000000000000000 ) ) ;
#5444=EDGE_CURVE ( 'NONE', #9493, #1604, #12041, .T. ) ;
#5448=ORIENTED_EDGE ( 'NONE', *, *, #6412, .F. ) ;
#5451=CARTESIAN_POINT ( 'NONE',  ( -27.15409092487699994, 0.3335619008453594714, 63.45000000000000284 ) ) ;
#5453=ORIENTED_EDGE ( 'NONE', *, *, #2288, .T. ) ;
#5454=ADVANCED_FACE ( 'NONE', ( #444 ), #5456, .T. ) ;
#5455=CARTESIAN_POINT ( 'NONE',  ( -23.24102627739274851, -6.265087914666289670, 63.45000000000000284 ) ) ;
#5456=CYLINDRICAL_SURFACE ( 'NONE', #6528, 34.70000000000000284 ) ;
#5458=DIRECTION ( 'NONE',  ( 0.000000000000000000, 0.000000000000000000, -1.000000000000000000 ) ) ;
#5459=CIRCLE ( 'NONE', #1226, 3.000000000000001332 ) ;
#5460=DIRECTION ( 'NONE',  ( 1.000000000000000000, 0.000000000000000000, 0.000000000000000000 ) ) ;
#5461=ORIENTED_EDGE ( 'NONE', *, *, #3088, .T. ) ;
#5462=CONICAL_SURFACE ( 'NONE', #8154, 5.500000000000002665, 0.7853981633974433940 ) ;
#5463=ORIENTED_EDGE ( 'NONE', *, *, #1868, .F. ) ;
#5470=CARTESIAN_POINT ( 'NONE',  ( -19.35500534946005402, 30.32416700404740340, 53.25030877638827320 ) ) ;
#5471=DIRECTION ( 'NONE',  ( 0.000000000000000000, 0.000000000000000000, 1.000000000000000000 ) ) ;
#5472=ORIENTED_EDGE ( 'NONE', *, *, #5025, .F. ) ;
#5473=DIRECTION ( 'NONE',  ( 0.000000000000000000, 0.000000000000000000, -1.000000000000000000 ) ) ;
#5474=DIRECTION ( 'NONE',  ( -0.4678190685372678459, 0.5302313826179257950, 0.7071067811865516806 ) ) ;
#5475=CARTESIAN_POINT ( 'NONE',  ( -18.05918829504999934, 10.97290950744599947, 62.14999999999999858 ) ) ;
#5476=CARTESIAN_POINT ( 'NONE',  ( -5.631644894983189431, 10.97290950744599947, 5.250000000000000000 ) ) ;
#5479=ORIENTED_EDGE ( 'NONE', *, *, #11052, .F. ) ;
#5483=VERTEX_POINT ( 'NONE', #11006 ) ;
#5485=DIRECTION ( 'NONE',  ( 0.000000000000000000, 0.000000000000000000, -1.000000000000000000 ) ) ;
#5486=AXIS2_PLACEMENT_3D ( 'NONE', #1890, #3025, #5086 ) ;
#5489=( LENGTH_UNIT ( ) NAMED_UNIT ( * ) SI_UNIT ( .MILLI., .METRE. ) );
#5492=DIRECTION ( 'NONE',  ( -1.000000000000000000, 0.000000000000000000, 0.000000000000000000 ) ) ;
#5494=ADVANCED_FACE ( 'NONE', ( #9735 ), #2496, .F. ) ;
#5495=VECTOR ( 'NONE', #4375, 1000.000000000000000 ) ;
#5496=CIRCLE ( 'NONE', #11104, 6.850000000000002309 ) ;
#5499=CARTESIAN_POINT ( 'NONE',  ( -15.45975122988422257, 30.21441468582782974, 54.15812869781769479 ) ) ;
#5500=ORIENTED_EDGE ( 'NONE', *, *, #10564, .T. ) ;
#5503=CARTESIAN_POINT ( 'NONE',  ( -11.74835982676941981, -4.028726038184999858, 62.14999999999999858 ) ) ;
#5505=LINE ( 'NONE', #7445, #9629 ) ;
#5506=EDGE_LOOP ( 'NONE', ( #1637, #6282, #3221, #7386, #9234 ) ) ;
#5509=DIRECTION ( 'NONE',  ( 0.000000000000000000, 0.000000000000000000, 1.000000000000000000 ) ) ;
#5512=VECTOR ( 'NONE', #11385, 1000.000000000000000 ) ;
#5518=DIRECTION ( 'NONE',  ( 0.000000000000000000, 0.000000000000000000, -1.000000000000000000 ) ) ;
#5519=ORIENTED_EDGE ( 'NONE', *, *, #8850, .T. ) ;
#5522=LINE ( 'NONE', #3387, #418 ) ;
#5523=DIRECTION ( 'NONE',  ( 1.000000000000000000, 0.000000000000000000, 0.000000000000000000 ) ) ;
#5525=LINE ( 'NONE', #6521, #10519 ) ;
#5527=DIRECTION ( 'NONE',  ( 0.000000000000000000, 0.000000000000000000, 1.000000000000000000 ) ) ;
#5528=CIRCLE ( 'NONE', #8895, 17.00000000000000355 ) ;
#5529=DIRECTION ( 'NONE',  ( 0.000000000000000000, 0.000000000000000000, 1.000000000000000000 ) ) ;
#5532=EDGE_CURVE ( 'NONE', #8353, #6343, #13233, .T. ) ;
#5534=DIRECTION ( 'NONE',  ( 0.000000000000000000, 0.000000000000000000, -1.000000000000000000 ) ) ;
#5535=VERTEX_POINT ( 'NONE', #12114 ) ;
#5536=EDGE_CURVE ( 'NONE', #8537, #12924, #10783, .T. ) ;
#5537=ORIENTED_EDGE ( 'NONE', *, *, #4424, .T. ) ;
#5542=EDGE_LOOP ( 'NONE', ( #9263, #6785, #13021, #1252 ) ) ;
#5545=DIRECTION ( 'NONE',  ( -1.000000000000000000, 0.000000000000000000, 0.000000000000000000 ) ) ;
#5546=DIRECTION ( 'NONE',  ( 1.000000000000000000, 0.000000000000000000, 0.000000000000000000 ) ) ;
#5548=CARTESIAN_POINT ( 'NONE',  ( -2.842019651049983331, 3.364325185445997679, 61.98378871700000303 ) ) ;
#5549=CARTESIAN_POINT ( 'NONE',  ( -35.05918829505000645, 27.97290950744599769, 58.85000000000000142 ) ) ;
#5551=CARTESIAN_POINT ( 'NONE',  ( -30.48673169511680214, 10.97290950744599947, 7.250000000000000000 ) ) ;
#5552=EDGE_LOOP ( 'NONE', ( #4530, #3955, #8101, #6972, #3715 ) ) ;
#5559=VERTEX_POINT ( 'NONE', #11066 ) ;
#5561=VERTEX_POINT ( 'NONE', #3799 ) ;
#5565=CIRCLE ( 'NONE', #2031, 7.618085573000000110 ) ;
#5566=AXIS2_PLACEMENT_3D ( 'NONE', #5956, #9261, #8073 ) ;
#5568=DIRECTION ( 'NONE',  ( 0.000000000000000000, 0.000000000000000000, 1.000000000000000000 ) ) ;
#5569=DIRECTION ( 'NONE',  ( -0.7071067811865500152, 8.659560562354959975E-17, 0.7071067811865450192 ) ) ;
#5572=AXIS2_PLACEMENT_3D ( 'NONE', #1824, #13679, #7108 ) ;
#5573=AXIS2_PLACEMENT_3D ( 'NONE', #11701, #5396, #6384 ) ;
#5575=CARTESIAN_POINT ( 'NONE',  ( -17.01680957860132537, 30.33693478204560989, 53.15683758623448085 ) ) ;
#5577=ADVANCED_FACE ( 'NONE', ( #1843 ), #10356, .F. ) ;
#5578=EDGE_CURVE ( 'NONE', #1000, #9989, #9247, .T. ) ;
#5579=VERTEX_POINT ( 'NONE', #7973 ) ;
#5585=CIRCLE ( 'NONE', #13398, 23.22993838181874793 ) ;
#5586=CONICAL_SURFACE ( 'NONE', #4274, 4.250000000000000000, 0.7853981633974518317 ) ;
#5588=CARTESIAN_POINT ( 'NONE',  ( -40.33164489498318517, 10.97290950744599947, 17.25000000000000000 ) ) ;
#5589=ORIENTED_EDGE ( 'NONE', *, *, #7839, .F. ) ;
#5590=AXIS2_PLACEMENT_3D ( 'NONE', #1744, #11454, #7040 ) ;
#5591=ORIENTED_EDGE ( 'NONE', *, *, #11274, .F. ) ;
#5593=CIRCLE ( 'NONE', #693, 17.66282263685195275 ) ;
#5595=VERTEX_POINT ( 'NONE', #11206 ) ;
#5596=EDGE_CURVE ( 'NONE', #586, #10750, #737, .T. ) ;
#5597=EDGE_LOOP ( 'NONE', ( #7049, #4290, #9346, #2768 ) ) ;
#5598=ORIENTED_EDGE ( 'NONE', *, *, #1847, .T. ) ;
#5601=CARTESIAN_POINT ( 'NONE',  ( -11.74835982676941981, -4.028726038184999858, 63.45000000000000284 ) ) ;
#5602=ORIENTED_EDGE ( 'NONE', *, *, #4784, .F. ) ;
#5603=EDGE_CURVE ( 'NONE', #3000, #12928, #11672, .T. ) ;
#5604=CARTESIAN_POINT ( 'NONE',  ( -18.05918829504999934, 10.97290950744599947, 61.25000000000000000 ) ) ;
#5605=DIRECTION ( 'NONE',  ( 0.000000000000000000, 0.000000000000000000, 1.000000000000000000 ) ) ;
#5606=FACE_BOUND ( 'NONE', #2967, .T. ) ;
#5608=CARTESIAN_POINT ( 'NONE',  ( -3.759188295049999518, 27.97290950744599769, 58.85000000000000142 ) ) ;
#5610=EDGE_CURVE ( 'NONE', #9493, #7236, #12569, .T. ) ;
#5611=CIRCLE ( 'NONE', #6287, 5.000000000000000888 ) ;
#5613=ORIENTED_EDGE ( 'NONE', *, *, #13379, .F. ) ;
#5614=ADVANCED_FACE ( 'NONE', ( #1560 ), #518, .F. ) ;
#5615=AXIS2_PLACEMENT_3D ( 'NONE', #4113, #4243, #2026 ) ;
#5618=LINE ( 'NONE', #4515, #12994 ) ;
#5620=CARTESIAN_POINT ( 'NONE',  ( -21.29502067386963304, 30.13379967401889203, 55.02888677376879656 ) ) ;
#5621=SURFACE_STYLE_USAGE ( .BOTH. , #6671 ) ;
#5625=CARTESIAN_POINT ( 'NONE',  ( -19.71317847370539766, 12.84756053868127879, 53.85000000000000142 ) ) ;
#5627=CARTESIAN_POINT ( 'NONE',  ( -25.73489962141544751, -4.139534227248430120, 61.65000000000000568 ) ) ;
#5629=CIRCLE ( 'NONE', #965, 8.300000000000000711 ) ;
#5630=EDGE_LOOP ( 'NONE', ( #974, #1082 ) ) ;
#5631=LINE ( 'NONE', #9912, #7452 ) ;
#5633=FACE_OUTER_BOUND ( 'NONE', #163, .T. ) ;
#5634=( NAMED_UNIT ( * ) SI_UNIT ( $, .STERADIAN. ) SOLID_ANGLE_UNIT ( ) );
#5637=LINE ( 'NONE', #11034, #6951 ) ;
#5638=FACE_OUTER_BOUND ( 'NONE', #10837, .T. ) ;
#5639=LINE ( 'NONE', #4542, #9843 ) ;
#5640=EDGE_CURVE ( 'NONE', #2414, #8708, #2096, .T. ) ;
#5643=AXIS2_PLACEMENT_3D ( 'NONE', #6897, #2599, #13320 ) ;
#5644=EDGE_LOOP ( 'NONE', ( #420, #10734, #6410, #6330 ) ) ;
#5645=ORIENTED_EDGE ( 'NONE', *, *, #4185, .F. ) ;
#5646=FACE_OUTER_BOUND ( 'NONE', #5552, .T. ) ;
#5647=VERTEX_POINT ( 'NONE', #10098 ) ;
#5648=DIRECTION ( 'NONE',  ( 1.000000000000000000, 0.000000000000000000, 0.000000000000000000 ) ) ;
#5653=DIRECTION ( 'NONE',  ( -0.6615960714621564875, 0.7498604124941129490, 0.000000000000000000 ) ) ;
#5654=ADVANCED_FACE ( 'NONE', ( #4780 ), #2909, .T. ) ;
#5655=EDGE_CURVE ( 'NONE', #9588, #8303, #2331, .T. ) ;
#5656=ORIENTED_EDGE ( 'NONE', *, *, #1753, .T. ) ;
#5657=EDGE_CURVE ( 'NONE', #6644, #1261, #969, .T. ) ;
#5659=DIRECTION ( 'NONE',  ( 0.000000000000000000, 1.000000000000000000, 0.000000000000000000 ) ) ;
#5660=ORIENTED_EDGE ( 'NONE', *, *, #8157, .F. ) ;
#5662=ORIENTED_EDGE ( 'NONE', *, *, #9557, .F. ) ;
#5663=VERTEX_POINT ( 'NONE', #9093 ) ;
#5665=ORIENTED_EDGE ( 'NONE', *, *, #10254, .F. ) ;
#5666=DIRECTION ( 'NONE',  ( -0.6615960714621564875, 0.7498604124941129490, 0.000000000000000000 ) ) ;
#5667=CARTESIAN_POINT ( 'NONE',  ( -17.37706816261102105, 26.95825899741793563, 56.01342904187733041 ) ) ;
#5669=DIRECTION ( 'NONE',  ( 0.000000000000000000, 0.000000000000000000, -1.000000000000000000 ) ) ;
#5670=EDGE_CURVE ( 'NONE', #1784, #3590, #1178, .T. ) ;
#5674=DIRECTION ( 'NONE',  ( -1.000000000000000000, 0.000000000000000000, 0.000000000000000000 ) ) ;
#5675=VERTEX_POINT ( 'NONE', #6997 ) ;
#5676=VECTOR ( 'NONE', #114, 1000.000000000000000 ) ;
#5677=CARTESIAN_POINT ( 'NONE',  ( -21.69765923394618667, 30.07360145807689733, 58.70649103051356121 ) ) ;
#5678=( NAMED_UNIT ( * ) PLANE_ANGLE_UNIT ( ) SI_UNIT ( $, .RADIAN. ) );
#5679=EDGE_LOOP ( 'NONE', ( #5739, #10634, #7247, #3155 ) ) ;
#5680=LINE ( 'NONE', #9959, #3538 ) ;
#5682=FACE_BOUND ( 'NONE', #1529, .T. ) ;
#5684=PRODUCT_DEFINITION_SHAPE ( 'NONE', 'NONE',  #7890 ) ;
#5686=EDGE_CURVE ( 'NONE', #6919, #9237, #8725, .T. ) ;
#5688=VECTOR ( 'NONE', #12827, 1000.000000000000000 ) ;
#5689=VERTEX_POINT ( 'NONE', #2251 ) ;
#5693=DIRECTION ( 'NONE',  ( 0.000000000000000000, 0.000000000000000000, -1.000000000000000000 ) ) ;
#5694=EDGE_LOOP ( 'NONE', ( #8368, #7530 ) ) ;
#5696=SURFACE_STYLE_FILL_AREA ( #13312 ) ;
#5697=CARTESIAN_POINT ( 'NONE',  ( -5.309188295050000228, 27.97290950744599769, 58.85000000000000142 ) ) ;
#5698=FACE_OUTER_BOUND ( 'NONE', #13598, .T. ) ;
#5699=CARTESIAN_POINT ( 'NONE',  ( -18.05918829504999934, 10.97290950744599947, 53.85000000000000142 ) ) ;
#5702=CARTESIAN_POINT ( 'NONE',  ( -10.78334210919089919, 29.19143287883919768, 64.85000000000000853 ) ) ;
#5703=CIRCLE ( 'NONE', #7925, 16.72262947720610171 ) ;
#5704=FACE_BOUND ( 'NONE', #5630, .T. ) ;
#5705=LINE ( 'NONE', #9006, #8224 ) ;
#5706=EDGE_CURVE ( 'NONE', #506, #87, #8538, .T. ) ;
#5707=EDGE_CURVE ( 'NONE', #8370, #11045, #12594, .T. ) ;
#5708=EDGE_LOOP ( 'NONE', ( #5731, #10396, #9824, #13278 ) ) ;
#5709=VECTOR ( 'NONE', #2054, 1000.000000000000114 ) ;
#5713=ORIENTED_EDGE ( 'NONE', *, *, #8545, .T. ) ;
#5717=FACE_OUTER_BOUND ( 'NONE', #1832, .T. ) ;
#5718=CARTESIAN_POINT ( 'NONE',  ( -18.05918829504999934, 10.97290950744599947, 61.65955166399999854 ) ) ;
#5719=AXIS2_PLACEMENT_3D ( 'NONE', #4692, #9070, #5648 ) ;
#5720=CARTESIAN_POINT ( 'NONE',  ( -18.05918829504999934, 10.97290950744599947, 30.59999999999999787 ) ) ;
#5721=VERTEX_POINT ( 'NONE', #1909 ) ;
#5723=EDGE_LOOP ( 'NONE', ( #6363, #13273, #10378, #8766 ) ) ;
#5724=DIRECTION ( 'NONE',  ( 0.000000000000000000, 0.000000000000000000, 1.000000000000000000 ) ) ;
#5725=EDGE_LOOP ( 'NONE', ( #509, #10764, #3789, #3102, #3409 ) ) ;
#5728=DIRECTION ( 'NONE',  ( 1.000000000000000000, 0.000000000000000000, 0.000000000000000000 ) ) ;
#5729=EDGE_CURVE ( 'NONE', #5077, #10024, #2780, .T. ) ;
#5730=CARTESIAN_POINT ( 'NONE',  ( -11.91335496205000055, 10.97290950744599947, 60.60999999999999943 ) ) ;
#5731=ORIENTED_EDGE ( 'NONE', *, *, #8691, .F. ) ;
#5732=CARTESIAN_POINT ( 'NONE',  ( -11.75918829505000041, 10.97290950744599947, 63.02000000000000313 ) ) ;
#5733=CARTESIAN_POINT ( 'NONE',  ( -12.00918829505000041, 10.97290950744599947, 64.85000000000000853 ) ) ;
#5734=DIRECTION ( 'NONE',  ( 0.000000000000000000, 0.000000000000000000, -1.000000000000000000 ) ) ;
#5735=DIRECTION ( 'NONE',  ( 0.4528443260392610026, 0.8915896008669278450, 0.000000000000000000 ) ) ;
#5737=CIRCLE ( 'NONE', #13549, 4.750000000000000888 ) ;
#5739=ORIENTED_EDGE ( 'NONE', *, *, #10464, .F. ) ;
#5741=ADVANCED_FACE ( 'NONE', ( #10496 ), #8998, .F. ) ;
#5743=ORIENTED_EDGE ( 'NONE', *, *, #2016, .T. ) ;
#5744=CIRCLE ( 'NONE', #9097, 16.95000000000000284 ) ;
#5747=EDGE_CURVE ( 'NONE', #11638, #1281, #11233, .T. ) ;
#5750=CARTESIAN_POINT ( 'NONE',  ( -20.72664669423063089, 30.20666037455253061, 60.46838943485088436 ) ) ;
#5751=DIRECTION ( 'NONE',  ( 0.000000000000000000, 0.000000000000000000, 1.000000000000000000 ) ) ;
#5752=DIRECTION ( 'NONE',  ( -1.000000000000000000, 0.000000000000000000, 0.000000000000000000 ) ) ;
#5753=CARTESIAN_POINT ( 'NONE',  ( -23.41085226126194740, -11.41022146549009975, 64.85000000000000853 ) ) ;
#5754=DIRECTION ( 'NONE',  ( 0.000000000000000000, 0.000000000000000000, 1.000000000000000000 ) ) ;
#5755=LINE ( 'NONE', #9837, #6234 ) ;
#5759=CIRCLE ( 'NONE', #9570, 6.450000000000009948 ) ;
#5761=AXIS2_PLACEMENT_3D ( 'NONE', #6929, #781, #11268 ) ;
#5764=CARTESIAN_POINT ( 'NONE',  ( -35.05918829505000645, -6.027090492554000534, 58.85000000000000142 ) ) ;
#5772=CARTESIAN_POINT ( 'NONE',  ( -1.059188295049996231, -6.027090492554000534, 5.250000000000000000 ) ) ;
#5773=CARTESIAN_POINT ( 'NONE',  ( -5.631644894983189431, 10.97290950744599947, 17.25000000000000000 ) ) ;
#5775=ADVANCED_FACE ( 'NONE', ( #11876 ), #6082, .T. ) ;
#5777=AXIS2_PLACEMENT_3D ( 'NONE', #2913, #3804, #9035 ) ;
#5778=PLANE ( 'NONE',  #10017 ) ;
#5779=ADVANCED_FACE ( 'NONE', ( #4397 ), #8331, .F. ) ;
#5781=AXIS2_PLACEMENT_3D ( 'NONE', #6734, #2566, #11067 ) ;
#5782=VERTEX_POINT ( 'NONE', #7587 ) ;
#5783=DIRECTION ( 'NONE',  ( 0.000000000000000000, 0.000000000000000000, -1.000000000000000000 ) ) ;
#5785=EDGE_CURVE ( 'NONE', #918, #2345, #13560, .T. ) ;
#5786=ORIENTED_EDGE ( 'NONE', *, *, #11186, .F. ) ;
#5789=CARTESIAN_POINT ( 'NONE',  ( -18.05918829504999934, 10.00028003023991907, 62.14999999999999858 ) ) ;
#5790=CARTESIAN_POINT ( 'NONE',  ( -41.50918829505000218, 27.97290950744599769, 17.25000000000000000 ) ) ;
#5792=CARTESIAN_POINT ( 'NONE',  ( -1.059188295049996231, -6.027090492554000534, 17.25000000000000000 ) ) ;
#5794=DIRECTION ( 'NONE',  ( 0.000000000000000000, 0.000000000000000000, -1.000000000000000000 ) ) ;
#5795=VECTOR ( 'NONE', #13481, 1000.000000000000000 ) ;
#5797=DIRECTION ( 'NONE',  ( 0.000000000000000000, 0.000000000000000000, 1.000000000000000000 ) ) ;
#5798=VERTEX_POINT ( 'NONE', #8574 ) ;
#5799=AXIS2_PLACEMENT_3D ( 'NONE', #13586, #4037, #8292 ) ;
#5800=EDGE_LOOP ( 'NONE', ( #3385, #8533, #8962, #10638 ) ) ;
#5801=AXIS2_PLACEMENT_3D ( 'NONE', #2735, #12208, #3564 ) ;
#5803=FACE_OUTER_BOUND ( 'NONE', #11478, .T. ) ;
#5804=CIRCLE ( 'NONE', #10968, 16.00000000000000000 ) ;
#5805=ORIENTED_EDGE ( 'NONE', *, *, #2482, .F. ) ;
#5806=CARTESIAN_POINT ( 'NONE',  ( -33.27635693905001801, 18.58149382944601058, 61.98378871700000303 ) ) ;
#5807=LINE ( 'NONE', #13078, #10233 ) ;
#5809=CARTESIAN_POINT ( 'NONE',  ( -18.05918829430469685, 19.27290950744890097, 63.15000000009349179 ) ) ;
#5813=FACE_BOUND ( 'NONE', #6012, .T. ) ;
#5815=AXIS2_PLACEMENT_3D ( 'NONE', #5974, #13255, #3695 ) ;
#5816=ORIENTED_EDGE ( 'NONE', *, *, #2180, .T. ) ;
#5817=VERTEX_POINT ( 'NONE', #849 ) ;
#5818=CARTESIAN_POINT ( 'NONE',  ( -18.05918829504999934, 10.97290950744599947, 57.35000000000000142 ) ) ;
#5820=DIRECTION ( 'NONE',  ( 0.000000000000000000, 0.000000000000000000, -1.000000000000000000 ) ) ;
#5821=CARTESIAN_POINT ( 'NONE',  ( -21.24216064964741690, 30.14123926836247591, 59.76621780875206014 ) ) ;
#5823=AXIS2_PLACEMENT_3D ( 'NONE', #3408, #13788, #7701 ) ;
#5826=AXIS2_PLACEMENT_3D ( 'NONE', #5954, #460, #1708 ) ;
#5831=EDGE_CURVE ( 'NONE', #13422, #11802, #5183, .T. ) ;
#5833=STYLED_ITEM ( 'NONE', ( #7435 ), #4601 ) ;
#5834=EDGE_CURVE ( 'NONE', #10854, #7101, #1189, .T. ) ;
#5837=FACE_OUTER_BOUND ( 'NONE', #12513, .T. ) ;
#5838=VERTEX_POINT ( 'NONE', #9922 ) ;
#5839=CARTESIAN_POINT ( 'NONE',  ( -35.05918829505000645, 27.97290950744599769, 5.250000000000000000 ) ) ;
#5840=CARTESIAN_POINT ( 'NONE',  ( -18.05918829504999934, 10.97290950744599947, 60.85000000000000142 ) ) ;
#5841=CARTESIAN_POINT ( 'NONE',  ( -18.05918829504999934, 10.97290950744599947, 53.85000000000000142 ) ) ;
#5844=DIRECTION ( 'NONE',  ( 0.000000000000000000, 0.000000000000000000, -1.000000000000000000 ) ) ;
#5846=CIRCLE ( 'NONE', #2077, 24.92993838181874722 ) ;
#5849=ADVANCED_FACE ( 'NONE', ( #8793 ), #11101, .T. ) ;
#5850=EDGE_LOOP ( 'NONE', ( #2707, #11125 ) ) ;
#5853=AXIS2_PLACEMENT_3D ( 'NONE', #4635, #5527, #11904 ) ;
#5854=CARTESIAN_POINT ( 'NONE',  ( -20.70557258089865016, 13.97235115742243927, 30.59999999999999787 ) ) ;
#5855=ORIENTED_EDGE ( 'NONE', *, *, #10569, .F. ) ;
#5857=CARTESIAN_POINT ( 'NONE',  ( -16.60019635188397658, 27.03346355975618565, 56.97665238683693190 ) ) ;
#5859=DIRECTION ( 'NONE',  ( 0.000000000000000000, 0.000000000000000000, -1.000000000000000000 ) ) ;
#5861=CARTESIAN_POINT ( 'NONE',  ( -18.05918829504999934, 10.97290950744599947, 60.60999999999999943 ) ) ;
#5862=FACE_OUTER_BOUND ( 'NONE', #9661, .T. ) ;
#5863=CARTESIAN_POINT ( 'NONE',  ( -1.059188295049996231, 27.97290950744599769, 7.250000000000000000 ) ) ;
#5864=AXIS2_PLACEMENT_3D ( 'NONE', #11133, #13227, #4914 ) ;
#5865=EDGE_CURVE ( 'NONE', #7102, #1633, #12579, .T. ) ;
#5866=ORIENTED_EDGE ( 'NONE', *, *, #2244, .F. ) ;
#5867=EDGE_CURVE ( 'NONE', #533, #2781, #8550, .T. ) ;
#5868=ORIENTED_EDGE ( 'NONE', *, *, #6387, .F. ) ;
#5875=ORIENTED_EDGE ( 'NONE', *, *, #2829, .T. ) ;
#5876=CARTESIAN_POINT ( 'NONE',  ( -15.54654308236029792, 19.85770471824265115, 64.85000000000000853 ) ) ;
#5879=CYLINDRICAL_SURFACE ( 'NONE', #9414, 1.725000000000000755 ) ;
#5880=CARTESIAN_POINT ( 'NONE',  ( -18.05918829504999934, 10.97290950744599947, 116.8499999999999943 ) ) ;
#5883=EDGE_CURVE ( 'NONE', #8303, #936, #11460, .T. ) ;
#5886=ORIENTED_EDGE ( 'NONE', *, *, #2760, .T. ) ;
#5889=DIRECTION ( 'NONE',  ( 0.000000000000000000, 0.000000000000000000, 1.000000000000000000 ) ) ;
#5890=CARTESIAN_POINT ( 'NONE',  ( -21.06699515661435029, 30.16479851496719533, 60.03871598454315262 ) ) ;
#5894=DIRECTION ( 'NONE',  ( -1.000000000000000000, 0.000000000000000000, 0.000000000000000000 ) ) ;
#5895=ORIENTED_EDGE ( 'NONE', *, *, #2502, .T. ) ;
#5896=AXIS2_PLACEMENT_3D ( 'NONE', #2115, #3289, #1041 ) ;
#5899=FACE_OUTER_BOUND ( 'NONE', #8075, .T. ) ;
#5905=CARTESIAN_POINT ( 'NONE',  ( 1.640811704950005057, -6.027090492554000534, 7.250000000000000000 ) ) ;
#5906=DIRECTION ( 'NONE',  ( -1.000000000000000000, 0.000000000000000000, 0.000000000000000000 ) ) ;
#5907=DIRECTION ( 'NONE',  ( 1.000000000000000000, 0.000000000000000000, 0.000000000000000000 ) ) ;
#5912=AXIS2_PLACEMENT_3D ( 'NONE', #11730, #5368, #9647 ) ;
#5914=DIRECTION ( 'NONE',  ( 0.000000000000000000, 0.000000000000000000, -1.000000000000000000 ) ) ;
#5915=ORIENTED_EDGE ( 'NONE', *, *, #3856, .T. ) ;
#5922=CARTESIAN_POINT ( 'NONE',  ( -18.05918829504999934, 19.27191034044600215, 63.13003331699999876 ) ) ;
#5923=DIRECTION ( 'NONE',  ( 0.000000000000000000, 0.000000000000000000, -1.000000000000000000 ) ) ;
#5926=CARTESIAN_POINT ( 'NONE',  ( -17.29478376989774446, 30.34769730472564930, 61.62036986256358517 ) ) ;
#5928=ORIENTED_EDGE ( 'NONE', *, *, #7644, .T. ) ;
#5929=CYLINDRICAL_SURFACE ( 'NONE', #10045, 34.69999999999999574 ) ;
#5930=DIRECTION ( 'NONE',  ( 0.000000000000000000, 0.000000000000000000, -1.000000000000000000 ) ) ;
#5934=DIRECTION ( 'NONE',  ( 0.000000000000000000, 0.000000000000000000, -1.000000000000000000 ) ) ;
#5935=EDGE_CURVE ( 'NONE', #6071, #10428, #9232, .T. ) ;
#5937=AXIS2_PLACEMENT_3D ( 'NONE', #11734, #2185, #6424 ) ;
#5941=DIRECTION ( 'NONE',  ( -0.000000000000000000, -0.000000000000000000, 1.000000000000000000 ) ) ;
#5943=EDGE_CURVE ( 'NONE', #11802, #12100, #3009, .T. ) ;
#5944=ORIENTED_EDGE ( 'NONE', *, *, #11452, .T. ) ;
#5947=CARTESIAN_POINT ( 'NONE',  ( -41.50918829505000218, -6.027090492554000534, 17.25000000000000000 ) ) ;
#5949=CARTESIAN_POINT ( 'NONE',  ( -20.39103306562181928, 30.24295657639994772, 60.79987120566779879 ) ) ;
#5950=CIRCLE ( 'NONE', #2872, 6.299999999999998046 ) ;
#5952=CIRCLE ( 'NONE', #13761, 0.9499999999999995115 ) ;
#5953=DIRECTION ( 'NONE',  ( -0.000000000000000000, -0.000000000000000000, 1.000000000000000000 ) ) ;
#5954=CARTESIAN_POINT ( 'NONE',  ( -18.05918829504999934, 10.97290950744599947, 58.54999999999999716 ) ) ;
#5956=CARTESIAN_POINT ( 'NONE',  ( -24.37001676333060018, -4.028726038184999858, 62.14999999999999858 ) ) ;
#5965=ORIENTED_EDGE ( 'NONE', *, *, #6812, .F. ) ;
#5967=LINE ( 'NONE', #9270, #3148 ) ;
#5968=CARTESIAN_POINT ( 'NONE',  ( -18.05918829504999934, 10.97290950744599947, 63.64999999999999858 ) ) ;
#5971=DIRECTION ( 'NONE',  ( 0.000000000000000000, 0.000000000000000000, -1.000000000000000000 ) ) ;
#5974=CARTESIAN_POINT ( 'NONE',  ( -1.059188295049996231, 27.97290950744599769, 5.250000000000000000 ) ) ;
#5976=DIRECTION ( 'NONE',  ( 0.000000000000000000, 0.000000000000000000, 1.000000000000000000 ) ) ;
#5978=AXIS2_PLACEMENT_3D ( 'NONE', #1418, #6852, #10225 ) ;
#5979=CIRCLE ( 'NONE', #10240, 4.250000000000000000 ) ;
#5981=ADVANCED_FACE ( 'NONE', ( #5704, #4806 ), #409, .F. ) ;
#5983=ORIENTED_EDGE ( 'NONE', *, *, #469, .F. ) ;
#5987=PRODUCT_DEFINITION_FORMATION_WITH_SPECIFIED_SOURCE ( 'ANY', '', #12935, .NOT_KNOWN. ) ;
#5988=AXIS2_PLACEMENT_3D ( 'NONE', #11886, #6567, #7446 ) ;
#5992=AXIS2_PLACEMENT_3D ( 'NONE', #10039, #4656, #4582 ) ;
#5995=LINE ( 'NONE', #766, #2451 ) ;
#5996=CARTESIAN_POINT ( 'NONE',  ( -10.47404583389237942, 25.90703532196704728, 57.35000000000000142 ) ) ;
#5997=FACE_OUTER_BOUND ( 'NONE', #7534, .T. ) ;
#5999=AXIS2_PLACEMENT_3D ( 'NONE', #30, #5395, #9675 ) ;
#6000=AXIS2_PLACEMENT_3D ( 'NONE', #4048, #8299, #12564 ) ;
#6001=EDGE_CURVE ( 'NONE', #5058, #7296, #13457, .T. ) ;
#6002=EDGE_CURVE ( 'NONE', #1128, #1821, #9277, .T. ) ;
#6003=ORIENTED_EDGE ( 'NONE', *, *, #12890, .T. ) ;
#6004=CARTESIAN_POINT ( 'NONE',  ( -15.56809582730673647, 30.22631440468149222, 60.65219431213508727 ) ) ;
#6005=ORIENTED_EDGE ( 'NONE', *, *, #4255, .T. ) ;
#6012=EDGE_LOOP ( 'NONE', ( #11748, #13213 ) ) ;
#6013=DIRECTION ( 'NONE',  ( 0.000000000000000000, 0.000000000000000000, 1.000000000000000000 ) ) ;
#6015=DIRECTION ( 'NONE',  ( 0.000000000000000000, 0.000000000000000000, -1.000000000000000000 ) ) ;
#6016=AXIS2_PLACEMENT_3D ( 'NONE', #12873, #93, #1072 ) ;
#6017=EDGE_LOOP ( 'NONE', ( #13644, #9966 ) ) ;
#6018=CARTESIAN_POINT ( 'NONE',  ( -1.396365658198039927, 10.97290950744599947, 5.250000000000000000 ) ) ;
#6020=ORIENTED_EDGE ( 'NONE', *, *, #4436, .F. ) ;
#6021=ORIENTED_EDGE ( 'NONE', *, *, #10161, .T. ) ;
#6023=AXIS2_PLACEMENT_3D ( 'NONE', #8007, #10380, #10186 ) ;
#6025=CIRCLE ( 'NONE', #10, 1.000000000000000000 ) ;
#6026=AXIS2_PLACEMENT_3D ( 'NONE', #6895, #11037, #545 ) ;
#6028=FACE_OUTER_BOUND ( 'NONE', #5679, .T. ) ;
#6031=DIRECTION ( 'NONE',  ( 0.000000000000000000, 0.000000000000000000, -1.000000000000000000 ) ) ;
#6033=DIRECTION ( 'NONE',  ( 0.000000000000000000, 0.000000000000000000, -1.000000000000000000 ) ) ;
#6035=VECTOR ( 'NONE', #4192, 1000.000000000000000 ) ;
#6037=ORIENTED_EDGE ( 'NONE', *, *, #5657, .F. ) ;
#6039=ORIENTED_EDGE ( 'NONE', *, *, #1566, .F. ) ;
#6040=EDGE_CURVE ( 'NONE', #6370, #9883, #1415, .T. ) ;
#6041=ORIENTED_EDGE ( 'NONE', *, *, #1348, .F. ) ;
#6044=CIRCLE ( 'NONE', #1142, 6.449999999999997513 ) ;
#6050=CARTESIAN_POINT ( 'NONE',  ( -18.05918829504999934, 10.97290950744599947, 60.04999999999999716 ) ) ;
#6051=CARTESIAN_POINT ( 'NONE',  ( -23.85417428574490373, 12.52794563810342154, 67.84999999999999432 ) ) ;
#6052=VERTEX_POINT ( 'NONE', #8363 ) ;
#6053=DIRECTION ( 'NONE',  ( 0.000000000000000000, 0.000000000000000000, -1.000000000000000000 ) ) ;
#6054=DIRECTION ( 'NONE',  ( 1.000000000000000000, 0.000000000000000000, 0.000000000000000000 ) ) ;
#6060=VERTEX_POINT ( 'NONE', #11441 ) ;
#6061=LINE ( 'NONE', #10335, #5688 ) ;
#6063=ADVANCED_FACE ( 'NONE', ( #3842, #9216 ), #11506, .T. ) ;
#6064=AXIS2_PLACEMENT_3D ( 'NONE', #457, #5751, #5546 ) ;
#6065=CARTESIAN_POINT ( 'NONE',  ( -22.64501676333060232, -4.028726038184999858, 62.14999999999999858 ) ) ;
#6066=CARTESIAN_POINT ( 'NONE',  ( -35.05918829505000645, 27.97290950744599769, 83.57661607529820458 ) ) ;
#6068=DIRECTION ( 'NONE',  ( 0.000000000000000000, 3.387121092260455192E-15, 1.000000000000000000 ) ) ;
#6069=CARTESIAN_POINT ( 'NONE',  ( -12.87735031270726083, -6.265087914666300328, 62.14999999999999858 ) ) ;
#6070=VECTOR ( 'NONE', #7147, 1000.000000000000114 ) ;
#6071=VERTEX_POINT ( 'NONE', #6184 ) ;
#6072=VERTEX_POINT ( 'NONE', #10458 ) ;
#6073=CARTESIAN_POINT ( 'NONE',  ( -15.68396707275562463, 30.23850757421161006, 60.76113458392060096 ) ) ;
#6075=CARTESIAN_POINT ( 'NONE',  ( -35.05918829505000645, 27.97290950744599769, 17.25000000000000000 ) ) ;
#6076=CARTESIAN_POINT ( 'NONE',  ( -5.631644894983189431, 10.97290950744599947, 73.76763816269230745 ) ) ;
#6079=PLANE ( 'NONE',  #5761 ) ;
#6081=CARTESIAN_POINT ( 'NONE',  ( -1.059188295049996231, -6.027090492554000534, 58.85000000000000142 ) ) ;
#6082=CONICAL_SURFACE ( 'NONE', #64, 16.75000000000000355, 0.7853981633974447263 ) ;
#6083=DIRECTION ( 'NONE',  ( 0.9496839325805432885, -0.3132098788326352912, 0.000000000000000000 ) ) ;
#6086=EDGE_CURVE ( 'NONE', #12239, #4997, #11909, .T. ) ;
#6087=DIRECTION ( 'NONE',  ( 0.000000000000000000, 0.000000000000000000, -1.000000000000000000 ) ) ;
#6090=VERTEX_POINT ( 'NONE', #7291 ) ;
#6091=EDGE_LOOP ( 'NONE', ( #2204, #13020, #12895, #12427 ) ) ;
#6092=ORIENTED_EDGE ( 'NONE', *, *, #9515, .T. ) ;
#6093=ORIENTED_EDGE ( 'NONE', *, *, #3377, .F. ) ;
#6094=LINE ( 'NONE', #5947, #6188 ) ;
#6095=CARTESIAN_POINT ( 'NONE',  ( -19.65133266638497389, 30.30564942401206352, 61.31020756158706320 ) ) ;
#6096=DIRECTION ( 'NONE',  ( 1.000000000000000000, 0.000000000000000000, 0.000000000000000000 ) ) ;
#6097=CARTESIAN_POINT ( 'NONE',  ( 3.190811704950004657, -6.027090492554000534, 64.35000000000000853 ) ) ;
#6098=FACE_OUTER_BOUND ( 'NONE', #12445, .T. ) ;
#6102=ORIENTED_EDGE ( 'NONE', *, *, #1864, .F. ) ;
#6107=VERTEX_POINT ( 'NONE', #12360 ) ;
#6108=DIRECTION ( 'NONE',  ( -1.000000000000000000, 0.000000000000000000, 0.000000000000000000 ) ) ;
#6109=CARTESIAN_POINT ( 'NONE',  ( -16.55918829504999579, 21.47290950744600124, 57.35000000000000142 ) ) ;
#6112=DIRECTION ( 'NONE',  ( 0.000000000000000000, 0.000000000000000000, 1.000000000000000000 ) ) ;
#6113=CYLINDRICAL_SURFACE ( 'NONE', #419, 6.000000000000002665 ) ;
#6114=LINE ( 'NONE', #7226, #11184 ) ;
#6117=DIRECTION ( 'NONE',  ( 0.6615960714621574867, -0.7498604124941119498, 0.000000000000000000 ) ) ;
#6119=ADVANCED_FACE ( 'NONE', ( #2871 ), #13243, .T. ) ;
#6120=CIRCLE ( 'NONE', #10826, 4.250000000000000000 ) ;
#6122=CARTESIAN_POINT ( 'NONE',  ( -32.35918829505000360, 27.97290950744599769, 64.85000000000000853 ) ) ;
#6124=CLOSED_SHELL ( 'NONE', ( #7365, #7182, #5849, #3477, #8176, #4346, #1319, #4585, #239, #11017, #10364, #9928, #35, #8817, #10475, #421, #12249 ) ) ;
#6126=VERTEX_POINT ( 'NONE', #7094 ) ;
#6127=CARTESIAN_POINT ( 'NONE',  ( -18.88016301897669891, 16.91647750172969822, 67.84999999999999432 ) ) ;
#6130=ORIENTED_EDGE ( 'NONE', *, *, #1950, .T. ) ;
#6138=CARTESIAN_POINT ( 'NONE',  ( -14.51101483699455841, 30.08769857173034623, 58.98207106897987728 ) ) ;
#6140=CARTESIAN_POINT ( 'NONE',  ( -15.54512322349380149, 8.123439939968370993, 27.09999999999999787 ) ) ;
#6144=ORIENTED_EDGE ( 'NONE', *, *, #11475, .F. ) ;
#6145=DIRECTION ( 'NONE',  ( 1.000000000000000000, 0.000000000000000000, 0.000000000000000000 ) ) ;
#6146=DIRECTION ( 'NONE',  ( 0.000000000000000000, 0.000000000000000000, -1.000000000000000000 ) ) ;
#6147=ORIENTED_EDGE ( 'NONE', *, *, #8978, .T. ) ;
#6151=AXIS2_PLACEMENT_3D ( 'NONE', #10485, #7187, #7249 ) ;
#6152=LINE ( 'NONE', #10424, #1804 ) ;
#6154=VERTEX_POINT ( 'NONE', #5346 ) ;
#6155=ORIENTED_EDGE ( 'NONE', *, *, #9908, .F. ) ;
#6156=ADVANCED_FACE ( 'NONE', ( #5275 ), #1783, .F. ) ;
#6158=ORIENTED_EDGE ( 'NONE', *, *, #10479, .T. ) ;
#6159=CIRCLE ( 'NONE', #10407, 2.700000000000000178 ) ;
#6160=LINE ( 'NONE', #8272, #3987 ) ;
#6162=DIRECTION ( 'NONE',  ( -1.000000000000000000, 0.000000000000000000, 0.000000000000000000 ) ) ;
#6168=ORIENTED_EDGE ( 'NONE', *, *, #1866, .F. ) ;
#6170=MECHANICAL_DESIGN_GEOMETRIC_PRESENTATION_REPRESENTATION('',(#4629),#2637);
#6171=EDGE_CURVE ( 'NONE', #2279, #1108, #653, .T. ) ;
#6173=CARTESIAN_POINT ( 'NONE',  ( -35.05918829505000645, -6.027090492554000534, 17.25000000000000000 ) ) ;
#6174=ORIENTED_EDGE ( 'NONE', *, *, #10960, .F. ) ;
#6176=CARTESIAN_POINT ( 'NONE',  ( -1.059188295049996231, 27.97290950744599769, 64.35000000000000853 ) ) ;
#6177=CIRCLE ( 'NONE', #10000, 3.000000000000001332 ) ;
#6181=CARTESIAN_POINT ( 'NONE',  ( -18.05918829504999934, 10.97290950744599947, 60.40999999999999659 ) ) ;
#6183=CARTESIAN_POINT ( 'NONE',  ( -35.05918829505000645, 27.97290950744599769, 5.250000000000000000 ) ) ;
#6184=CARTESIAN_POINT ( 'NONE',  ( -1.059188295049996231, 10.97290950744599947, 63.54999999999999716 ) ) ;
#6185=FACE_OUTER_BOUND ( 'NONE', #1553, .T. ) ;
#6186=CIRCLE ( 'NONE', #13548, 8.395833332999998788 ) ;
#6187=ORIENTED_EDGE ( 'NONE', *, *, #2034, .F. ) ;
#6188=VECTOR ( 'NONE', #1704, 1000.000000000000000 ) ;
#6189=ORIENTED_EDGE ( 'NONE', *, *, #10641, .F. ) ;
#6191=CARTESIAN_POINT ( 'NONE',  ( -28.87730642030695094, 29.81324547859994922, 5.250000000000000000 ) ) ;
#6194=DIRECTION ( 'NONE',  ( 1.000000000000000000, 0.000000000000000000, 0.000000000000000000 ) ) ;
#6198=AXIS2_PLACEMENT_3D ( 'NONE', #4544, #2113, #6351 ) ;
#6200=CONICAL_SURFACE ( 'NONE', #178, 6.145833333000002341, 0.2014252309328122270 ) ;
#6201=CIRCLE ( 'NONE', #10904, 2.700000000000001066 ) ;
#6203=AXIS2_PLACEMENT_3D ( 'NONE', #2595, #3637, #12211 ) ;
#6205=DIRECTION ( 'NONE',  ( 1.000000000000000000, 0.000000000000000000, 0.000000000000000000 ) ) ;
#6207=VECTOR ( 'NONE', #4405, 1000.000000000000114 ) ;
#6211=VECTOR ( 'NONE', #5341, 1000.000000000000227 ) ;
#6212=CARTESIAN_POINT ( 'NONE',  ( -15.33453732926608915, 30.19994085548103513, 60.40352641156652425 ) ) ;
#6213=EDGE_LOOP ( 'NONE', ( #4739, #6238, #4134, #7824 ) ) ;
#6214=EDGE_LOOP ( 'NONE', ( #2373, #2709, #4293, #12257 ) ) ;
#6215=ORIENTED_EDGE ( 'NONE', *, *, #5747, .T. ) ;
#6216=CARTESIAN_POINT ( 'NONE',  ( -1.059188295049996231, -6.027090492554000534, 83.57661607529820458 ) ) ;
#6219=ORIENTED_EDGE ( 'NONE', *, *, #8920, .T. ) ;
#6220=DIRECTION ( 'NONE',  ( 0.000000000000000000, 0.000000000000000000, -1.000000000000000000 ) ) ;
#6221=DIRECTION ( 'NONE',  ( 0.000000000000000000, 0.000000000000000000, -1.000000000000000000 ) ) ;
#6224=DIRECTION ( 'NONE',  ( 0.000000000000000000, 0.000000000000000000, -1.000000000000000000 ) ) ;
#6226=CARTESIAN_POINT ( 'NONE',  ( 8.157609394192110841, 24.73469418910620021, 17.25000000000000000 ) ) ;
#6228=DIRECTION ( 'NONE',  ( 0.000000000000000000, -1.000000000000000000, 0.000000000000000000 ) ) ;
#6231=ORIENTED_EDGE ( 'NONE', *, *, #3526, .T. ) ;
#6233=ORIENTED_EDGE ( 'NONE', *, *, #13648, .F. ) ;
#6234=VECTOR ( 'NONE', #10954, 1000.000000000000000 ) ;
#6236=LINE ( 'NONE', #7406, #2437 ) ;
#6238=ORIENTED_EDGE ( 'NONE', *, *, #3847, .T. ) ;
#6240=CARTESIAN_POINT ( 'NONE',  ( -18.05918829504999934, 10.97290950744599947, 30.59999999999999787 ) ) ;
#6241=CARTESIAN_POINT ( 'NONE',  ( -18.93268260677970716, 26.94904914358915704, 56.13056362116011400 ) ) ;
#6242=DIRECTION ( 'NONE',  ( 0.3132098788326365124, -0.9496839325805429555, 0.000000000000000000 ) ) ;
#6246=EDGE_LOOP ( 'NONE', ( #8633, #1976 ) ) ;
#6249=VECTOR ( 'NONE', #2609, 1000.000000000000000 ) ;
#6251=AXIS2_PLACEMENT_3D ( 'NONE', #3764, #9138, #2665 ) ;
#6258=DIRECTION ( 'NONE',  ( 0.000000000000000000, 0.000000000000000000, -1.000000000000000000 ) ) ;
#6259=DIRECTION ( 'NONE',  ( 0.000000000000000000, 0.000000000000000000, -1.000000000000000000 ) ) ;
#6260=AXIS2_PLACEMENT_3D ( 'NONE', #12654, #11604, #7053 ) ;
#6261=AXIS2_PLACEMENT_3D ( 'NONE', #8376, #10547, #977 ) ;
#6263=CARTESIAN_POINT ( 'NONE',  ( -18.05918829504999934, 7.130333642789880244, 5.250000000000000000 ) ) ;
#6265=AXIS2_PLACEMENT_3D ( 'NONE', #9705, #3493, #12904 ) ;
#6266=DIRECTION ( 'NONE',  ( 1.000000000000000000, 0.000000000000000000, 0.000000000000000000 ) ) ;
#6267=DIRECTION ( 'NONE',  ( 0.000000000000000000, 0.000000000000000000, -1.000000000000000000 ) ) ;
#6270=ADVANCED_FACE ( 'NONE', ( #11777 ), #2097, .T. ) ;
#6271=EDGE_CURVE ( 'NONE', #3389, #13286, #10597, .T. ) ;
#6272=ORIENTED_EDGE ( 'NONE', *, *, #8868, .F. ) ;
#6275=AXIS2_PLACEMENT_3D ( 'NONE', #5150, #11504, #9484 ) ;
#6276=EDGE_LOOP ( 'NONE', ( #2131, #5886, #3097, #1094, #8797, #3384, #5048, #13122, #11894, #5284, #3096, #4531, #2317, #5103, #2525 ) ) ;
#6278=DIRECTION ( 'NONE',  ( 0.000000000000000000, 0.000000000000000000, -1.000000000000000000 ) ) ;
#6279=ORIENTED_EDGE ( 'NONE', *, *, #8487, .T. ) ;
#6282=ORIENTED_EDGE ( 'NONE', *, *, #11055, .T. ) ;
#6284=CARTESIAN_POINT ( 'NONE',  ( -7.241070169793059286, 29.81324547859994922, 5.250000000000000000 ) ) ;
#6285=CARTESIAN_POINT ( 'NONE',  ( -1.859188294733151059, 2.872909506853357442, 63.35000000001166143 ) ) ;
#6287=AXIS2_PLACEMENT_3D ( 'NONE', #6791, #2564, #10016 ) ;
#6288=CARTESIAN_POINT ( 'NONE',  ( -18.05918829504999934, 10.97290950744599947, 62.14999999999999858 ) ) ;
#6290=EDGE_CURVE ( 'NONE', #11290, #642, #966, .T. ) ;
#6294=CARTESIAN_POINT ( 'NONE',  ( -14.73910058758217723, 30.12180271180697133, 55.18720206871329736 ) ) ;
#6296=ORIENTED_EDGE ( 'NONE', *, *, #5596, .T. ) ;
#6298=LINE ( 'NONE', #10559, #7259 ) ;
#6301=ORIENTED_EDGE ( 'NONE', *, *, #6551, .T. ) ;
#6302=ORIENTED_EDGE ( 'NONE', *, *, #6399, .T. ) ;
#6303=FACE_OUTER_BOUND ( 'NONE', #13766, .T. ) ;
#6304=DIRECTION ( 'NONE',  ( 0.000000000000000000, -1.000000000000000000, 0.000000000000000000 ) ) ;
#6305=FACE_OUTER_BOUND ( 'NONE', #11841, .T. ) ;
#6306=EDGE_CURVE ( 'NONE', #6072, #912, #4690, .T. ) ;
#6311=VERTEX_POINT ( 'NONE', #1296 ) ;
#6312=EDGE_LOOP ( 'NONE', ( #4719, #9330, #652, #11418, #330, #2019, #4624, #2713, #4771, #13164, #6798, #8580, #104 ) ) ;
#6313=ORIENTED_EDGE ( 'NONE', *, *, #10960, .T. ) ;
#6317=DIRECTION ( 'NONE',  ( 0.000000000000000000, 0.000000000000000000, -1.000000000000000000 ) ) ;
#6318=VERTEX_POINT ( 'NONE', #8839 ) ;
#6319=DIRECTION ( 'NONE',  ( 2.267612386897784912E-16, -1.000000000000000000, 0.000000000000000000 ) ) ;
#6320=CARTESIAN_POINT ( 'NONE',  ( -35.05918829505000645, 27.97290950744599769, 68.85549045786049760 ) ) ;
#6323=EDGE_CURVE ( 'NONE', #10024, #3793, #7114, .T. ) ;
#6327=AXIS2_PLACEMENT_3D ( 'NONE', #10298, #7904, #783 ) ;
#6328=EDGE_CURVE ( 'NONE', #1042, #642, #3578, .T. ) ;
#6329=VERTEX_POINT ( 'NONE', #5627 ) ;
#6330=ORIENTED_EDGE ( 'NONE', *, *, #13427, .F. ) ;
#6331=CARTESIAN_POINT ( 'NONE',  ( -10.25088531517539714, 30.80589556422609832, 83.57661607529820458 ) ) ;
#6332=ORIENTED_EDGE ( 'NONE', *, *, #7232, .T. ) ;
#6334=CARTESIAN_POINT ( 'NONE',  ( -18.05918829504999934, 30.47290950744599769, 61.89660000000000650 ) ) ;
#6336=CARTESIAN_POINT ( 'NONE',  ( -20.13390280776154384, 30.26743272311685118, 53.69271067728588775 ) ) ;
#6337=SURFACE_STYLE_FILL_AREA ( #5339 ) ;
#6340=DIRECTION ( 'NONE',  ( 0.000000000000000000, 0.000000000000000000, -1.000000000000000000 ) ) ;
#6343=VERTEX_POINT ( 'NONE', #4793 ) ;
#6345=EDGE_CURVE ( 'NONE', #2105, #9316, #12489, .T. ) ;
#6347=CARTESIAN_POINT ( 'NONE',  ( -13.29473957835121389, 8.508638270346013499, 68.48645984990002944 ) ) ;
#6349=FILL_AREA_STYLE ('',( #193 ) ) ;
#6350=DIRECTION ( 'NONE',  ( 0.000000000000000000, 0.000000000000000000, -1.000000000000000000 ) ) ;
#6351=DIRECTION ( 'NONE',  ( 1.000000000000000000, 0.000000000000000000, 0.000000000000000000 ) ) ;
#6354=CARTESIAN_POINT ( 'NONE',  ( -15.32570436422911975, 30.19895062898915938, 54.30601320233879648 ) ) ;
#6357=VERTEX_POINT ( 'NONE', #1374 ) ;
#6359=ORIENTED_EDGE ( 'NONE', *, *, #11254, .T. ) ;
#6360=DIRECTION ( 'NONE',  ( 0.4528443260392608916, 0.8915896008669279560, 0.000000000000000000 ) ) ;
#6362=CARTESIAN_POINT ( 'NONE',  ( -18.05918829504999934, 10.97290950744599947, 53.85000000000000142 ) ) ;
#6363=ORIENTED_EDGE ( 'NONE', *, *, #7319, .F. ) ;
#6365=FACE_OUTER_BOUND ( 'NONE', #4830, .T. ) ;
#6367=FACE_BOUND ( 'NONE', #804, .T. ) ;
#6368=AXIS2_PLACEMENT_3D ( 'NONE', #8230, #6278, #9147 ) ;
#6369=ORIENTED_EDGE ( 'NONE', *, *, #10248, .F. ) ;
#6370=VERTEX_POINT ( 'NONE', #3683 ) ;
#6372=EDGE_CURVE ( 'NONE', #8976, #9897, #6458, .T. ) ;
#6373=ORIENTED_EDGE ( 'NONE', *, *, #12028, .T. ) ;
#6375=LINE ( 'NONE', #2801, #8431 ) ;
#6376=DIRECTION ( 'NONE',  ( -1.000000000000000000, 0.000000000000000000, 0.000000000000000000 ) ) ;
#6377=VECTOR ( 'NONE', #12552, 1000.000000000000000 ) ;
#6378=ADVANCED_FACE ( 'NONE', ( #3623 ), #1575, .T. ) ;
#6380=CARTESIAN_POINT ( 'NONE',  ( -19.02868427256591133, 26.94368128781859539, 56.20497232447349489 ) ) ;
#6382=DIRECTION ( 'NONE',  ( 0.4528443260392608916, 0.8915896008669279560, 0.000000000000000000 ) ) ;
#6384=DIRECTION ( 'NONE',  ( -1.000000000000000000, 0.000000000000000000, 0.000000000000000000 ) ) ;
#6386=EDGE_LOOP ( 'NONE', ( #7203, #9146, #8387, #6520 ) ) ;
#6387=EDGE_CURVE ( 'NONE', #6644, #13079, #5755, .T. ) ;
#6391=CARTESIAN_POINT ( 'NONE',  ( -1.559188295050000006, 10.97290950744599947, 57.35000000000000142 ) ) ;
#6392=CARTESIAN_POINT ( 'NONE',  ( -20.76349711708835954, 30.20233709048880755, 54.27308111598625118 ) ) ;
#6393=DIRECTION ( 'NONE',  ( 0.000000000000000000, 0.000000000000000000, -1.000000000000000000 ) ) ;
#6395=CARTESIAN_POINT ( 'NONE',  ( -1.059188295049996231, 27.97290950744599769, 17.25000000000000000 ) ) ;
#6396=CARTESIAN_POINT ( 'NONE',  ( -18.05918829488915023, 18.13901823688300396, 61.72253826514069885 ) ) ;
#6397=DIRECTION ( 'NONE',  ( 0.000000000000000000, 0.000000000000000000, -1.000000000000000000 ) ) ;
#6398=CIRCLE ( 'NONE', #1713, 6.449999999999997513 ) ;
#6399=EDGE_CURVE ( 'NONE', #8485, #87, #6905, .T. ) ;
#6403=DIRECTION ( 'NONE',  ( 0.000000000000000000, 0.000000000000000000, -1.000000000000000000 ) ) ;
#6404=ORIENTED_EDGE ( 'NONE', *, *, #8140, .F. ) ;
#6406=ORIENTED_EDGE ( 'NONE', *, *, #5444, .F. ) ;
#6408=CARTESIAN_POINT ( 'NONE',  ( -38.38077571930826082, 22.44393519180575680, 5.250000000000000000 ) ) ;
#6410=ORIENTED_EDGE ( 'NONE', *, *, #5444, .T. ) ;
#6412=EDGE_CURVE ( 'NONE', #6850, #12924, #9907, .T. ) ;
#6414=AXIS2_PLACEMENT_3D ( 'NONE', #12357, #542, #3838 ) ;
#6416=UNCERTAINTY_MEASURE_WITH_UNIT (LENGTH_MEASURE( 1.000000000000000082E-05 ), #4949, 'distance_accuracy_value', 'NONE');
#6417=ORIENTED_EDGE ( 'NONE', *, *, #5061, .T. ) ;
#6418=CARTESIAN_POINT ( 'NONE',  ( -15.23092771910337717, 30.18746625253793425, 54.42100116539269550 ) ) ;
#6419=AXIS2_PLACEMENT_3D ( 'NONE', #6288, #5227, #10342 ) ;
#6422=EDGE_LOOP ( 'NONE', ( #553, #9166, #10928, #4832 ) ) ;
#6424=DIRECTION ( 'NONE',  ( -1.000000000000000000, 0.000000000000000000, 0.000000000000000000 ) ) ;
#6425=AXIS2_PLACEMENT_3D ( 'NONE', #3192, #11694, #2005 ) ;
#6426=CARTESIAN_POINT ( 'NONE',  ( -35.05918829505000645, 27.97290950744599769, 64.85000000000000853 ) ) ;
#6427=SURFACE_SIDE_STYLE ('',( #7518 ) ) ;
#6429=ORIENTED_EDGE ( 'NONE', *, *, #7619, .F. ) ;
#6431=DIRECTION ( 'NONE',  ( 0.000000000000000000, 0.000000000000000000, -1.000000000000000000 ) ) ;
#6432=CARTESIAN_POINT ( 'NONE',  ( -1.899121662050003101, 19.05294282444601706, 63.34900083300006202 ) ) ;
#6433=PLANE ( 'NONE',  #11389 ) ;
#6434=AXIS2_PLACEMENT_3D ( 'NONE', #11654, #12825, #11856 ) ;
#6435=EDGE_CURVE ( 'NONE', #1261, #4307, #8918, .T. ) ;
#6436=AXIS2_PLACEMENT_3D ( 'NONE', #5549, #4657, #10040 ) ;
#6439=VERTEX_POINT ( 'NONE', #13307 ) ;
#6440=DIRECTION ( 'NONE',  ( 0.000000000000000000, 0.000000000000000000, 1.000000000000000000 ) ) ;
#6441=ORIENTED_EDGE ( 'NONE', *, *, #5217, .T. ) ;
#6443=VERTEX_POINT ( 'NONE', #10878 ) ;
#6446=LINE ( 'NONE', #10713, #853 ) ;
#6447=CARTESIAN_POINT ( 'NONE',  ( -10.25088531517539714, 30.80589556422609832, 17.25000000000000000 ) ) ;
#6448=AXIS2_PLACEMENT_3D ( 'NONE', #13590, #10455, #884 ) ;
#6453=CARTESIAN_POINT ( 'NONE',  ( -18.05918829504999934, 10.97290950744599947, 61.85000000000000142 ) ) ;
#6456=ADVANCED_FACE ( 'NONE', ( #3478 ), #7706, .F. ) ;
#6457=AXIS2_PLACEMENT_3D ( 'NONE', #3802, #8972, #2706 ) ;
#6458=CIRCLE ( 'NONE', #890, 17.00000000000000000 ) ;
#6467=ORIENTED_EDGE ( 'NONE', *, *, #8159, .F. ) ;
#6468=DIRECTION ( 'NONE',  ( -1.000000000000000000, 0.000000000000000000, 0.000000000000000000 ) ) ;
#6469=DIRECTION ( 'NONE',  ( 1.000000000000000000, -9.130123557772674004E-16, 0.000000000000000000 ) ) ;
#6470=CARTESIAN_POINT ( 'NONE',  ( -18.05918829309690210, 18.59099508048574734, 61.65955166400529919 ) ) ;
#6471=DIRECTION ( 'NONE',  ( 0.000000000000000000, 0.000000000000000000, -1.000000000000000000 ) ) ;
#6472=AXIS2_PLACEMENT_3D ( 'NONE', #5095, #2759, #13336 ) ;
#6473=AXIS2_PLACEMENT_3D ( 'NONE', #6587, #2567, #5735 ) ;
#6477=DIRECTION ( 'NONE',  ( 0.2878798879079290662, 0.9576665234506832602, 0.000000000000000000 ) ) ;
#6479=AXIS2_PLACEMENT_3D ( 'NONE', #5720, #5442, #5653 ) ;
#6482=ORIENTED_EDGE ( 'NONE', *, *, #5536, .T. ) ;
#6483=CARTESIAN_POINT ( 'NONE',  ( -10.78334210919089919, 29.19143287883919768, 64.85000000000000853 ) ) ;
#6485=CYLINDRICAL_SURFACE ( 'NONE', #8067, 16.72262947720610171 ) ;
#6486=CARTESIAN_POINT ( 'NONE',  ( -19.91165729514404603, 13.07251866242952154, 23.90000000000000213 ) ) ;
#6487=CARTESIAN_POINT ( 'NONE',  ( -18.05918829504999934, 10.97290950744599947, 63.64999999999999858 ) ) ;
#6488=DIRECTION ( 'NONE',  ( 0.000000000000000000, 0.000000000000000000, 1.000000000000000000 ) ) ;
#6489=LINE ( 'NONE', #8794, #11551 ) ;
#6492=AXIS2_PLACEMENT_3D ( 'NONE', #12899, #3426, #1308 ) ;
#6494=VERTEX_POINT ( 'NONE', #10373 ) ;
#6496=CARTESIAN_POINT ( 'NONE',  ( -17.20179490422193780, 30.34444651895395850, 53.10284867194972946 ) ) ;
#6500=CARTESIAN_POINT ( 'NONE',  ( -10.79835982676942052, -4.028726038184999858, 63.45000000000000284 ) ) ;
#6501=STYLED_ITEM ( 'NONE', ( #210 ), #4352 ) ;
#6505=VECTOR ( 'NONE', #6033, 1000.000000000000000 ) ;
#6506=VERTEX_POINT ( 'NONE', #2720 ) ;
#6509=LINE ( 'NONE', #10566, #450 ) ;
#6511=VECTOR ( 'NONE', #12777, 1000.000000000000114 ) ;
#6512=EDGE_LOOP ( 'NONE', ( #1839, #3482, #6757, #12637 ) ) ;
#6513=LINE ( 'NONE', #9083, #560 ) ;
#6516=ORIENTED_EDGE ( 'NONE', *, *, #8878, .T. ) ;
#6517=CARTESIAN_POINT ( 'NONE',  ( -25.05563313235659706, -2.802149825948039741, 58.54999999999999716 ) ) ;
#6519=DIRECTION ( 'NONE',  ( -1.000000000000000000, 0.000000000000000000, 0.000000000000000000 ) ) ;
#6520=ORIENTED_EDGE ( 'NONE', *, *, #714, .F. ) ;
#6521=CARTESIAN_POINT ( 'NONE',  ( -38.63164489498320364, 10.97290950744599947, 73.76763816269230745 ) ) ;
#6522=CIRCLE ( 'NONE', #13434, 1.725000000000000755 ) ;
#6523=CARTESIAN_POINT ( 'NONE',  ( -17.28440556981917808, 26.95410257713844615, 56.06541086284084230 ) ) ;
#6528=AXIS2_PLACEMENT_3D ( 'NONE', #3391, #4715, #8757 ) ;
#6530=ORIENTED_EDGE ( 'NONE', *, *, #11721, .F. ) ;
#6533=ORIENTED_EDGE ( 'NONE', *, *, #1664, .F. ) ;
#6534=DIRECTION ( 'NONE',  ( 0.000000000000000000, 0.000000000000000000, -1.000000000000000000 ) ) ;
#6535=CARTESIAN_POINT ( 'NONE',  ( -41.50918829505000218, -6.027090492554000534, 83.57661607529820458 ) ) ;
#6536=EDGE_CURVE ( 'NONE', #3266, #10507, #10932, .T. ) ;
#6538=CARTESIAN_POINT ( 'NONE',  ( -20.27573349293325933, 30.25428168448397415, 53.80284863901545833 ) ) ;
#6540=CARTESIAN_POINT ( 'NONE',  ( -1.059188295049996231, -6.027090492554000534, 64.35000000000000853 ) ) ;
#6542=VECTOR ( 'NONE', #6083, 1000.000000000000114 ) ;
#6544=ADVANCED_FACE ( 'NONE', ( #3819 ), #11488, .T. ) ;
#6546=AXIS2_PLACEMENT_3D ( 'NONE', #12078, #8860, #7872 ) ;
#6548=VERTEX_POINT ( 'NONE', #596 ) ;
#6549=EDGE_LOOP ( 'NONE', ( #8649, #1737, #9353, #3851 ) ) ;
#6550=DIRECTION ( 'NONE',  ( -1.000000000000000000, 0.000000000000000000, 0.000000000000000000 ) ) ;
#6551=EDGE_CURVE ( 'NONE', #707, #9911, #2256, .T. ) ;
#6552=FACE_OUTER_BOUND ( 'NONE', #7756, .T. ) ;
#6553=DIRECTION ( 'NONE',  ( 0.000000000000000000, 0.000000000000000000, 1.000000000000000000 ) ) ;
#6558=ADVANCED_FACE ( 'NONE', ( #2790 ), #227, .T. ) ;
#6559=ORIENTED_EDGE ( 'NONE', *, *, #8350, .T. ) ;
#6561=CARTESIAN_POINT ( 'NONE',  ( -17.24607760227289077, 30.34604302011652521, 53.09143874144074005 ) ) ;
#6563=LINE ( 'NONE', #10831, #2171 ) ;
#6565=DIRECTION ( 'NONE',  ( 0.000000000000000000, 0.000000000000000000, 1.000000000000000000 ) ) ;
#6567=DIRECTION ( 'NONE',  ( 0.3132098788326395100, 0.9496839325805419563, 0.000000000000000000 ) ) ;
#6569=EDGE_CURVE ( 'NONE', #10012, #13212, #11426, .T. ) ;
#6574=CIRCLE ( 'NONE', #10601, 8.300000000000000711 ) ;
#6575=CARTESIAN_POINT ( 'NONE',  ( -35.05918829505000645, 27.97290950744599769, 68.85549045786049760 ) ) ;
#6577=VERTEX_POINT ( 'NONE', #13447 ) ;
#6578=ORIENTED_EDGE ( 'NONE', *, *, #6536, .F. ) ;
#6580=DIRECTION ( 'NONE',  ( 0.000000000000000000, 0.000000000000000000, -1.000000000000000000 ) ) ;
#6582=DIRECTION ( 'NONE',  ( 0.000000000000000000, 0.000000000000000000, -1.000000000000000000 ) ) ;
#6584=CARTESIAN_POINT ( 'NONE',  ( -34.68447646404997897, 19.28555359244599288, 63.26601075299999621 ) ) ;
#6585=CARTESIAN_POINT ( 'NONE',  ( -18.05918829504999934, 10.97290950744599947, 64.85000000000000853 ) ) ;
#6587=CARTESIAN_POINT ( 'NONE',  ( -18.05918829504999934, 10.97290950744599947, 61.65000000000000568 ) ) ;
#6589=VERTEX_POINT ( 'NONE', #3060 ) ;
#6590=CIRCLE ( 'NONE', #12833, 6.000000000000000888 ) ;
#6591=DIRECTION ( 'NONE',  ( 0.000000000000000000, 0.000000000000000000, -1.000000000000000000 ) ) ;
#6596=CARTESIAN_POINT ( 'NONE',  ( -19.29163931862649406, 30.32761401381639033, 53.22486482497648552 ) ) ;
#6598=CARTESIAN_POINT ( 'NONE',  ( -18.05918829505001355, 18.23680593644599668, 62.03182374100007479 ) ) ;
#6599=DIRECTION ( 'NONE',  ( 1.000000000000000000, 0.000000000000000000, 0.000000000000000000 ) ) ;
#6600=LINE ( 'NONE', #11715, #7591 ) ;
#6601=DIRECTION ( 'NONE',  ( -1.000000000000000000, 0.000000000000000000, 0.000000000000000000 ) ) ;
#6603=EDGE_CURVE ( 'NONE', #6784, #1834, #9841, .T. ) ;
#6607=EDGE_LOOP ( 'NONE', ( #6429, #5345 ) ) ;
#6612=FACE_OUTER_BOUND ( 'NONE', #5049, .T. ) ;
#6613=AXIS2_PLACEMENT_3D ( 'NONE', #9766, #3282, #11934 ) ;
#6617=CARTESIAN_POINT ( 'NONE',  ( -24.35918829505000005, 10.97290950744599947, 61.86500000000000199 ) ) ;
#6619=CARTESIAN_POINT ( 'NONE',  ( -35.05918829505000645, 27.97290950744599769, 64.85000000000000853 ) ) ;
#6620=CARTESIAN_POINT ( 'NONE',  ( -23.05918829504999934, 10.97290950744599947, 118.8499999999999943 ) ) ;
#6623=ADVANCED_FACE ( 'NONE', ( #11632 ), #7335, .T. ) ;
#6625=CARTESIAN_POINT ( 'NONE',  ( -15.52422514065462877, 30.22157476238875162, 54.09163654685160338 ) ) ;
#6628=DIRECTION ( 'NONE',  ( -1.000000000000000000, 0.000000000000000000, 0.000000000000000000 ) ) ;
#6629=CIRCLE ( 'NONE', #613, 23.22993838181875148 ) ;
#6630=ORIENTED_EDGE ( 'NONE', *, *, #3969, .T. ) ;
#6634=EDGE_CURVE ( 'NONE', #952, #2401, #11597, .T. ) ;
#6635=CIRCLE ( 'NONE', #10232, 5.500000000000000888 ) ;
#6636=ORIENTED_EDGE ( 'NONE', *, *, #5865, .F. ) ;
#6637=AXIS2_PLACEMENT_3D ( 'NONE', #13767, #13385, #1655 ) ;
#6638=EDGE_LOOP ( 'NONE', ( #1144, #316, #10083, #13022 ) ) ;
#6641=DIRECTION ( 'NONE',  ( -0.9496839325805422893, 0.3132098788326386218, 0.000000000000000000 ) ) ;
#6642=ORIENTED_EDGE ( 'NONE', *, *, #12957, .T. ) ;
#6643=EDGE_LOOP ( 'NONE', ( #3673, #4295, #6970, #7592, #12836, #9302 ) ) ;
#6644=VERTEX_POINT ( 'NONE', #1140 ) ;
#6645=EDGE_CURVE ( 'NONE', #10203, #12272, #13714, .T. ) ;
#6646=ORIENTED_EDGE ( 'NONE', *, *, #2071, .F. ) ;
#6647=CARTESIAN_POINT ( 'NONE',  ( -18.05918829504999934, 30.36027202460864771, 52.99086025162979752 ) ) ;
#6648=DIRECTION ( 'NONE',  ( 0.000000000000000000, 0.000000000000000000, -1.000000000000000000 ) ) ;
#6651=DIRECTION ( 'NONE',  ( 1.000000000000000000, 0.000000000000000000, 0.000000000000000000 ) ) ;
#6653=PLANE ( 'NONE',  #7746 ) ;
#6654=FACE_OUTER_BOUND ( 'NONE', #8138, .T. ) ;
#6655=AXIS2_PLACEMENT_3D ( 'NONE', #7393, #6221, #6304 ) ;
#6656=CARTESIAN_POINT ( 'NONE',  ( 3.190811704950004657, -6.027090492554000534, 58.85000000000000142 ) ) ;
#6658=EDGE_LOOP ( 'NONE', ( #7475, #11723, #13662, #838 ) ) ;
#6663=EDGE_LOOP ( 'NONE', ( #9935, #6559, #7991, #8249, #6313, #415, #12155, #2360 ) ) ;
#6665=EDGE_CURVE ( 'NONE', #3112, #10847, #7469, .T. ) ;
#6668=DIRECTION ( 'NONE',  ( 0.000000000000000000, 0.000000000000000000, 1.000000000000000000 ) ) ;
#6670=CARTESIAN_POINT ( 'NONE',  ( -20.65862537727294068, 30.21441468393235041, 60.54187128424251085 ) ) ;
#6671=SURFACE_SIDE_STYLE ('',( #3542 ) ) ;
#6672=CARTESIAN_POINT ( 'NONE',  ( -23.85417428574490373, 12.52794563810342154, 68.84999999999999432 ) ) ;
#6675=DIRECTION ( 'NONE',  ( -1.000000000000000000, 0.000000000000000000, 0.000000000000000000 ) ) ;
#6676=AXIS2_PLACEMENT_3D ( 'NONE', #6453, #11971, #6382 ) ;
#6677=AXIS2_PLACEMENT_3D ( 'NONE', #4659, #6809, #6675 ) ;
#6678=VERTEX_POINT ( 'NONE', #4369 ) ;
#6679=EDGE_LOOP ( 'NONE', ( #9415, #7349, #10705, #7750 ) ) ;
#6682=DIRECTION ( 'NONE',  ( 0.000000000000000000, 0.000000000000000000, 1.000000000000000000 ) ) ;
#6686=CARTESIAN_POINT ( 'NONE',  ( -37.75918829505000218, -6.027090492554000534, 64.85000000000000853 ) ) ;
#6687=DIRECTION ( 'NONE',  ( 0.000000000000000000, 0.000000000000000000, -1.000000000000000000 ) ) ;
#6688=CARTESIAN_POINT ( 'NONE',  ( -26.35918829505000005, 10.97290950744599947, 61.86500000000000199 ) ) ;
#6691=ADVANCED_FACE ( 'NONE', ( #7274 ), #11557, .T. ) ;
#6692=CARTESIAN_POINT ( 'NONE',  ( -18.05918829504999934, 10.97290950744599947, 60.04999999999999716 ) ) ;
#6695=DIRECTION ( 'NONE',  ( 0.000000000000000000, 0.000000000000000000, -1.000000000000000000 ) ) ;
#6699=EDGE_CURVE ( 'NONE', #10425, #2443, #13378, .T. ) ;
#6700=CIRCLE ( 'NONE', #5777, 6.450000000000001066 ) ;
#6701=AXIS2_PLACEMENT_3D ( 'NONE', #11336, #3041, #4977 ) ;
#6702=ORIENTED_EDGE ( 'NONE', *, *, #3801, .T. ) ;
#6703=ORIENTED_EDGE ( 'NONE', *, *, #9094, .T. ) ;
#6704=DIRECTION ( 'NONE',  ( 0.000000000000000000, 0.000000000000000000, -1.000000000000000000 ) ) ;
#6707=FACE_OUTER_BOUND ( 'NONE', #6663, .T. ) ;
#6709=DIRECTION ( 'NONE',  ( 0.000000000000000000, 0.000000000000000000, -1.000000000000000000 ) ) ;
#6712=CIRCLE ( 'NONE', #6260, 1.000000000000000000 ) ;
#6713=VECTOR ( 'NONE', #9560, 1000.000000000000000 ) ;
#6716=EDGE_CURVE ( 'NONE', #13212, #5077, #8035, .T. ) ;
#6721=CARTESIAN_POINT ( 'NONE',  ( -15.85016405347683488, 30.25500104532764212, 60.90324978431328162 ) ) ;
#6722=VECTOR ( 'NONE', #5392, 1000.000000000000000 ) ;
#6723=AXIS2_PLACEMENT_3D ( 'NONE', #1205, #9737, #10646 ) ;
#6724=ORIENTED_EDGE ( 'NONE', *, *, #6569, .F. ) ;
#6727=ORIENTED_EDGE ( 'NONE', *, *, #13461, .F. ) ;
#6728=CARTESIAN_POINT ( 'NONE',  ( 3.690811704950004657, -6.027090492554000534, 68.85549045786049760 ) ) ;
#6729=PLANE ( 'NONE',  #8647 ) ;
#6732=CARTESIAN_POINT ( 'NONE',  ( -11.46335496205000126, 10.97290950744599947, 60.40999999999999659 ) ) ;
#6733=CARTESIAN_POINT ( 'NONE',  ( -16.64497473267689998, 26.91028695795525039, 56.84999999999999432 ) ) ;
#6734=CARTESIAN_POINT ( 'NONE',  ( -18.05918829504999934, 10.97290950744599947, 68.84999999999999432 ) ) ;
#6736=ADVANCED_FACE ( 'NONE', ( #12116 ), #3394, .T. ) ;
#6738=ORIENTED_EDGE ( 'NONE', *, *, #5831, .F. ) ;
#6739=ORIENTED_EDGE ( 'NONE', *, *, #9102, .F. ) ;
#6740=CONICAL_SURFACE ( 'NONE', #5615, 7.618085573000000110, 0.1329427246665018103 ) ;
#6741=CARTESIAN_POINT ( 'NONE',  ( 1.097360187335109982, -3.327306731351814761, 7.250000000000000000 ) ) ;
#6742=ORIENTED_EDGE ( 'NONE', *, *, #10839, .F. ) ;
#6744=EDGE_CURVE ( 'NONE', #3046, #3872, #12284, .T. ) ;
#6745=CARTESIAN_POINT ( 'NONE',  ( -21.37114540074985314, 30.12306837294896056, 55.16656713510205634 ) ) ;
#6750=DIRECTION ( 'NONE',  ( 0.000000000000000000, 0.000000000000000000, 1.000000000000000000 ) ) ;
#6751=DIRECTION ( 'NONE',  ( 1.224646799147353207E-16, 1.000000000000000000, -0.000000000000000000 ) ) ;
#6752=EDGE_CURVE ( 'NONE', #4217, #6, #12181, .T. ) ;
#6756=DIRECTION ( 'NONE',  ( 0.000000000000000000, 0.000000000000000000, -1.000000000000000000 ) ) ;
#6757=ORIENTED_EDGE ( 'NONE', *, *, #4180, .T. ) ;
#6762=PLANE ( 'NONE',  #3165 ) ;
#6763=CARTESIAN_POINT ( 'NONE',  ( -35.05918829505000645, 27.97290950744599769, 58.85000000000000142 ) ) ;
#6765=DIRECTION ( 'NONE',  ( 0.000000000000000000, 0.000000000000000000, -1.000000000000000000 ) ) ;
#6766=PLANE ( 'NONE',  #9851 ) ;
#6767=DIRECTION ( 'NONE',  ( 0.000000000000000000, 0.000000000000000000, -1.000000000000000000 ) ) ;
#6769=AXIS2_PLACEMENT_3D ( 'NONE', #8935, #13192, #3642 ) ;
#6771=FACE_OUTER_BOUND ( 'NONE', #512, .T. ) ;
#6772=ORIENTED_EDGE ( 'NONE', *, *, #9101, .F. ) ;
#6775=DIRECTION ( 'NONE',  ( 0.000000000000000000, 0.000000000000000000, -1.000000000000000000 ) ) ;
#6777=FACE_OUTER_BOUND ( 'NONE', #13645, .T. ) ;
#6778=PLANE ( 'NONE',  #2704 ) ;
#6780=VECTOR ( 'NONE', #250, 1000.000000000000000 ) ;
#6782=CARTESIAN_POINT ( 'NONE',  ( -14.32322260522609980, 18.32852371459815188, 60.04999999999999716 ) ) ;
#6784=VERTEX_POINT ( 'NONE', #9950 ) ;
#6785=ORIENTED_EDGE ( 'NONE', *, *, #11763, .T. ) ;
#6786=ORIENTED_EDGE ( 'NONE', *, *, #9499, .T. ) ;
#6788=PLANE ( 'NONE',  #1298 ) ;
#6789=DIRECTION ( 'NONE',  ( 0.000000000000000000, 0.000000000000000000, 1.000000000000000000 ) ) ;
#6790=ORIENTED_EDGE ( 'NONE', *, *, #3636, .F. ) ;
#6791=CARTESIAN_POINT ( 'NONE',  ( -18.05918829504999934, 10.97290950744599947, 116.8499999999999943 ) ) ;
#6793=FACE_OUTER_BOUND ( 'NONE', #13235, .T. ) ;
#6794=CARTESIAN_POINT ( 'NONE',  ( -16.07440008066354764, 8.723328269963658954, 27.09999999999999787 ) ) ;
#6795=CIRCLE ( 'NONE', #11049, 3.000000000000000888 ) ;
#6796=ORIENTED_EDGE ( 'NONE', *, *, #7448, .T. ) ;
#6798=ORIENTED_EDGE ( 'NONE', *, *, #4180, .F. ) ;
#6800=DIRECTION ( 'NONE',  ( -1.000000000000000000, 0.000000000000000000, 0.000000000000000000 ) ) ;
#6801=ORIENTED_EDGE ( 'NONE', *, *, #6699, .T. ) ;
#6803=AXIS2_PLACEMENT_3D ( 'NONE', #3500, #11043, #2470 ) ;
#6804=CARTESIAN_POINT ( 'NONE',  ( -21.64539278097895902, 30.08178984978753689, 58.87173069243009138 ) ) ;
#6805=DIRECTION ( 'NONE',  ( 0.000000000000000000, 0.000000000000000000, 1.000000000000000000 ) ) ;
#6807=DIRECTION ( 'NONE',  ( 0.000000000000000000, 0.000000000000000000, -1.000000000000000000 ) ) ;
#6808=DIRECTION ( 'NONE',  ( 0.000000000000000000, 0.000000000000000000, 1.000000000000000000 ) ) ;
#6809=DIRECTION ( 'NONE',  ( 0.000000000000000000, 0.000000000000000000, -1.000000000000000000 ) ) ;
#6812=EDGE_CURVE ( 'NONE', #5535, #6329, #12046, .T. ) ;
#6814=EDGE_LOOP ( 'NONE', ( #10011, #7646, #7856, #5419 ) ) ;
#6816=DIRECTION ( 'NONE',  ( 0.000000000000000000, 0.000000000000000000, 1.000000000000000000 ) ) ;
#6818=DIRECTION ( 'NONE',  ( -0.3202092937642119774, -0.6304490528084099044, 0.7071067811865499042 ) ) ;
#6819=DIRECTION ( 'NONE',  ( 0.000000000000000000, 0.000000000000000000, 1.000000000000000000 ) ) ;
#6820=EDGE_CURVE ( 'NONE', #10750, #4939, #4434, .T. ) ;
#6822=DIRECTION ( 'NONE',  ( 0.000000000000000000, 0.000000000000000000, 1.000000000000000000 ) ) ;
#6826=DIRECTION ( 'NONE',  ( -0.9496839325805410681, 0.3132098788326420635, 0.000000000000000000 ) ) ;
#6828=CARTESIAN_POINT ( 'NONE',  ( -18.05918829504999934, 10.97290950744599947, 60.04999999999999716 ) ) ;
#6829=VERTEX_POINT ( 'NONE', #5608 ) ;
#6830=AXIS2_PLACEMENT_3D ( 'NONE', #2607, #9927, #3852 ) ;
#6831=ORIENTED_EDGE ( 'NONE', *, *, #8957, .F. ) ;
#6833=DIRECTION ( 'NONE',  ( 0.000000000000000000, 0.000000000000000000, 1.000000000000000000 ) ) ;
#6836=ADVANCED_FACE ( 'NONE', ( #8973 ), #7131, .F. ) ;
#6839=DIRECTION ( 'NONE',  ( 1.000000000000000000, 0.000000000000000000, 0.000000000000000000 ) ) ;
#6841=AXIS2_PLACEMENT_3D ( 'NONE', #9206, #3070, #11573 ) ;
#6842=DIRECTION ( 'NONE',  ( 0.000000000000000000, 1.000000000000000000, 0.000000000000000000 ) ) ;
#6843=EDGE_LOOP ( 'NONE', ( #13346, #13405, #4767, #1105 ) ) ;
#6844=ORIENTED_EDGE ( 'NONE', *, *, #11587, .F. ) ;
#6846=CARTESIAN_POINT ( 'NONE',  ( -16.51503883096479441, 30.30889438433393224, 61.33492039510051086 ) ) ;
#6849=EDGE_LOOP ( 'NONE', ( #6967, #441 ) ) ;
#6850=VERTEX_POINT ( 'NONE', #6656 ) ;
#6851=ORIENTED_EDGE ( 'NONE', *, *, #6435, .T. ) ;
#6852=DIRECTION ( 'NONE',  ( 0.000000000000000000, 0.000000000000000000, -1.000000000000000000 ) ) ;
#6855=DIRECTION ( 'NONE',  ( -1.000000000000000000, 0.000000000000000000, 0.000000000000000000 ) ) ;
#6856=CARTESIAN_POINT ( 'NONE',  ( -1.059188295049996231, -6.027090492554000534, 58.85000000000000142 ) ) ;
#6857=EDGE_CURVE ( 'NONE', #10151, #12033, #11137, .T. ) ;
#6858=DIRECTION ( 'NONE',  ( -0.4528443260392609471, -0.8915896008669278450, 0.000000000000000000 ) ) ;
#6863=VECTOR ( 'NONE', #2505, 1000.000000000000114 ) ;
#6865=ORIENTED_EDGE ( 'NONE', *, *, #6744, .T. ) ;
#6867=VECTOR ( 'NONE', #5529, 1000.000000000000000 ) ;
#6868=AXIS2_PLACEMENT_3D ( 'NONE', #3933, #13627, #13694 ) ;
#6873=CARTESIAN_POINT ( 'NONE',  ( -21.32667269782450603, 30.12932847811543269, 59.61340462581008381 ) ) ;
#6877=EDGE_CURVE ( 'NONE', #2075, #9462, #5348, .T. ) ;
#6878=DIRECTION ( 'NONE',  ( -1.000000000000000000, 0.000000000000000000, 0.000000000000000000 ) ) ;
#6882=AXIS2_PLACEMENT_3D ( 'NONE', #7447, #13628, #5240 ) ;
#6884=VERTEX_POINT ( 'NONE', #11410 ) ;
#6885=DIRECTION ( 'NONE',  ( 0.000000000000000000, 0.000000000000000000, 1.000000000000000000 ) ) ;
#6888=LINE ( 'NONE', #13311, #7572 ) ;
#6891=PLANE ( 'NONE',  #7575 ) ;
#6892=CARTESIAN_POINT ( 'NONE',  ( -18.05918829504999934, 10.97290950744599947, 23.90000000000000213 ) ) ;
#6894=DIRECTION ( 'NONE',  ( 0.4528443260392610026, 0.8915896008669278450, 0.000000000000000000 ) ) ;
#6895=CARTESIAN_POINT ( 'NONE',  ( -35.05918829505000645, -6.027090492554000534, 7.250000000000000000 ) ) ;
#6897=CARTESIAN_POINT ( 'NONE',  ( -18.05918829504999934, 10.97290950744599947, 60.40999999999999659 ) ) ;
#6898=AXIS2_PLACEMENT_3D ( 'NONE', #11272, #1844, #4916 ) ;
#6902=ORIENTED_EDGE ( 'NONE', *, *, #7436, .F. ) ;
#6904=FACE_OUTER_BOUND ( 'NONE', #8782, .T. ) ;
#6905=CIRCLE ( 'NONE', #8689, 33.00000000000000000 ) ;
#6906=DIRECTION ( 'NONE',  ( 0.000000000000000000, 0.000000000000000000, -1.000000000000000000 ) ) ;
#6908=CARTESIAN_POINT ( 'NONE',  ( -37.75918829505000218, 27.97290950744599769, 7.250000000000000000 ) ) ;
#6910=CARTESIAN_POINT ( 'NONE',  ( -18.05918829504999934, 2.892876190446000084, 63.34900083300000517 ) ) ;
#6911=DIRECTION ( 'NONE',  ( 0.4528443260392608360, 0.8915896008669278450, 0.000000000000000000 ) ) ;
#6912=DIRECTION ( 'NONE',  ( -1.000000000000000000, 0.000000000000000000, 0.000000000000000000 ) ) ;
#6913=AXIS2_PLACEMENT_3D ( 'NONE', #13517, #3960, #4799 ) ;
#6916=EDGE_CURVE ( 'NONE', #11045, #952, #6700, .T. ) ;
#6918=CARTESIAN_POINT ( 'NONE',  ( -17.27672718608728886, 30.34709526170184546, 61.61607410999997114 ) ) ;
#6919=VERTEX_POINT ( 'NONE', #11476 ) ;
#6922=VECTOR ( 'NONE', #8620, 1000.000000000000000 ) ;
#6924=ORIENTED_EDGE ( 'NONE', *, *, #12631, .F. ) ;
#6925=AXIS2_PLACEMENT_3D ( 'NONE', #5115, #8333, #5379 ) ;
#6926=CARTESIAN_POINT ( 'NONE',  ( -34.72201093190195564, 10.97290950744599947, 17.25000000000000000 ) ) ;
#6927=AXIS2_PLACEMENT_3D ( 'NONE', #9380, #4083, #8329 ) ;
#6929=CARTESIAN_POINT ( 'NONE',  ( -25.86749127492454647, -8.860076549334127805, 83.57661607529820458 ) ) ;
#6931=CARTESIAN_POINT ( 'NONE',  ( -18.05918829504999934, 10.97290950744599947, 61.86500000000000199 ) ) ;
#6934=VECTOR ( 'NONE', #11498, 1000.000000000000000 ) ;
#6935=AXIS2_PLACEMENT_3D ( 'NONE', #5253, #4365, #10643 ) ;
#6939=EDGE_CURVE ( 'NONE', #1440, #8302, #9163, .T. ) ;
#6941=EDGE_LOOP ( 'NONE', ( #5424, #7190 ) ) ;
#6943=CARTESIAN_POINT ( 'NONE',  ( -20.86626825454071010, 30.19004818229314324, 60.30515349700372951 ) ) ;
#6947=FACE_OUTER_BOUND ( 'NONE', #6607, .T. ) ;
#6948=CARTESIAN_POINT ( 'NONE',  ( -5.631644894983189431, 10.97290950744599947, 17.25000000000000000 ) ) ;
#6949=CARTESIAN_POINT ( 'NONE',  ( -35.05918829505000645, 27.97290950744599769, 7.250000000000000000 ) ) ;
#6951=VECTOR ( 'NONE', #4803, 1000.000000000000000 ) ;
#6957=SURFACE_STYLE_USAGE ( .BOTH. , #3756 ) ;
#6961=DIRECTION ( 'NONE',  ( -1.000000000000000000, 0.000000000000000000, 0.000000000000000000 ) ) ;
#6963=LINE ( 'NONE', #11303, #11839 ) ;
#6965=DIRECTION ( 'NONE',  ( 0.000000000000000000, 0.000000000000000000, -1.000000000000000000 ) ) ;
#6967=ORIENTED_EDGE ( 'NONE', *, *, #1598, .T. ) ;
#6968=ADVANCED_FACE ( 'NONE', ( #12529 ), #8127, .F. ) ;
#6969=CYLINDRICAL_SURFACE ( 'NONE', #12168, 33.00000000000000000 ) ;
#6970=ORIENTED_EDGE ( 'NONE', *, *, #10164, .T. ) ;
#6972=ORIENTED_EDGE ( 'NONE', *, *, #4225, .F. ) ;
#6975=DIRECTION ( 'NONE',  ( -1.000000000000000000, 0.000000000000000000, 0.000000000000000000 ) ) ;
#6978=CARTESIAN_POINT ( 'NONE',  ( -30.48673169511680214, 10.97290950744599947, 64.85000000000000853 ) ) ;
#6979=DIRECTION ( 'NONE',  ( 0.000000000000000000, 0.000000000000000000, -1.000000000000000000 ) ) ;
#6981=ORIENTED_EDGE ( 'NONE', *, *, #2180, .F. ) ;
#6985=CARTESIAN_POINT ( 'NONE',  ( -1.059188295049996231, 27.97290950744599769, 64.85000000000000853 ) ) ;
#6987=ORIENTED_EDGE ( 'NONE', *, *, #10254, .T. ) ;
#6988=( NAMED_UNIT ( * ) PLANE_ANGLE_UNIT ( ) SI_UNIT ( $, .RADIAN. ) );
#6990=CYLINDRICAL_SURFACE ( 'NONE', #9848, 5.000000000000000888 ) ;
#6991=ORIENTED_EDGE ( 'NONE', *, *, #6569, .T. ) ;
#6992=CIRCLE ( 'NONE', #981, 4.750000000000000888 ) ;
#6995=EDGE_CURVE ( 'NONE', #12924, #8537, #9606, .T. ) ;
#6996=CARTESIAN_POINT ( 'NONE',  ( -17.23821357112329977, 5.029341513162310484, 64.85000000000000853 ) ) ;
#6997=CARTESIAN_POINT ( 'NONE',  ( -18.05918829504999934, 30.36027202460864771, 61.70913974837019822 ) ) ;
#6998=EDGE_CURVE ( 'NONE', #11514, #2014, #3940, .T. ) ;
#6999=CARTESIAN_POINT ( 'NONE',  ( -17.14002684535937604, 27.94862847170599096, 58.55192794567741288 ) ) ;
#7002=ORIENTED_EDGE ( 'NONE', *, *, #497, .T. ) ;
#7003=ORIENTED_EDGE ( 'NONE', *, *, #2930, .F. ) ;
#7004=ORIENTED_EDGE ( 'NONE', *, *, #3910, .F. ) ;
#7006=CARTESIAN_POINT ( 'NONE',  ( -18.05918829504999934, 10.97290950744599947, 7.250000000000000000 ) ) ;
#7007=DIRECTION ( 'NONE',  ( 0.000000000000000000, 1.000000000000000000, 0.000000000000000000 ) ) ;
#7010=DIRECTION ( 'NONE',  ( 1.000000000000000000, 0.000000000000000000, 0.000000000000000000 ) ) ;
#7011=ORIENTED_EDGE ( 'NONE', *, *, #4569, .F. ) ;
#7012=EDGE_CURVE ( 'NONE', #2384, #12649, #3152, .T. ) ;
#7014=CLOSED_SHELL ( 'NONE', ( #1795, #1093, #4105, #9200, #2378, #9800 ) ) ;
#7015=AXIS2_PLACEMENT_3D ( 'NONE', #10145, #6440, #1338 ) ;
#7022=FACE_OUTER_BOUND ( 'NONE', #3047, .T. ) ;
#7024=DIRECTION ( 'NONE',  ( 0.000000000000000000, 0.000000000000000000, -1.000000000000000000 ) ) ;
#7026=DIRECTION ( 'NONE',  ( 1.000000000000000000, 0.000000000000000000, 0.000000000000000000 ) ) ;
#7029=EDGE_CURVE ( 'NONE', #11722, #6318, #907, .T. ) ;
#7030=CIRCLE ( 'NONE', #6368, 16.95000000000000284 ) ;
#7034=ORIENTED_EDGE ( 'NONE', *, *, #9594, .F. ) ;
#7035=FACE_OUTER_BOUND ( 'NONE', #6214, .T. ) ;
#7036=ORIENTED_EDGE ( 'NONE', *, *, #3860, .F. ) ;
#7038=AXIS2_PLACEMENT_3D ( 'NONE', #4311, #7554, #5333 ) ;
#7040=DIRECTION ( 'NONE',  ( -0.6615960714621564875, 0.7498604124941129490, 0.000000000000000000 ) ) ;
#7043=DIRECTION ( 'NONE',  ( 1.000000000000000000, 0.000000000000000000, 0.000000000000000000 ) ) ;
#7044=ADVANCED_FACE ( 'NONE', ( #5813, #10231 ), #6433, .F. ) ;
#7046=AXIS2_PLACEMENT_3D ( 'NONE', #13622, #8250, #12722 ) ;
#7047=ADVANCED_FACE ( 'NONE', ( #8397 ), #4086, .T. ) ;
#7048=ORIENTED_EDGE ( 'NONE', *, *, #11486, .F. ) ;
#7049=ORIENTED_EDGE ( 'NONE', *, *, #5729, .F. ) ;
#7050=CARTESIAN_POINT ( 'NONE',  ( -14.22822014949529112, 30.04220389463379703, 57.85890972080246542 ) ) ;
#7051=VERTEX_POINT ( 'NONE', #9387 ) ;
#7052=DIRECTION ( 'NONE',  ( 0.000000000000000000, 0.000000000000000000, -1.000000000000000000 ) ) ;
#7053=DIRECTION ( 'NONE',  ( 0.000000000000000000, 0.000000000000000000, -1.000000000000000000 ) ) ;
#7054=ORIENTED_EDGE ( 'NONE', *, *, #3973, .F. ) ;
#7055=ORIENTED_EDGE ( 'NONE', *, *, #11747, .F. ) ;
#7056=FACE_OUTER_BOUND ( 'NONE', #6679, .T. ) ;
#7057=CARTESIAN_POINT ( 'NONE',  ( -18.05918829504999934, 10.97290950744599947, 63.54999999999999716 ) ) ;
#7059=AXIS2_PLACEMENT_3D ( 'NONE', #12785, #9575, #3503 ) ;
#7060=CARTESIAN_POINT ( 'NONE',  ( -8.964285665223000521, 0.3335619008453594714, 62.14999999999999858 ) ) ;
#7061=DIRECTION ( 'NONE',  ( 0.000000000000000000, 0.000000000000000000, 1.000000000000000000 ) ) ;
#7062=CARTESIAN_POINT ( 'NONE',  ( -24.35918829505000005, 10.97290950744599947, 61.86500000000000199 ) ) ;
#7063=ADVANCED_FACE ( 'NONE', ( #5309 ), #13634, .F. ) ;
#7065=ADVANCED_FACE ( 'NONE', ( #12733 ), #8458, .T. ) ;
#7068=ORIENTED_EDGE ( 'NONE', *, *, #8106, .F. ) ;
#7069=DIRECTION ( 'NONE',  ( -1.000000000000000000, 0.000000000000000000, 0.000000000000000000 ) ) ;
#7070=CARTESIAN_POINT ( 'NONE',  ( -18.88608202933837177, 30.34555471844934615, 61.60507349188181081 ) ) ;
#7071=CONICAL_SURFACE ( 'NONE', #8416, 4.250000000000000000, 0.7853981633974524978 ) ;
#7073=CONICAL_SURFACE ( 'NONE', #8874, 6.145833333000002341, 0.2014252309328122270 ) ;
#7074=DIRECTION ( 'NONE',  ( 1.000000000000000000, 0.000000000000000000, 0.000000000000000000 ) ) ;
#7075=DIRECTION ( 'NONE',  ( 1.000000000000000000, 0.000000000000000000, 0.000000000000000000 ) ) ;
#7076=AXIS2_PLACEMENT_3D ( 'NONE', #10657, #1085, #41 ) ;
#7079=ORIENTED_EDGE ( 'NONE', *, *, #1566, .T. ) ;
#7081=EDGE_CURVE ( 'NONE', #12302, #5689, #8714, .T. ) ;
#7084=CARTESIAN_POINT ( 'NONE',  ( -25.67727386805000123, 10.97290950744599947, 61.65955166399999854 ) ) ;
#7087=CARTESIAN_POINT ( 'NONE',  ( 0.09777679598749960954, -1.420146627243658033, 7.250000000000000000 ) ) ;
#7093=FACE_OUTER_BOUND ( 'NONE', #1962, .T. ) ;
#7094=CARTESIAN_POINT ( 'NONE',  ( -25.86749127492454647, -8.860076549334129581, 17.25000000000000000 ) ) ;
#7095=CARTESIAN_POINT ( 'NONE',  ( -18.05918829504999934, 10.97290950744599947, 67.84999999999999432 ) ) ;
#7098=AXIS2_PLACEMENT_3D ( 'NONE', #8913, #2445, #261 ) ;
#7101=VERTEX_POINT ( 'NONE', #7450 ) ;
#7102=VERTEX_POINT ( 'NONE', #13759 ) ;
#7103=DIRECTION ( 'NONE',  ( -1.000000000000000000, 0.000000000000000000, 0.000000000000000000 ) ) ;
#7104=EDGE_CURVE ( 'NONE', #11891, #11645, #12597, .T. ) ;
#7105=ADVANCED_FACE ( 'NONE', ( #3045 ), #1344, .F. ) ;
#7108=DIRECTION ( 'NONE',  ( -1.000000000000000000, 0.000000000000000000, 0.000000000000000000 ) ) ;
#7110=DIRECTION ( 'NONE',  ( 0.000000000000000000, 0.000000000000000000, -1.000000000000000000 ) ) ;
#7112=CARTESIAN_POINT ( 'NONE',  ( -11.74835982676941981, -4.028726038184999858, 62.14999999999999858 ) ) ;
#7113=CONICAL_SURFACE ( 'NONE', #10914, 6.145833333000000565, 0.7853981633974503884 ) ;
#7114=CIRCLE ( 'NONE', #4903, 33.00000000000000000 ) ;
#7115=ORIENTED_EDGE ( 'NONE', *, *, #13565, .T. ) ;
#7116=ORIENTED_EDGE ( 'NONE', *, *, #4784, .T. ) ;
#7117=CARTESIAN_POINT ( 'NONE',  ( -14.30862101885204218, 30.05623439619531467, 58.39394286420760949 ) ) ;
#7119=ORIENTED_EDGE ( 'NONE', *, *, #12786, .F. ) ;
#7121=ORIENTED_EDGE ( 'NONE', *, *, #767, .F. ) ;
#7122=DIRECTION ( 'NONE',  ( -1.000000000000000000, 0.000000000000000000, 0.000000000000000000 ) ) ;
#7123=CARTESIAN_POINT ( 'NONE',  ( -18.05918829504998513, 2.672909507137216867, 63.26715728756901314 ) ) ;
#7124=EDGE_LOOP ( 'NONE', ( #4615, #11413, #5029, #8848 ) ) ;
#7125=LINE ( 'NONE', #12447, #2219 ) ;
#7127=ADVANCED_FACE ( 'NONE', ( #11742, #78 ), #11540, .F. ) ;
#7129=CIRCLE ( 'NONE', #4250, 4.250000000000000000 ) ;
#7130=CARTESIAN_POINT ( 'NONE',  ( -35.05918829505000645, -6.027090492554000534, 17.25000000000000000 ) ) ;
#7131=CONICAL_SURFACE ( 'NONE', #10056, 4.250000000000000000, 0.7853981633974524978 ) ;
#7132=FACE_OUTER_BOUND ( 'NONE', #2453, .T. ) ;
#7135=ADVANCED_FACE ( 'NONE', ( #6367, #8593 ), #4351, .T. ) ;
#7136=ORIENTED_EDGE ( 'NONE', *, *, #6665, .T. ) ;
#7139=CIRCLE ( 'NONE', #6479, 5.500000000000000888 ) ;
#7140=VECTOR ( 'NONE', #9859, 1000.000000000000114 ) ;
#7142=EDGE_CURVE ( 'NONE', #5559, #3451, #6152, .T. ) ;
#7143=ORIENTED_EDGE ( 'NONE', *, *, #10617, .F. ) ;
#7144=ORIENTED_EDGE ( 'NONE', *, *, #12034, .T. ) ;
#7146=CARTESIAN_POINT ( 'NONE',  ( -18.32176785559807541, 30.36027202460865482, 61.70913974837018401 ) ) ;
#7147=DIRECTION ( 'NONE',  ( -0.9496839325805428444, -0.3132098788326364569, 0.000000000000000000 ) ) ;
#7148=DIRECTION ( 'NONE',  ( 0.000000000000000000, 0.000000000000000000, 1.000000000000000000 ) ) ;
#7155=EDGE_CURVE ( 'NONE', #7831, #6311, #4483, .T. ) ;
#7159=ORIENTED_EDGE ( 'NONE', *, *, #13532, .T. ) ;
#7160=ORIENTED_EDGE ( 'NONE', *, *, #11090, .T. ) ;
#7162=DIRECTION ( 'NONE',  ( 0.000000000000000000, 0.000000000000000000, -1.000000000000000000 ) ) ;
#7164=DIRECTION ( 'NONE',  ( -0.6615960714621569316, 0.7498604124941125049, 0.000000000000000000 ) ) ;
#7165=DIRECTION ( 'NONE',  ( 0.000000000000000000, 0.000000000000000000, 1.000000000000000000 ) ) ;
#7166=CARTESIAN_POINT ( 'NONE',  ( -18.05918829504999934, 10.97290950744599947, 57.35000000000000142 ) ) ;
#7168=EDGE_CURVE ( 'NONE', #6678, #10600, #5242, .T. ) ;
#7170=SURFACE_STYLE_USAGE ( .BOTH. , #9344 ) ;
#7173=ORIENTED_EDGE ( 'NONE', *, *, #7568, .T. ) ;
#7175=ORIENTED_EDGE ( 'NONE', *, *, #4060, .F. ) ;
#7176=CARTESIAN_POINT ( 'NONE',  ( -20.45106689899080976, 15.53048109713862246, 68.70606566337372101 ) ) ;
#7177=CIRCLE ( 'NONE', #7846, 16.66282263685194920 ) ;
#7180=CYLINDRICAL_SURFACE ( 'NONE', #11340, 4.750000000000000888 ) ;
#7182=ADVANCED_FACE ( 'NONE', ( #360 ), #7604, .T. ) ;
#7183=VECTOR ( 'NONE', #312, 1000.000000000000114 ) ;
#7184=ORIENTED_EDGE ( 'NONE', *, *, #4987, .F. ) ;
#7185=CARTESIAN_POINT ( 'NONE',  ( -15.16757089999424402, 30.17981166147537309, 60.20239525771318512 ) ) ;
#7186=ORIENTED_EDGE ( 'NONE', *, *, #3044, .F. ) ;
#7187=DIRECTION ( 'NONE',  ( 0.000000000000000000, 0.000000000000000000, 1.000000000000000000 ) ) ;
#7189=CARTESIAN_POINT ( 'NONE',  ( -18.05918829249644730, 2.672909507443099741, 63.15000000009349179 ) ) ;
#7190=ORIENTED_EDGE ( 'NONE', *, *, #1133, .T. ) ;
#7192=DIRECTION ( 'NONE',  ( -1.000000000000000000, 0.000000000000000000, 0.000000000000000000 ) ) ;
#7197=DIRECTION ( 'NONE',  ( 0.000000000000000000, 0.000000000000000000, -1.000000000000000000 ) ) ;
#7202=AXIS2_PLACEMENT_3D ( 'NONE', #2536, #6767, #11039 ) ;
#7203=ORIENTED_EDGE ( 'NONE', *, *, #8335, .F. ) ;
#7206=EDGE_LOOP ( 'NONE', ( #12111, #5246, #5519, #5081 ) ) ;
#7209=CYLINDRICAL_SURFACE ( 'NONE', #12345, 4.250000000000000000 ) ;
#7214=AXIS2_PLACEMENT_3D ( 'NONE', #6173, #321, #11977 ) ;
#7219=EDGE_LOOP ( 'NONE', ( #3702, #5314, #8340, #7277 ) ) ;
#7222=CARTESIAN_POINT ( 'NONE',  ( -23.05918829504999934, 10.97290950744599947, 116.8499999999999943 ) ) ;
#7226=CARTESIAN_POINT ( 'NONE',  ( -10.25088531517539714, 30.80589556422609832, 17.25000000000000000 ) ) ;
#7230=AXIS2_PLACEMENT_3D ( 'NONE', #12317, #1618, #13217 ) ;
#7232=EDGE_CURVE ( 'NONE', #10781, #1636, #7139, .T. ) ;
#7235=EDGE_LOOP ( 'NONE', ( #8655, #2007, #22, #8672, #9573 ) ) ;
#7236=VERTEX_POINT ( 'NONE', #213 ) ;
#7237=CARTESIAN_POINT ( 'NONE',  ( -11.74835982676941981, -4.028726038184999858, 63.45000000000000284 ) ) ;
#7243=VERTEX_POINT ( 'NONE', #2413 ) ;
#7244=VECTOR ( 'NONE', #11764, 1000.000000000000000 ) ;
#7245=EDGE_CURVE ( 'NONE', #7236, #8398, #1332, .T. ) ;
#7246=CARTESIAN_POINT ( 'NONE',  ( -14.93697936199538034, 30.14955231555997273, 59.86459082872807613 ) ) ;
#7247=ORIENTED_EDGE ( 'NONE', *, *, #13338, .F. ) ;
#7249=DIRECTION ( 'NONE',  ( 1.000000000000000000, 0.000000000000000000, 0.000000000000000000 ) ) ;
#7250=DIRECTION ( 'NONE',  ( 0.000000000000000000, 0.000000000000000000, -1.000000000000000000 ) ) ;
#7251=DIRECTION ( 'NONE',  ( 0.000000000000000000, 0.000000000000000000, 1.000000000000000000 ) ) ;
#7252=ORIENTED_EDGE ( 'NONE', *, *, #1410, .F. ) ;
#7253=CYLINDRICAL_SURFACE ( 'NONE', #6868, 24.92993838181874722 ) ;
#7255=EDGE_LOOP ( 'NONE', ( #7003, #10074, #13200, #6772 ) ) ;
#7256=FACE_OUTER_BOUND ( 'NONE', #4566, .T. ) ;
#7257=CARTESIAN_POINT ( 'NONE',  ( -18.05918829504999934, 10.97290950744599947, 68.84999999999999432 ) ) ;
#7259=VECTOR ( 'NONE', #10622, 1000.000000000000000 ) ;
#7262=VERTEX_POINT ( 'NONE', #5588 ) ;
#7263=ORIENTED_EDGE ( 'NONE', *, *, #10027, .F. ) ;
#7264=ORIENTED_EDGE ( 'NONE', *, *, #10617, .T. ) ;
#7265=CIRCLE ( 'NONE', #4838, 0.9499999999999995115 ) ;
#7269=DIRECTION ( 'NONE',  ( 1.000000000000000000, 0.000000000000000000, 0.000000000000000000 ) ) ;
#7270=CARTESIAN_POINT ( 'NONE',  ( -18.91658168612351787, 30.34444651895818268, 61.59715132800811688 ) ) ;
#7274=FACE_OUTER_BOUND ( 'NONE', #2420, .T. ) ;
#7275=ORIENTED_EDGE ( 'NONE', *, *, #13758, .T. ) ;
#7276=VECTOR ( 'NONE', #8996, 1000.000000000000000 ) ;
#7277=ORIENTED_EDGE ( 'NONE', *, *, #5327, .F. ) ;
#7280=ORIENTED_EDGE ( 'NONE', *, *, #1227, .T. ) ;
#7287=EDGE_LOOP ( 'NONE', ( #7115, #6332 ) ) ;
#7288=FACE_OUTER_BOUND ( 'NONE', #6213, .T. ) ;
#7291=CARTESIAN_POINT ( 'NONE',  ( -10.89307956596845983, 10.97290950744599947, 61.72253826518770836 ) ) ;
#7292=AXIS2_PLACEMENT_3D ( 'NONE', #2046, #4129, #12711 ) ;
#7293=AXIS2_PLACEMENT_3D ( 'NONE', #13250, #4598, #12000 ) ;
#7294=VERTEX_POINT ( 'NONE', #4486 ) ;
#7295=VECTOR ( 'NONE', #6580, 1000.000000000000000 ) ;
#7296=VERTEX_POINT ( 'NONE', #11811 ) ;
#7297=VERTEX_POINT ( 'NONE', #8742 ) ;
#7301=CARTESIAN_POINT ( 'NONE',  ( -20.12305801176480813, 15.81988081417610381, 68.58194257568855789 ) ) ;
#7302=ORIENTED_EDGE ( 'NONE', *, *, #11954, .T. ) ;
#7303=CARTESIAN_POINT ( 'NONE',  ( -11.74835982676941981, -4.028726038184999858, 62.14999999999999858 ) ) ;
#7306=VECTOR ( 'NONE', #12802, 1000.000000000000114 ) ;
#7308=CARTESIAN_POINT ( 'NONE',  ( -25.73489962141544751, -4.139534227248430120, 57.54999999999999716 ) ) ;
#7310=CARTESIAN_POINT ( 'NONE',  ( -25.29804148384604900, -2.574630058508220021, 62.14999999999999858 ) ) ;
#7312=ADVANCED_FACE ( 'NONE', ( #1881 ), #3322, .F. ) ;
#7315=EDGE_LOOP ( 'NONE', ( #13035, #1548, #12799, #2702 ) ) ;
#7316=CARTESIAN_POINT ( 'NONE',  ( -14.83031415886561000, 30.13477816397302789, 59.68356427289636912 ) ) ;
#7317=ORIENTED_EDGE ( 'NONE', *, *, #13300, .F. ) ;
#7318=VERTEX_POINT ( 'NONE', #4900 ) ;
#7319=EDGE_CURVE ( 'NONE', #1146, #1530, #6025, .T. ) ;
#7320=CARTESIAN_POINT ( 'NONE',  ( -18.05918829504999934, 10.97290950744599947, 57.35000000000000142 ) ) ;
#7326=CARTESIAN_POINT ( 'NONE',  ( -35.05918829505000645, 10.97290950744599947, 57.35000000000000142 ) ) ;
#7328=CARTESIAN_POINT ( 'NONE',  ( -1.433900126049995061, 19.28555359244599288, 63.26601075299999621 ) ) ;
#7332=ORIENTED_EDGE ( 'NONE', *, *, #12628, .T. ) ;
#7333=EDGE_LOOP ( 'NONE', ( #7610, #12376, #2568, #1323 ) ) ;
#7334=AXIS2_PLACEMENT_3D ( 'NONE', #12230, #3710, #3507 ) ;
#7335=CONICAL_SURFACE ( 'NONE', #9149, 6.595833333000001630, 0.4098752297613067475 ) ;
#7338=CARTESIAN_POINT ( 'NONE',  ( -28.87730642030694028, 29.81324547859995278, 17.25000000000000000 ) ) ;
#7339=CARTESIAN_POINT ( 'NONE',  ( -19.31260878079642751, 26.92505106486307298, 56.52244572334543449 ) ) ;
#7340=CARTESIAN_POINT ( 'NONE',  ( -5.809188295050001116, 27.97290950744599769, 7.250000000000000000 ) ) ;
#7344=CONICAL_SURFACE ( 'NONE', #6023, 6.595833333000001630, 0.4098752297613067475 ) ;
#7347=AXIS2_PLACEMENT_3D ( 'NONE', #1315, #2464, #4396 ) ;
#7349=ORIENTED_EDGE ( 'NONE', *, *, #9102, .T. ) ;
#7352=ORIENTED_EDGE ( 'NONE', *, *, #5867, .T. ) ;
#7353=DIRECTION ( 'NONE',  ( 0.000000000000000000, 0.5150380749100549327, 0.8571673007021118895 ) ) ;
#7354=DIRECTION ( 'NONE',  ( -1.000000000000000000, 0.000000000000000000, 0.000000000000000000 ) ) ;
#7356=AXIS2_PLACEMENT_3D ( 'NONE', #9375, #3037, #7251 ) ;
#7357=AXIS2_PLACEMENT_3D ( 'NONE', #7303, #3982, #13741 ) ;
#7360=CARTESIAN_POINT ( 'NONE',  ( -30.32854245105399826, -5.598733283342819611, 7.250000000000000000 ) ) ;
#7361=VECTOR ( 'NONE', #1944, 1000.000000000000000 ) ;
#7362=CARTESIAN_POINT ( 'NONE',  ( -12.62505638257885998, 21.67198471784914915, 62.85000000000000142 ) ) ;
#7364=DIRECTION ( 'NONE',  ( 1.000000000000000000, 0.000000000000000000, 0.000000000000000000 ) ) ;
#7365=ADVANCED_FACE ( 'NONE', ( #10212 ), #628, .T. ) ;
#7366=ORIENTED_EDGE ( 'NONE', *, *, #6002, .F. ) ;
#7371=ORIENTED_EDGE ( 'NONE', *, *, #13715, .T. ) ;
#7372=EDGE_LOOP ( 'NONE', ( #5178, #12764, #10523, #4957 ) ) ;
#7374=EDGE_LOOP ( 'NONE', ( #13736, #4907, #10501, #13258 ) ) ;
#7375=FACE_OUTER_BOUND ( 'NONE', #2649, .T. ) ;
#7376=CARTESIAN_POINT ( 'NONE',  ( -14.08961186627706041, 6.473747032481329988, 31.09999999999999787 ) ) ;
#7377=CARTESIAN_POINT ( 'NONE',  ( -11.91335496205000055, 10.97290950744599947, 60.60999999999999943 ) ) ;
#7378=CARTESIAN_POINT ( 'NONE',  ( -16.01484020223730553, 6.108714422173897596, 68.57364943554455294 ) ) ;
#7380=DIRECTION ( 'NONE',  ( -1.000000000000000000, 0.000000000000000000, 0.000000000000000000 ) ) ;
#7384=CYLINDRICAL_SURFACE ( 'NONE', #5896, 18.00000000000000000 ) ;
#7386=ORIENTED_EDGE ( 'NONE', *, *, #6001, .F. ) ;
#7389=EDGE_CURVE ( 'NONE', #8708, #8341, #9936, .T. ) ;
#7390=EDGE_CURVE ( 'NONE', #13422, #5137, #2144, .T. ) ;
#7393=CARTESIAN_POINT ( 'NONE',  ( -9.143292286380720668, 6.444466247053390440, 64.85000000000000853 ) ) ;
#7395=CARTESIAN_POINT ( 'NONE',  ( -41.50918829505000218, 27.97290950744599769, 17.25000000000000000 ) ) ;
#7397=ADVANCED_FACE ( 'NONE', ( #11187 ), #13488, .T. ) ;
#7399=EDGE_LOOP ( 'NONE', ( #11945, #3158, #9148, #8568 ) ) ;
#7400=VERTEX_POINT ( 'NONE', #9077 ) ;
#7405=ORIENTED_EDGE ( 'NONE', *, *, #4901, .T. ) ;
#7406=CARTESIAN_POINT ( 'NONE',  ( -25.33503448090910126, 29.19143287883919768, 64.85000000000000853 ) ) ;
#7408=CARTESIAN_POINT ( 'NONE',  ( -12.54628844161313950, -7.366404416634599883, 62.14999999999999858 ) ) ;
#7409=CARTESIAN_POINT ( 'NONE',  ( -18.97262203685356141, 26.94685435944512264, 56.15999655357090603 ) ) ;
#7411=DIRECTION ( 'NONE',  ( -1.000000000000000000, 0.000000000000000000, 0.000000000000000000 ) ) ;
#7413=VECTOR ( 'NONE', #13525, 1000.000000000000000 ) ;
#7414=ORIENTED_EDGE ( 'NONE', *, *, #584, .T. ) ;
#7415=ORIENTED_EDGE ( 'NONE', *, *, #3910, .T. ) ;
#7416=EDGE_CURVE ( 'NONE', #3005, #6052, #13053, .T. ) ;
#7417=CARTESIAN_POINT ( 'NONE',  ( 1.629816981350590055, -4.941769416738769571, 5.250000000000000000 ) ) ;
#7422=CARTESIAN_POINT ( 'NONE',  ( -20.55028075881694249, 30.22631440511032963, 54.04780568389777073 ) ) ;
#7425=CARTESIAN_POINT ( 'NONE',  ( -2.819094421049990640, 18.59295644444599915, 61.63595870799996845 ) ) ;
#7427=CARTESIAN_POINT ( 'NONE',  ( -18.05918829505000289, 18.55161869500264515, 61.95399527332316580 ) ) ;
#7428=DIRECTION ( 'NONE',  ( 0.000000000000000000, 0.000000000000000000, 1.000000000000000000 ) ) ;
#7429=ORIENTED_EDGE ( 'NONE', *, *, #11318, .F. ) ;
#7430=CARTESIAN_POINT ( 'NONE',  ( -18.05918829504999934, 10.97290950744599947, 62.85000000000000142 ) ) ;
#7431=ORIENTED_EDGE ( 'NONE', *, *, #13603, .F. ) ;
#7432=CARTESIAN_POINT ( 'NONE',  ( -7.241070169793070832, 29.81324547859995278, 17.25000000000000000 ) ) ;
#7433=CARTESIAN_POINT ( 'NONE',  ( -28.87730642030695094, -7.867426463707980488, 17.25000000000000000 ) ) ;
#7434=VERTEX_POINT ( 'NONE', #7891 ) ;
#7435=PRESENTATION_STYLE_ASSIGNMENT (( #3351 ) ) ;
#7436=EDGE_CURVE ( 'NONE', #7790, #13237, #3471, .T. ) ;
#7437=DIRECTION ( 'NONE',  ( 1.000000000000000000, 0.000000000000000000, 0.000000000000000000 ) ) ;
#7438=EDGE_CURVE ( 'NONE', #6850, #3038, #6120, .T. ) ;
#7440=AXIS2_PLACEMENT_3D ( 'NONE', #9231, #13483, #12435 ) ;
#7442=CARTESIAN_POINT ( 'NONE',  ( -16.48613393974217090, 30.30694957908812270, 53.37988226775320300 ) ) ;
#7443=VECTOR ( 'NONE', #4259, 1000.000000000000000 ) ;
#7444=CYLINDRICAL_SURFACE ( 'NONE', #10283, 6.449999999999997513 ) ;
#7445=CARTESIAN_POINT ( 'NONE',  ( -10.25088531517539892, 30.80589556422609832, 17.25000000000000000 ) ) ;
#7446=DIRECTION ( 'NONE',  ( 0.000000000000000000, 0.000000000000000000, -1.000000000000000000 ) ) ;
#7447=CARTESIAN_POINT ( 'NONE',  ( -18.05918829504999934, 14.81548537210212046, 17.25000000000000000 ) ) ;
#7448=EDGE_CURVE ( 'NONE', #7735, #10798, #10163, .T. ) ;
#7449=CARTESIAN_POINT ( 'NONE',  ( -35.72201093190194854, 10.97290950744599947, 6.250000000000000000 ) ) ;
#7450=CARTESIAN_POINT ( 'NONE',  ( -9.663354962050000552, 10.97290950744599947, 60.04999999999999716 ) ) ;
#7451=EDGE_CURVE ( 'NONE', #6, #5283, #11710, .T. ) ;
#7452=VECTOR ( 'NONE', #8843, 1000.000000000000000 ) ;
#7453=ADVANCED_FACE ( 'NONE', ( #8812 ), #1262, .T. ) ;
#7455=CYLINDRICAL_SURFACE ( 'NONE', #2586, 17.00000000000000000 ) ;
#7456=ORIENTED_EDGE ( 'NONE', *, *, #2366, .T. ) ;
#7457=ORIENTED_EDGE ( 'NONE', *, *, #9180, .T. ) ;
#7461=ADVANCED_FACE ( 'NONE', ( #8671 ), #4294, .F. ) ;
#7463=AXIS2_PLACEMENT_3D ( 'NONE', #13380, #10449, #9413 ) ;
#7469=LINE ( 'NONE', #11760, #451 ) ;
#7471=CIRCLE ( 'NONE', #800, 34.70000000000000284 ) ;
#7473=ORIENTED_EDGE ( 'NONE', *, *, #13512, .F. ) ;
#7475=ORIENTED_EDGE ( 'NONE', *, *, #13300, .T. ) ;
#7477=DIRECTION ( 'NONE',  ( 0.2878798879079290662, 0.9576665234506832602, 0.000000000000000000 ) ) ;
#7478=DIRECTION ( 'NONE',  ( 0.000000000000000000, 0.000000000000000000, 1.000000000000000000 ) ) ;
#7479=CARTESIAN_POINT ( 'NONE',  ( -20.69640587970463486, 30.21012672718795855, 54.19793656979756236 ) ) ;
#7482=DIRECTION ( 'NONE',  ( 0.000000000000000000, 0.000000000000000000, -1.000000000000000000 ) ) ;
#7484=PLANE ( 'NONE',  #9621 ) ;
#7488=EDGE_CURVE ( 'NONE', #5579, #6589, #12818, .T. ) ;
#7492=CARTESIAN_POINT ( 'NONE',  ( -23.57208814848684852, -7.366404416634599883, 62.14999999999999858 ) ) ;
#7494=ORIENTED_EDGE ( 'NONE', *, *, #1282, .T. ) ;
#7498=DIRECTION ( 'NONE',  ( 1.000000000000000000, 0.000000000000000000, 0.000000000000000000 ) ) ;
#7499=CARTESIAN_POINT ( 'NONE',  ( -18.05918829504999934, 10.97290950744599947, 5.250000000000000000 ) ) ;
#7500=DIRECTION ( 'NONE',  ( 1.000000000000000000, 0.000000000000000000, 0.000000000000000000 ) ) ;
#7502=DIRECTION ( 'NONE',  ( -0.6615960714621564875, 0.7498604124941129490, 0.000000000000000000 ) ) ;
#7504=CIRCLE ( 'NONE', #9323, 16.95000000000000284 ) ;
#7505=VECTOR ( 'NONE', #7849, 1000.000000000000114 ) ;
#7506=ADVANCED_FACE ( 'NONE', ( #2201 ), #12797, .T. ) ;
#7508=EDGE_CURVE ( 'NONE', #8435, #4307, #6795, .T. ) ;
#7510=AXIS2_PLACEMENT_3D ( 'NONE', #903, #10279, #8242 ) ;
#7512=AXIS2_PLACEMENT_3D ( 'NONE', #4678, #8933, #13190 ) ;
#7513=ORIENTED_EDGE ( 'NONE', *, *, #11023, .F. ) ;
#7514=ORIENTED_EDGE ( 'NONE', *, *, #2906, .F. ) ;
#7515=CARTESIAN_POINT ( 'NONE',  ( -10.79835982676942052, -4.028726038184999858, 62.14999999999999858 ) ) ;
#7516=AXIS2_PLACEMENT_3D ( 'NONE', #1480, #8754, #1347 ) ;
#7518=SURFACE_STYLE_FILL_AREA ( #11950 ) ;
#7522=DIRECTION ( 'NONE',  ( 0.000000000000000000, 0.000000000000000000, -1.000000000000000000 ) ) ;
#7523=CIRCLE ( 'NONE', #11580, 16.72262947720610171 ) ;
#7524=VECTOR ( 'NONE', #3506, 1000.000000000000114 ) ;
#7530=ORIENTED_EDGE ( 'NONE', *, *, #12273, .F. ) ;
#7531=( BOUNDED_SURFACE ( )  B_SPLINE_SURFACE ( 3, 3, ( 
 ( #2374, #8624, #12961, #4450 ),
 ( #44, #105, #8776, #6598 ),
 ( #1088, #5548, #4379, #10808 ),
 ( #4522, #11773, #7425, #9751 ) ),
 .UNSPECIFIED., .F., .F., .T. ) 
 B_SPLINE_SURFACE_WITH_KNOTS ( ( 4, 4 ),
 ( 4, 4 ),
 ( 0.000000000000000000, 1.000000000000000000 ),
 ( 0.000000000000000000, 1.000000000000000000 ),
 .UNSPECIFIED. ) 
 GEOMETRIC_REPRESENTATION_ITEM ( )  RATIONAL_B_SPLINE_SURFACE ( (
 ( 1.000000000000000000, 0.3333333333333329818, 0.3333333333333329818, 1.000000000000000000),
 ( 0.4470472315060959878, 0.1490157438353659769, 0.1490157438353659769, 0.4470472315060959878),
 ( 0.4470472315060959878, 0.1490157438353659769, 0.1490157438353659769, 0.4470472315060959878),
 ( 1.000000000000000000, 0.3333333333333329818, 0.3333333333333329818, 1.000000000000000000) ) ) 
 REPRESENTATION_ITEM ( '' )  SURFACE ( )  );
#7534=EDGE_LOOP ( 'NONE', ( #11890, #5656, #5479, #879 ) ) ;
#7538=CARTESIAN_POINT ( 'NONE',  ( -5.809188295050001116, 27.97290950744599769, 64.85000000000000853 ) ) ;
#7539=ORIENTED_EDGE ( 'NONE', *, *, #8564, .T. ) ;
#7540=CARTESIAN_POINT ( 'NONE',  ( 0.000000000000000000, 0.000000000000000000, 5.250000000000000000 ) ) ;
#7545=CARTESIAN_POINT ( 'NONE',  ( -25.64433075620760150, -3.961216307075045240, 61.85000000000000142 ) ) ;
#7550=VECTOR ( 'NONE', #9755, 1000.000000000000114 ) ;
#7552=ORIENTED_EDGE ( 'NONE', *, *, #12631, .T. ) ;
#7553=ORIENTED_EDGE ( 'NONE', *, *, #4225, .T. ) ;
#7554=DIRECTION ( 'NONE',  ( 0.000000000000000000, 0.000000000000000000, -1.000000000000000000 ) ) ;
#7555=VERTEX_POINT ( 'NONE', #5315 ) ;
#7557=CARTESIAN_POINT ( 'NONE',  ( -18.05918829504999934, 10.97290950744599947, 30.59999999999999787 ) ) ;
#7559=CARTESIAN_POINT ( 'NONE',  ( -18.05918829504999934, 30.36027202460864771, 52.99086025162979752 ) ) ;
#7561=CARTESIAN_POINT ( 'NONE',  ( -18.05918829504999934, 10.97290950744599947, 62.14999999999999858 ) ) ;
#7565=CIRCLE ( 'NONE', #13599, 6.749999999999999112 ) ;
#7566=VECTOR ( 'NONE', #10695, 1000.000000000000000 ) ;
#7568=EDGE_CURVE ( 'NONE', #12316, #10704, #5385, .T. ) ;
#7569=ORIENTED_EDGE ( 'NONE', *, *, #12372, .T. ) ;
#7572=VECTOR ( 'NONE', #7477, 1000.000000000000227 ) ;
#7573=DIRECTION ( 'NONE',  ( 0.2878798879079290662, 0.9576665234506832602, 0.000000000000000000 ) ) ;
#7575=AXIS2_PLACEMENT_3D ( 'NONE', #5841, #6822, #3634 ) ;
#7576=AXIS2_PLACEMENT_3D ( 'NONE', #12794, #11615, #9658 ) ;
#7578=ORIENTED_EDGE ( 'NONE', *, *, #1439, .T. ) ;
#7582=ADVANCED_FACE ( 'NONE', ( #3303 ), #7455, .F. ) ;
#7583=DIRECTION ( 'NONE',  ( -1.000000000000000000, 0.000000000000000000, 0.000000000000000000 ) ) ;
#7584=CARTESIAN_POINT ( 'NONE',  ( -1.059188295049996231, 27.97290950744599769, 58.85000000000000142 ) ) ;
#7586=FACE_OUTER_BOUND ( 'NONE', #4139, .T. ) ;
#7587=CARTESIAN_POINT ( 'NONE',  ( -30.32854245105399826, 27.54455229823479812, 7.250000000000000000 ) ) ;
#7588=CARTESIAN_POINT ( 'NONE',  ( -10.25088531517540069, -8.860076549334108265, 83.57661607529820458 ) ) ;
#7590=CONICAL_SURFACE ( 'NONE', #1584, 4.546599999999997976, 1.029744258676653645 ) ;
#7591=VECTOR ( 'NONE', #9905, 1000.000000000000114 ) ;
#7592=ORIENTED_EDGE ( 'NONE', *, *, #8942, .F. ) ;
#7593=CARTESIAN_POINT ( 'NONE',  ( -16.42191933243140056, 30.30251685243779036, 53.41373514583168713 ) ) ;
#7594=VERTEX_POINT ( 'NONE', #13072 ) ;
#7600=ORIENTED_EDGE ( 'NONE', *, *, #8564, .F. ) ;
#7603=EDGE_CURVE ( 'NONE', #12804, #6443, #12607, .T. ) ;
#7604=CYLINDRICAL_SURFACE ( 'NONE', #12729, 34.69999999999999574 ) ;
#7605=AXIS2_PLACEMENT_3D ( 'NONE', #7499, #4334, #9562 ) ;
#7608=ORIENTED_EDGE ( 'NONE', *, *, #10133, .F. ) ;
#7610=ORIENTED_EDGE ( 'NONE', *, *, #13673, .F. ) ;
#7614=DIRECTION ( 'NONE',  ( 0.000000000000000000, -1.000000000000000000, 2.732534507816519619E-15 ) ) ;
#7616=CARTESIAN_POINT ( 'NONE',  ( -1.396365658198039927, 10.97290950744599947, 5.250000000000000000 ) ) ;
#7617=STYLED_ITEM ( 'NONE', ( #3207 ), #5147 ) ;
#7618=CARTESIAN_POINT ( 'NONE',  ( -16.68844204839930612, 26.91524980442654069, 56.72172238493448049 ) ) ;
#7619=EDGE_CURVE ( 'NONE', #10997, #10707, #10964, .T. ) ;
#7620=CARTESIAN_POINT ( 'NONE',  ( -38.38077571930825371, 22.44393519180574970, 17.25000000000000000 ) ) ;
#7621=DIRECTION ( 'NONE',  ( 0.000000000000000000, 0.000000000000000000, -1.000000000000000000 ) ) ;
#7622=EDGE_CURVE ( 'NONE', #9965, #1818, #6513, .T. ) ;
#7623=DIRECTION ( 'NONE',  ( -1.000000000000000000, 0.000000000000000000, 0.000000000000000000 ) ) ;
#7626=ORIENTED_EDGE ( 'NONE', *, *, #2816, .F. ) ;
#7627=COLOUR_RGB ( '', 0.31764706, 0.68627451, 0.89019608) ;
#7630=EDGE_LOOP ( 'NONE', ( #2315, #12917, #3145, #2469 ) ) ;
#7632=CARTESIAN_POINT ( 'NONE',  ( -11.74835982676941981, -4.028726038184999858, 62.14999999999999858 ) ) ;
#7634=DIRECTION ( 'NONE',  ( 0.000000000000000000, 0.000000000000000000, -1.000000000000000000 ) ) ;
#7636=CARTESIAN_POINT ( 'NONE',  ( -18.19063477396443318, 30.36027202460863705, 52.99086025162979752 ) ) ;
#7637=VERTEX_POINT ( 'NONE', #6782 ) ;
#7642=VECTOR ( 'NONE', #13632, 1000.000000000000114 ) ;
#7644=EDGE_CURVE ( 'NONE', #2345, #467, #6574, .T. ) ;
#7645=EDGE_CURVE ( 'NONE', #11014, #2826, #13344, .T. ) ;
#7646=ORIENTED_EDGE ( 'NONE', *, *, #5349, .F. ) ;
#7649=EDGE_LOOP ( 'NONE', ( #3771, #3093, #5866, #2041 ) ) ;
#7654=CARTESIAN_POINT ( 'NONE',  ( -18.05918829504999934, 10.97290950744599947, 60.04999999999999716 ) ) ;
#7656=FACE_OUTER_BOUND ( 'NONE', #12441, .T. ) ;
#7658=EDGE_CURVE ( 'NONE', #6311, #7831, #4136, .T. ) ;
#7659=CARTESIAN_POINT ( 'NONE',  ( -26.35918829505000005, 10.97290950744599947, 61.86500000000000199 ) ) ;
#7660=DIRECTION ( 'NONE',  ( 0.000000000000000000, 0.000000000000000000, 1.000000000000000000 ) ) ;
#7661=ADVANCED_FACE ( 'NONE', ( #9937 ), #8959, .F. ) ;
#7662=ORIENTED_EDGE ( 'NONE', *, *, #10144, .T. ) ;
#7663=CARTESIAN_POINT ( 'NONE',  ( -16.95433748440508737, 30.33404188113821931, 53.17780894285112225 ) ) ;
#7665=DIRECTION ( 'NONE',  ( 0.000000000000000000, 0.000000000000000000, -1.000000000000000000 ) ) ;
#7666=CARTESIAN_POINT ( 'NONE',  ( -12.54628844161313950, -7.366404416634599883, 62.14999999999999858 ) ) ;
#7668=CARTESIAN_POINT ( 'NONE',  ( -18.05918829504999934, 19.27191034044600215, 63.13003331699999876 ) ) ;
#7670=ADVANCED_FACE ( 'NONE', ( #8037 ), #9708, .F. ) ;
#7671=ADVANCED_FACE ( 'NONE', ( #4905 ), #13141, .F. ) ;
#7672=EDGE_LOOP ( 'NONE', ( #2765, #11131, #9328, #7514 ) ) ;
#7676=ORIENTED_EDGE ( 'NONE', *, *, #10330, .T. ) ;
#7677=EDGE_LOOP ( 'NONE', ( #3956, #13646 ) ) ;
#7678=ORIENTED_EDGE ( 'NONE', *, *, #3893, .F. ) ;
#7682=ORIENTED_EDGE ( 'NONE', *, *, #5883, .F. ) ;
#7684=CARTESIAN_POINT ( 'NONE',  ( -17.20223088790494970, 26.94994329434792490, 56.11889009176745446 ) ) ;
#7685=DIRECTION ( 'NONE',  ( 0.000000000000000000, 0.000000000000000000, -1.000000000000000000 ) ) ;
#7686=CYLINDRICAL_SURFACE ( 'NONE', #7828, 4.250000000000000000 ) ;
#7687=AXIS2_PLACEMENT_3D ( 'NONE', #4689, #11247, #3576 ) ;
#7691=EDGE_CURVE ( 'NONE', #5675, #11446, #12716, .T. ) ;
#7692=ORIENTED_EDGE ( 'NONE', *, *, #9365, .F. ) ;
#7694=ADVANCED_FACE ( 'NONE', ( #3169 ), #7384, .F. ) ;
#7695=AXIS2_PLACEMENT_3D ( 'NONE', #13309, #8004, #12275 ) ;
#7699=DIRECTION ( 'NONE',  ( 1.000000000000000000, 0.000000000000000000, 0.000000000000000000 ) ) ;
#7700=DIRECTION ( 'NONE',  ( 0.000000000000000000, 0.000000000000000000, -1.000000000000000000 ) ) ;
#7701=DIRECTION ( 'NONE',  ( -0.9496839325805416232, -0.3132098788326400096, 0.000000000000000000 ) ) ;
#7703=CARTESIAN_POINT ( 'NONE',  ( -35.72201093190194854, 10.97290950744599947, 7.250000000000000000 ) ) ;
#7706=CYLINDRICAL_SURFACE ( 'NONE', #215, 2.700000000000001066 ) ;
#7711=ORIENTED_EDGE ( 'NONE', *, *, #3076, .F. ) ;
#7712=PLANE ( 'NONE',  #582 ) ;
#7714=ORIENTED_EDGE ( 'NONE', *, *, #4589, .T. ) ;
#7717=EDGE_LOOP ( 'NONE', ( #11198, #11106 ) ) ;
#7719=EDGE_CURVE ( 'NONE', #10426, #8976, #2825, .T. ) ;
#7722=DIRECTION ( 'NONE',  ( -1.000000000000000000, 7.097562450402079698E-15, 0.000000000000000000 ) ) ;
#7724=DIRECTION ( 'NONE',  ( -0.2148617826751194892, -2.631297944121794810E-17, -0.9766444667050899753 ) ) ;
#7726=CARTESIAN_POINT ( 'NONE',  ( -30.48673169511680214, 10.97290950744599947, 5.250000000000000000 ) ) ;
#7727=EDGE_CURVE ( 'NONE', #9462, #6784, #3925, .T. ) ;
#7730=VECTOR ( 'NONE', #5358, 1000.000000000000114 ) ;
#7734=CARTESIAN_POINT ( 'NONE',  ( -35.05918829505000645, 10.97290950744599947, 62.14999999999999858 ) ) ;
#7735=VERTEX_POINT ( 'NONE', #7734 ) ;
#7741=AXIS2_PLACEMENT_3D ( 'NONE', #3273, #7482, #6468 ) ;
#7742=DIRECTION ( 'NONE',  ( 0.000000000000000000, 0.000000000000000000, -1.000000000000000000 ) ) ;
#7744=CYLINDRICAL_SURFACE ( 'NONE', #11596, 16.66282263685194920 ) ;
#7746=AXIS2_PLACEMENT_3D ( 'NONE', #10933, #1541, #9016 ) ;
#7747=AXIS2_PLACEMENT_3D ( 'NONE', #2459, #4742, #9917 ) ;
#7748=CIRCLE ( 'NONE', #4430, 16.72262947720610171 ) ;
#7750=ORIENTED_EDGE ( 'NONE', *, *, #5596, .F. ) ;
#7751=ADVANCED_FACE ( 'NONE', ( #13058 ), #12156, .F. ) ;
#7752=CONICAL_SURFACE ( 'NONE', #8657, 8.300000000000000711, 0.08573846772804097349 ) ;
#7753=VERTEX_POINT ( 'NONE', #5854 ) ;
#7755=ADVANCED_FACE ( 'NONE', ( #6771 ), #3703, .F. ) ;
#7756=EDGE_LOOP ( 'NONE', ( #13142, #13642 ) ) ;
#7759=CARTESIAN_POINT ( 'NONE',  ( -19.55918829504999934, 28.64232754551664684, 57.35000000000000142 ) ) ;
#7761=VERTEX_POINT ( 'NONE', #493 ) ;
#7762=ADVANCED_FACE ( 'NONE', ( #1459 ), #2605, .T. ) ;
#7764=CARTESIAN_POINT ( 'NONE',  ( -17.08318469166218989, 26.94349457154494232, 56.20301699921735405 ) ) ;
#7766=CIRCLE ( 'NONE', #10020, 7.166108729582679970 ) ;
#7767=CARTESIAN_POINT ( 'NONE',  ( -19.55918829504999934, 27.40458623260099813, 57.35000000000000142 ) ) ;
#7770=DIRECTION ( 'NONE',  ( 0.000000000000000000, 0.000000000000000000, 1.000000000000000000 ) ) ;
#7773=AXIS2_PLACEMENT_3D ( 'NONE', #12192, #1497, #9045 ) ;
#7777=CARTESIAN_POINT ( 'NONE',  ( -21.51338012790479226, 30.10205818035979419, 55.47564455151579210 ) ) ;
#7778=DIRECTION ( 'NONE',  ( 1.000000000000000000, 0.000000000000000000, 0.000000000000000000 ) ) ;
#7779=ORIENTED_EDGE ( 'NONE', *, *, #5578, .F. ) ;
#7780=CARTESIAN_POINT ( 'NONE',  ( -21.79515398487389888, 3.617295300293844829, 60.04999999999999716 ) ) ;
#7781=LINE ( 'NONE', #3681, #10253 ) ;
#7783=DIRECTION ( 'NONE',  ( -1.000000000000000000, 1.075797504481739195E-15, 0.000000000000000000 ) ) ;
#7784=ADVANCED_FACE ( 'NONE', ( #6904 ), #12085, .F. ) ;
#7785=AXIS2_PLACEMENT_3D ( 'NONE', #13228, #9033, #3728 ) ;
#7789=CARTESIAN_POINT ( 'NONE',  ( -9.759188295050000406, 10.97290950744599947, 61.86500000000000199 ) ) ;
#7790=VERTEX_POINT ( 'NONE', #4754 ) ;
#7791=PLANE ( 'NONE',  #3751 ) ;
#7794=AXIS2_PLACEMENT_3D ( 'NONE', #1275, #8688, #10023 ) ;
#7796=DIRECTION ( 'NONE',  ( 0.000000000000000000, 0.000000000000000000, -1.000000000000000000 ) ) ;
#7798=DIRECTION ( 'NONE',  ( 0.000000000000000000, 3.387121092260455192E-15, 1.000000000000000000 ) ) ;
#7799=CARTESIAN_POINT ( 'NONE',  ( -18.05918829504999934, 10.97290950744599947, 63.54999999999999716 ) ) ;
#7801=ADVANCED_FACE ( 'NONE', ( #9011 ), #6969, .T. ) ;
#7802=ADVANCED_FACE ( 'NONE', ( #9991, #8022 ), #12301, .T. ) ;
#7804=VECTOR ( 'NONE', #12841, 1000.000000000000114 ) ;
#7806=AXIS2_PLACEMENT_3D ( 'NONE', #6081, #4008, #9176 ) ;
#7807=VERTEX_POINT ( 'NONE', #8800 ) ;
#7808=DIRECTION ( 'NONE',  ( 0.000000000000000000, 0.000000000000000000, 1.000000000000000000 ) ) ;
#7811=DIRECTION ( 'NONE',  ( 0.000000000000000000, 0.000000000000000000, 1.000000000000000000 ) ) ;
#7813=DIRECTION ( 'NONE',  ( -1.000000000000000000, 0.000000000000000000, 0.000000000000000000 ) ) ;
#7816=CIRCLE ( 'NONE', #3166, 6.450000000000019718 ) ;
#7818=ADVANCED_FACE ( 'NONE', ( #5646 ), #11282, .F. ) ;
#7822=EDGE_CURVE ( 'NONE', #1952, #7434, #416, .T. ) ;
#7824=ORIENTED_EDGE ( 'NONE', *, *, #6290, .F. ) ;
#7826=CARTESIAN_POINT ( 'NONE',  ( -16.52469481223740644, 30.30953598072262167, 61.33979638101006060 ) ) ;
#7827=VECTOR ( 'NONE', #13519, 1000.000000000000000 ) ;
#7828=AXIS2_PLACEMENT_3D ( 'NONE', #8474, #2213, #9601 ) ;
#7831=VERTEX_POINT ( 'NONE', #1820 ) ;
#7832=ORIENTED_EDGE ( 'NONE', *, *, #9388, .T. ) ;
#7834=CARTESIAN_POINT ( 'NONE',  ( -7.241070169793070832, 29.81324547859995278, 5.250000000000000000 ) ) ;
#7836=CARTESIAN_POINT ( 'NONE',  ( -14.42040990200814043, 6.848677238728379635, 30.59999999999999787 ) ) ;
#7837=CARTESIAN_POINT ( 'NONE',  ( -18.05918829504999934, 10.97290950744599947, 56.84999999999999432 ) ) ;
#7838=CARTESIAN_POINT ( 'NONE',  ( -19.51818023821623882, 27.03346355975680737, 56.97665238683753586 ) ) ;
#7839=EDGE_CURVE ( 'NONE', #5283, #6, #5459, .T. ) ;
#7842=ORIENTED_EDGE ( 'NONE', *, *, #2274, .F. ) ;
#7843=EDGE_CURVE ( 'NONE', #9433, #5595, #2037, .T. ) ;
#7844=VERTEX_POINT ( 'NONE', #4058 ) ;
#7846=AXIS2_PLACEMENT_3D ( 'NONE', #3963, #11299, #1805 ) ;
#7849=DIRECTION ( 'NONE',  ( -0.3202092937642124215, -0.6304490528084107925, -0.7071067811865487940 ) ) ;
#7850=CARTESIAN_POINT ( 'NONE',  ( -21.86795241036432813, 30.04605120275055796, 57.88020891191813888 ) ) ;
#7856=ORIENTED_EDGE ( 'NONE', *, *, #3636, .T. ) ;
#7859=ORIENTED_EDGE ( 'NONE', *, *, #13245, .T. ) ;
#7860=CARTESIAN_POINT ( 'NONE',  ( -16.20671929495594910, 8.873300352462479168, 23.90000000000000213 ) ) ;
#7862=DIRECTION ( 'NONE',  ( 1.000000000000000000, 0.000000000000000000, 0.000000000000000000 ) ) ;
#7867=LINE ( 'NONE', #1591, #2722 ) ;
#7868=DIRECTION ( 'NONE',  ( 0.6615960714621574867, -0.7498604124941119498, 0.000000000000000000 ) ) ;
#7872=DIRECTION ( 'NONE',  ( -1.000000000000000000, 0.000000000000000000, 0.000000000000000000 ) ) ;
#7876=ORIENTED_EDGE ( 'NONE', *, *, #2235, .F. ) ;
#7877=VERTEX_POINT ( 'NONE', #12364 ) ;
#7878=CARTESIAN_POINT ( 'NONE',  ( -39.30918829504999934, -6.027090492554000534, 64.85000000000000853 ) ) ;
#7879=EDGE_CURVE ( 'NONE', #8989, #3167, #2811, .T. ) ;
#7882=ORIENTED_EDGE ( 'NONE', *, *, #2795, .T. ) ;
#7883=CARTESIAN_POINT ( 'NONE',  ( -16.55918829504999579, 27.40458623260099813, 57.35000000000000142 ) ) ;
#7884=DIRECTION ( 'NONE',  ( 1.000000000000000000, 0.000000000000000000, 0.000000000000000000 ) ) ;
#7885=DIRECTION ( 'NONE',  ( 0.000000000000000000, 0.000000000000000000, 1.000000000000000000 ) ) ;
#7887=ADVANCED_FACE ( 'NONE', ( #7035 ), #10172, .T. ) ;
#7890=PRODUCT_DEFINITION ( 'UNKNOWN', '', #5987, #9217 ) ;
#7891=CARTESIAN_POINT ( 'NONE',  ( -39.30918829504999934, -6.027090492554000534, 64.35000000000000853 ) ) ;
#7892=ORIENTED_EDGE ( 'NONE', *, *, #11434, .T. ) ;
#7894=CARTESIAN_POINT ( 'NONE',  ( -18.05918829504999934, 30.36027202460864771, 61.70913974837019822 ) ) ;
#7895=EDGE_LOOP ( 'NONE', ( #491, #6724, #1601, #569 ) ) ;
#7896=ADVANCED_FACE ( 'NONE', ( #11379 ), #13472, .F. ) ;
#7897=ORIENTED_EDGE ( 'NONE', *, *, #1091, .T. ) ;
#7900=CARTESIAN_POINT ( 'NONE',  ( -1.059188295049996231, 27.97290950744599769, 58.85000000000000142 ) ) ;
#7901=ORIENTED_EDGE ( 'NONE', *, *, #3997, .F. ) ;
#7903=FACE_OUTER_BOUND ( 'NONE', #4932, .T. ) ;
#7904=DIRECTION ( 'NONE',  ( 0.000000000000000000, 0.000000000000000000, -1.000000000000000000 ) ) ;
#7905=CARTESIAN_POINT ( 'NONE',  ( -18.05918829504999934, 10.97290950744599947, 60.04999999999999716 ) ) ;
#7906=DIRECTION ( 'NONE',  ( 1.000000000000000000, 0.000000000000000000, 0.000000000000000000 ) ) ;
#7909=VERTEX_POINT ( 'NONE', #11513 ) ;
#7911=ORIENTED_EDGE ( 'NONE', *, *, #6323, .T. ) ;
#7913=CARTESIAN_POINT ( 'NONE',  ( -41.50918829505000218, 27.97290950744599769, 83.57661607529820458 ) ) ;
#7915=CIRCLE ( 'NONE', #1912, 4.749999999999997335 ) ;
#7916=CARTESIAN_POINT ( 'NONE',  ( -21.22921039045582958, 30.14298388890195568, 54.91443165197912180 ) ) ;
#7918=FACE_OUTER_BOUND ( 'NONE', #874, .T. ) ;
#7919=CARTESIAN_POINT ( 'NONE',  ( -9.562604962050000879, 19.46949284044600148, 60.04999999999999716 ) ) ;
#7920=EDGE_CURVE ( 'NONE', #13003, #2432, #10272, .T. ) ;
#7921=CARTESIAN_POINT ( 'NONE',  ( -21.05918829504999934, 10.97290950744599947, 116.8499999999999943 ) ) ;
#7925=AXIS2_PLACEMENT_3D ( 'NONE', #534, #9051, #7927 ) ;
#7927=DIRECTION ( 'NONE',  ( 1.000000000000000000, 0.000000000000000000, 0.000000000000000000 ) ) ;
#7929=VERTEX_POINT ( 'NONE', #6191 ) ;
#7930=CARTESIAN_POINT ( 'NONE',  ( -22.58763155544259860, 2.057013498776719906, 62.85000000000000142 ) ) ;
#7931=LINE ( 'NONE', #1589, #9314 ) ;
#7938=DIRECTION ( 'NONE',  ( 0.000000000000000000, 0.000000000000000000, 1.000000000000000000 ) ) ;
#7940=EDGE_CURVE ( 'NONE', #11264, #1821, #7030, .T. ) ;
#7943=UNCERTAINTY_MEASURE_WITH_UNIT (LENGTH_MEASURE( 1.000000000000000082E-05 ), #9239, 'distance_accuracy_value', 'NONE');
#7951=DIRECTION ( 'NONE',  ( 0.000000000000000000, 1.000000000000000000, 0.000000000000000000 ) ) ;
#7953=CARTESIAN_POINT ( 'NONE',  ( -34.21925492805003444, 2.892876190445991202, 63.34900083300006202 ) ) ;
#7954=CYLINDRICAL_SURFACE ( 'NONE', #888, 12.00000000000000355 ) ;
#7956=CARTESIAN_POINT ( 'NONE',  ( -24.37001676333060018, -4.028726038184999858, 62.14999999999999858 ) ) ;
#7957=EDGE_CURVE ( 'NONE', #12322, #10219, #6061, .T. ) ;
#7960=DIRECTION ( 'NONE',  ( 0.000000000000000000, 1.000000000000000000, 0.000000000000000000 ) ) ;
#7961=VECTOR ( 'NONE', #5474, 999.9999999999998863 ) ;
#7964=CIRCLE ( 'NONE', #1968, 6.749999999999999112 ) ;
#7968=CARTESIAN_POINT ( 'NONE',  ( -18.05918829504999934, 3.352862570446000223, 61.63595870800000398 ) ) ;
#7970=DIRECTION ( 'NONE',  ( 0.000000000000000000, -1.000000000000000000, 0.000000000000000000 ) ) ;
#7971=ORIENTED_EDGE ( 'NONE', *, *, #12998, .T. ) ;
#7972=CARTESIAN_POINT ( 'NONE',  ( -18.05918829505001000, 19.19006679501500656, 63.35000000030875356 ) ) ;
#7973=CARTESIAN_POINT ( 'NONE',  ( -5.809188295050001116, -6.027090492554000534, 7.250000000000000000 ) ) ;
#7974=DIRECTION ( 'NONE',  ( 0.000000000000000000, 0.000000000000000000, -1.000000000000000000 ) ) ;
#7976=DIRECTION ( 'NONE',  ( -1.000000000000000000, 0.000000000000000000, 0.000000000000000000 ) ) ;
#7977=AXIS2_PLACEMENT_3D ( 'NONE', #4026, #7148, #7074 ) ;
#7978=ORIENTED_EDGE ( 'NONE', *, *, #4766, .T. ) ;
#7980=EDGE_CURVE ( 'NONE', #11868, #4563, #12893, .T. ) ;
#7982=ORIENTED_EDGE ( 'NONE', *, *, #12434, .T. ) ;
#7983=DIRECTION ( 'NONE',  ( 1.000000000000000000, 0.000000000000000000, 0.000000000000000000 ) ) ;
#7986=CIRCLE ( 'NONE', #1522, 8.250000000000001776 ) ;
#7987=CIRCLE ( 'NONE', #3984, 24.92993838181874722 ) ;
#7989=AXIS2_PLACEMENT_3D ( 'NONE', #9308, #709, #9244 ) ;
#7990=CARTESIAN_POINT ( 'NONE',  ( -21.37927600327723354, 30.12180271171412826, 59.51279792984109207 ) ) ;
#7991=ORIENTED_EDGE ( 'NONE', *, *, #5201, .T. ) ;
#7999=AXIS2_PLACEMENT_3D ( 'NONE', #889, #3016, #8223 ) ;
#8000=CIRCLE ( 'NONE', #11134, 6.145833333000000565 ) ;
#8002=VECTOR ( 'NONE', #2804, 1000.000000000000000 ) ;
#8003=EDGE_CURVE ( 'NONE', #9556, #722, #10832, .T. ) ;
#8004=DIRECTION ( 'NONE',  ( 0.000000000000000000, 0.000000000000000000, -1.000000000000000000 ) ) ;
#8005=DIRECTION ( 'NONE',  ( 0.000000000000000000, 0.000000000000000000, -1.000000000000000000 ) ) ;
#8006=ORIENTED_EDGE ( 'NONE', *, *, #7691, .T. ) ;
#8007=CARTESIAN_POINT ( 'NONE',  ( -18.05918829504999934, 10.97290950744599947, 60.40999999999999659 ) ) ;
#8011=CARTESIAN_POINT ( 'NONE',  ( -22.66538754097585340, 13.57680303481476614, 68.55875404394534200 ) ) ;
#8016=AXIS2_PLACEMENT_3D ( 'NONE', #13633, #2911, #4143 ) ;
#8017=CARTESIAN_POINT ( 'NONE',  ( -18.05918829504999934, 10.97290950744599947, 62.14999999999999858 ) ) ;
#8018=EDGE_CURVE ( 'NONE', #1491, #3000, #12701, .T. ) ;
#8020=EDGE_CURVE ( 'NONE', #1848, #1852, #3149, .T. ) ;
#8022=FACE_OUTER_BOUND ( 'NONE', #12127, .T. ) ;
#8023=AXIS2_PLACEMENT_3D ( 'NONE', #12133, #2648, #9963 ) ;
#8024=EDGE_LOOP ( 'NONE', ( #12844, #7414, #1335, #7054 ) ) ;
#8027=CARTESIAN_POINT ( 'NONE',  ( -38.38077571930826082, 22.44393519180575680, 17.25000000000000000 ) ) ;
#8028=CARTESIAN_POINT ( 'NONE',  ( -18.05918829504999934, 10.97290950744599947, 67.84999999999999432 ) ) ;
#8029=FACE_OUTER_BOUND ( 'NONE', #7630, .T. ) ;
#8030=CARTESIAN_POINT ( 'NONE',  ( -35.05918829505000645, -6.027090492554000534, 17.25000000000000000 ) ) ;
#8031=DIRECTION ( 'NONE',  ( 1.000000000000000000, 0.000000000000000000, 0.000000000000000000 ) ) ;
#8033=CIRCLE ( 'NONE', #4040, 15.45000000000000462 ) ;
#8034=VECTOR ( 'NONE', #8438, 1000.000000000000000 ) ;
#8035=CIRCLE ( 'NONE', #12714, 4.750000000000000000 ) ;
#8036=ORIENTED_EDGE ( 'NONE', *, *, #2614, .F. ) ;
#8037=FACE_OUTER_BOUND ( 'NONE', #6422, .T. ) ;
#8039=CARTESIAN_POINT ( 'NONE',  ( -20.70557258089865016, 13.97235115742243927, 30.59999999999999787 ) ) ;
#8045=CARTESIAN_POINT ( 'NONE',  ( -18.05918829504999934, 18.13068114044600065, 61.70038048199999281 ) ) ;
#8051=DIRECTION ( 'NONE',  ( 1.000000000000000000, 0.000000000000000000, 0.000000000000000000 ) ) ;
#8052=CARTESIAN_POINT ( 'NONE',  ( -35.05918829505000645, 27.97290950744599769, 64.85000000000000853 ) ) ;
#8054=AXIS2_PLACEMENT_3D ( 'NONE', #10787, #1064, #3390 ) ;
#8055=APPLICATION_CONTEXT ( 'automotive_design' ) ;
#8057=VERTEX_POINT ( 'NONE', #1095 ) ;
#8059=ORIENTED_EDGE ( 'NONE', *, *, #4200, .T. ) ;
#8061=EDGE_CURVE ( 'NONE', #6439, #12897, #12771, .T. ) ;
#8062=ORIENTED_EDGE ( 'NONE', *, *, #4200, .F. ) ;
#8064=CARTESIAN_POINT ( 'NONE',  ( -25.29804148384604900, -2.574630058508220021, 62.14999999999999858 ) ) ;
#8065=EDGE_LOOP ( 'NONE', ( #11396, #13038, #1378, #10043, #11584 ) ) ;
#8066=CARTESIAN_POINT ( 'NONE',  ( -20.84781795900099155, 30.19228463275523566, 60.32764583509811018 ) ) ;
#8067=AXIS2_PLACEMENT_3D ( 'NONE', #10753, #10610, #1171 ) ;
#8069=CARTESIAN_POINT ( 'NONE',  ( -18.05918829504999934, 10.97290950744599947, 63.14999999999999858 ) ) ;
#8073=DIRECTION ( 'NONE',  ( 1.000000000000000000, 0.000000000000000000, 0.000000000000000000 ) ) ;
#8075=EDGE_LOOP ( 'NONE', ( #13702, #7676 ) ) ;
#8076=VECTOR ( 'NONE', #10262, 1000.000000000000114 ) ;
#8078=ORIENTED_EDGE ( 'NONE', *, *, #7081, .F. ) ;
#8080=CARTESIAN_POINT ( 'NONE',  ( -34.72201093190195564, 10.97290950744599947, 5.250000000000000000 ) ) ;
#8081=EDGE_CURVE ( 'NONE', #9242, #3266, #13734, .T. ) ;
#8082=DIRECTION ( 'NONE',  ( 0.000000000000000000, 0.000000000000000000, 1.000000000000000000 ) ) ;
#8086=DIRECTION ( 'NONE',  ( 0.4678190685372686231, -0.5302313826179265721, 0.7071067811865505703 ) ) ;
#8089=LINE ( 'NONE', #11163, #5354 ) ;
#8090=CIRCLE ( 'NONE', #3425, 16.75000000000000355 ) ;
#8092=LINE ( 'NONE', #752, #192 ) ;
#8094=UNCERTAINTY_MEASURE_WITH_UNIT (LENGTH_MEASURE( 1.000000000000000082E-05 ), #538, 'distance_accuracy_value', 'NONE');
#8101=ORIENTED_EDGE ( 'NONE', *, *, #4075, .F. ) ;
#8102=EDGE_CURVE ( 'NONE', #3976, #12622, #10376, .T. ) ;
#8106=EDGE_CURVE ( 'NONE', #4562, #10360, #7915, .T. ) ;
#8107=FACE_OUTER_BOUND ( 'NONE', #12509, .T. ) ;
#8108=CYLINDRICAL_SURFACE ( 'NONE', #11149, 4.250000000000000000 ) ;
#8113=ORIENTED_EDGE ( 'NONE', *, *, #11055, .F. ) ;
#8114=CARTESIAN_POINT ( 'NONE',  ( -15.86143927199362302, 30.25607652234101863, 60.91235729977573499 ) ) ;
#8115=ORIENTED_EDGE ( 'NONE', *, *, #10330, .F. ) ;
#8117=DIRECTION ( 'NONE',  ( 0.000000000000000000, 0.000000000000000000, -1.000000000000000000 ) ) ;
#8118=FACE_OUTER_BOUND ( 'NONE', #11867, .T. ) ;
#8123=PLANE ( 'NONE',  #7806 ) ;
#8125=CYLINDRICAL_SURFACE ( 'NONE', #6898, 4.749999999999997335 ) ;
#8127=CYLINDRICAL_SURFACE ( 'NONE', #9393, 2.700000000000001066 ) ;
#8128=ORIENTED_EDGE ( 'NONE', *, *, #3997, .T. ) ;
#8131=CARTESIAN_POINT ( 'NONE',  ( -19.87176177124059251, 30.28946906204819101, 61.18505942812437581 ) ) ;
#8138=EDGE_LOOP ( 'NONE', ( #9728, #1682, #5172, #12894 ) ) ;
#8140=EDGE_CURVE ( 'NONE', #12773, #803, #6590, .T. ) ;
#8142=DIRECTION ( 'NONE',  ( 0.000000000000000000, 0.000000000000000000, -1.000000000000000000 ) ) ;
#8143=ORIENTED_EDGE ( 'NONE', *, *, #1679, .T. ) ;
#8146=FACE_OUTER_BOUND ( 'NONE', #3084, .T. ) ;
#8148=ORIENTED_EDGE ( 'NONE', *, *, #1439, .F. ) ;
#8149=FACE_OUTER_BOUND ( 'NONE', #11431, .T. ) ;
#8154=AXIS2_PLACEMENT_3D ( 'NONE', #12240, #4831, #2696 ) ;
#8155=VECTOR ( 'NONE', #6477, 1000.000000000000227 ) ;
#8157=EDGE_CURVE ( 'NONE', #4997, #6, #270, .T. ) ;
#8158=VERTEX_POINT ( 'NONE', #9973 ) ;
#8159=EDGE_CURVE ( 'NONE', #2432, #10425, #1442, .T. ) ;
#8163=CARTESIAN_POINT ( 'NONE',  ( -21.09568578533284011, 14.96173881432403086, 68.84049927876318975 ) ) ;
#8166=FACE_OUTER_BOUND ( 'NONE', #5644, .T. ) ;
#8171=DIRECTION ( 'NONE',  ( 0.4528443260392608916, 0.8915896008669279560, 0.000000000000000000 ) ) ;
#8174=CARTESIAN_POINT ( 'NONE',  ( -14.86617432291880370, 30.13979931665073408, 59.74664482119747078 ) ) ;
#8176=ADVANCED_FACE ( 'NONE', ( #9849 ), #7712, .T. ) ;
#8177=FILL_AREA_STYLE_COLOUR ( '', #3027 ) ;
#8178=CARTESIAN_POINT ( 'NONE',  ( -16.07440008066354764, 8.723328269963658954, 27.09999999999999787 ) ) ;
#8179=ORIENTED_EDGE ( 'NONE', *, *, #3860, .T. ) ;
#8184=CARTESIAN_POINT ( 'NONE',  ( -11.70083760351054103, 35.47811937223634970, 17.25000000000000000 ) ) ;
#8186=CARTESIAN_POINT ( 'NONE',  ( -19.26019363180991206, 27.93101569915827653, 58.27028413769223647 ) ) ;
#8187=DIRECTION ( 'NONE',  ( 0.7071067811865505703, 0.000000000000000000, 0.7071067811865444641 ) ) ;
#8192=ORIENTED_EDGE ( 'NONE', *, *, #6328, .F. ) ;
#8193=EDGE_LOOP ( 'NONE', ( #7859, #11196, #9634, #7678 ) ) ;
#8194=EDGE_CURVE ( 'NONE', #2353, #5798, #5703, .T. ) ;
#8196=CARTESIAN_POINT ( 'NONE',  ( -19.10156701222420850, 30.33693478205813676, 61.54316241360875495 ) ) ;
#8198=CYLINDRICAL_SURFACE ( 'NONE', #1853, 6.145833333000002341 ) ;
#8199=VECTOR ( 'NONE', #12353, 1000.000000000000000 ) ;
#8205=VERTEX_POINT ( 'NONE', #12201 ) ;
#8207=CIRCLE ( 'NONE', #3095, 6.449999999999997513 ) ;
#8210=CIRCLE ( 'NONE', #9555, 8.300000000000000711 ) ;
#8214=FACE_OUTER_BOUND ( 'NONE', #13605, .T. ) ;
#8215=CARTESIAN_POINT ( 'NONE',  ( -8.500289910546818817, -3.085093966544980137, 62.14999999999999858 ) ) ;
#8216=CARTESIAN_POINT ( 'NONE',  ( -18.05918829504999934, 10.97290950744599947, 57.35000000000000142 ) ) ;
#8220=EDGE_CURVE ( 'NONE', #4278, #7243, #4605, .T. ) ;
#8223=DIRECTION ( 'NONE',  ( 1.000000000000000000, 0.000000000000000000, 0.000000000000000000 ) ) ;
#8224=VECTOR ( 'NONE', #485, 1000.000000000000000 ) ;
#8225=VERTEX_POINT ( 'NONE', #2727 ) ;
#8226=AXIS2_PLACEMENT_3D ( 'NONE', #13147, #11267, #1691 ) ;
#8228=CIRCLE ( 'NONE', #180, 18.00000000000000000 ) ;
#8229=ORIENTED_EDGE ( 'NONE', *, *, #8478, .T. ) ;
#8230=CARTESIAN_POINT ( 'NONE',  ( -18.05918829504999934, 10.97290950744599947, 58.35000000000000142 ) ) ;
#8236=AXIS2_PLACEMENT_3D ( 'NONE', #3410, #10874, #1294 ) ;
#8237=CARTESIAN_POINT ( 'NONE',  ( -39.80918829504999934, 27.97290950744599769, 68.85549045786049760 ) ) ;
#8239=CARTESIAN_POINT ( 'NONE',  ( -18.05918829504999934, 10.00028003023991907, 62.14999999999999858 ) ) ;
#8242=DIRECTION ( 'NONE',  ( 0.000000000000000000, 1.000000000000000000, 0.000000000000000000 ) ) ;
#8245=AXIS2_PLACEMENT_3D ( 'NONE', #12965, #12765, #12889 ) ;
#8247=CARTESIAN_POINT ( 'NONE',  ( -15.15614148912509229, 30.17819129753064544, 54.51704934337099218 ) ) ;
#8248=ORIENTED_EDGE ( 'NONE', *, *, #9722, .F. ) ;
#8249=ORIENTED_EDGE ( 'NONE', *, *, #504, .T. ) ;
#8250=DIRECTION ( 'NONE',  ( 0.000000000000000000, 0.000000000000000000, -1.000000000000000000 ) ) ;
#8251=LINE ( 'NONE', #12723, #9914 ) ;
#8253=ORIENTED_EDGE ( 'NONE', *, *, #5080, .F. ) ;
#8254=CARTESIAN_POINT ( 'NONE',  ( -18.05918829504999934, 10.97290950744599947, 61.10999999999999943 ) ) ;
#8255=CARTESIAN_POINT ( 'NONE',  ( -14.32322260522609980, 18.32852371459815188, 60.04999999999999716 ) ) ;
#8256=EDGE_CURVE ( 'NONE', #651, #912, #5631, .T. ) ;
#8258=DIRECTION ( 'NONE',  ( 1.000000000000000000, 0.000000000000000000, 0.000000000000000000 ) ) ;
#8261=AXIS2_PLACEMENT_3D ( 'NONE', #2429, #5669, #7623 ) ;
#8263=CARTESIAN_POINT ( 'NONE',  ( -38.63164489498320364, 10.97290950744599947, 7.250000000000000000 ) ) ;
#8267=AXIS2_PLACEMENT_3D ( 'NONE', #12330, #6087, #12453 ) ;
#8268=CIRCLE ( 'NONE', #2039, 6.850000000000002309 ) ;
#8269=ORIENTED_EDGE ( 'NONE', *, *, #12712, .T. ) ;
#8270=ORIENTED_EDGE ( 'NONE', *, *, #1051, .F. ) ;
#8271=ORIENTED_EDGE ( 'NONE', *, *, #5655, .T. ) ;
#8272=CARTESIAN_POINT ( 'NONE',  ( -2.059188295050000228, 10.97290950744599947, 56.84999999999999432 ) ) ;
#8275=CARTESIAN_POINT ( 'NONE',  ( -9.861988295050000630, 2.775709507445999868, 63.35000000000000142 ) ) ;
#8276=DIRECTION ( 'NONE',  ( 0.000000000000000000, 1.000000000000000000, 0.000000000000000000 ) ) ;
#8277=CYLINDRICAL_SURFACE ( 'NONE', #10983, 4.750000000000000888 ) ;
#8279=AXIS2_PLACEMENT_3D ( 'NONE', #4516, #6668, #7699 ) ;
#8283=CIRCLE ( 'NONE', #5815, 6.450000000000001066 ) ;
#8284=VERTEX_POINT ( 'NONE', #10183 ) ;
#8285=EDGE_CURVE ( 'NONE', #6318, #11722, #11509, .T. ) ;
#8287=DIRECTION ( 'NONE',  ( 0.000000000000000000, 0.000000000000000000, -1.000000000000000000 ) ) ;
#8288=CIRCLE ( 'NONE', #3617, 4.000000000000000888 ) ;
#8291=EDGE_LOOP ( 'NONE', ( #735, #97, #1408, #8192 ) ) ;
#8292=DIRECTION ( 'NONE',  ( 0.4528443260392610026, 0.8915896008669278450, 0.000000000000000000 ) ) ;
#8293=CARTESIAN_POINT ( 'NONE',  ( -30.30918829504999934, 27.97290950744599769, 64.85000000000000853 ) ) ;
#8294=CARTESIAN_POINT ( 'NONE',  ( -18.05918829504999934, 10.97290950744599947, 62.14999999999999858 ) ) ;
#8295=DIRECTION ( 'NONE',  ( 0.000000000000000000, 0.000000000000000000, 1.000000000000000000 ) ) ;
#8298=DIRECTION ( 'NONE',  ( 0.000000000000000000, 0.000000000000000000, -1.000000000000000000 ) ) ;
#8299=DIRECTION ( 'NONE',  ( 0.000000000000000000, 0.000000000000000000, 1.000000000000000000 ) ) ;
#8300=FACE_BOUND ( 'NONE', #3667, .T. ) ;
#8301=EDGE_CURVE ( 'NONE', #4997, #12239, #5028, .T. ) ;
#8302=VERTEX_POINT ( 'NONE', #5135 ) ;
#8303=VERTEX_POINT ( 'NONE', #4034 ) ;
#8305=ORIENTED_EDGE ( 'NONE', *, *, #7619, .T. ) ;
#8309=LINE ( 'NONE', #9436, #6035 ) ;
#8311=LINE ( 'NONE', #13479, #12015 ) ;
#8312=LINE ( 'NONE', #7310, #5512 ) ;
#8316=EDGE_CURVE ( 'NONE', #1491, #10398, #9333, .T. ) ;
#8317=CARTESIAN_POINT ( 'NONE',  ( -15.08247214573220241, 30.16892808493238221, 60.08567788817938293 ) ) ;
#8318=VERTEX_POINT ( 'NONE', #9127 ) ;
#8319=EDGE_CURVE ( 'NONE', #9069, #13237, #11429, .T. ) ;
#8320=ORIENTED_EDGE ( 'NONE', *, *, #9599, .F. ) ;
#8321=EDGE_LOOP ( 'NONE', ( #12170, #6037, #2688, #5317 ) ) ;
#8322=DIRECTION ( 'NONE',  ( 1.000000000000000000, 0.000000000000000000, 0.000000000000000000 ) ) ;
#8324=CYLINDRICAL_SURFACE ( 'NONE', #1354, 2.700000000000000178 ) ;
#8326=CARTESIAN_POINT ( 'NONE',  ( -14.75120793773922045, 7.223607444975439940, 68.84999999999999432 ) ) ;
#8328=ORIENTED_EDGE ( 'NONE', *, *, #2235, .T. ) ;
#8329=DIRECTION ( 'NONE',  ( 1.000000000000000000, 0.000000000000000000, 0.000000000000000000 ) ) ;
#8330=AXIS2_PLACEMENT_3D ( 'NONE', #7130, #6015, #4979 ) ;
#8331=CYLINDRICAL_SURFACE ( 'NONE', #3655, 16.00000000000000355 ) ;
#8333=DIRECTION ( 'NONE',  ( 0.000000000000000000, 0.000000000000000000, -1.000000000000000000 ) ) ;
#8335=EDGE_CURVE ( 'NONE', #1822, #95, #12180, .T. ) ;
#8337=EDGE_LOOP ( 'NONE', ( #9448, #1336, #8128, #1193 ) ) ;
#8340=ORIENTED_EDGE ( 'NONE', *, *, #11252, .F. ) ;
#8341=VERTEX_POINT ( 'NONE', #2859 ) ;
#8343=CARTESIAN_POINT ( 'NONE',  ( -20.46575897078212947, 30.23534695989346233, 60.73312205491463089 ) ) ;
#8345=PLANE ( 'NONE',  #2651 ) ;
#8346=DIRECTION ( 'NONE',  ( 0.000000000000000000, -1.000000000000000000, 0.000000000000000000 ) ) ;
#8350=EDGE_CURVE ( 'NONE', #1667, #1818, #2394, .T. ) ;
#8351=DIRECTION ( 'NONE',  ( 0.000000000000000000, 0.000000000000000000, -1.000000000000000000 ) ) ;
#8352=ORIENTED_EDGE ( 'NONE', *, *, #10678, .T. ) ;
#8353=VERTEX_POINT ( 'NONE', #4935 ) ;
#8356=EDGE_CURVE ( 'NONE', #2296, #5219, #9202, .T. ) ;
#8357=DIRECTION ( 'NONE',  ( -0.4528443260392609471, -0.8915896008669278450, 0.000000000000000000 ) ) ;
#8359=ORIENTED_EDGE ( 'NONE', *, *, #5707, .F. ) ;
#8361=DIRECTION ( 'NONE',  ( 0.4528443260392607250, 0.8915896008669278450, 0.000000000000000000 ) ) ;
#8363=CARTESIAN_POINT ( 'NONE',  ( -36.21615338608749823, 23.36596564213564875, 7.250000000000000000 ) ) ;
#8364=( NAMED_UNIT ( * ) PLANE_ANGLE_UNIT ( ) SI_UNIT ( $, .RADIAN. ) );
#8365=EDGE_CURVE ( 'NONE', #6548, #10843, #11227, .T. ) ;
#8366=EDGE_LOOP ( 'NONE', ( #9373, #13567, #4074, #9440 ) ) ;
#8367=AXIS2_PLACEMENT_3D ( 'NONE', #7956, #2822, #9159 ) ;
#8368=ORIENTED_EDGE ( 'NONE', *, *, #1969, .F. ) ;
#8370=VERTEX_POINT ( 'NONE', #5063 ) ;
#8373=CARTESIAN_POINT ( 'NONE',  ( -20.08141632792401765, 15.85662095137910299, 68.56416753914237461 ) ) ;
#8374=EDGE_LOOP ( 'NONE', ( #6924, #4721, #6865, #717 ) ) ;
#8376=CARTESIAN_POINT ( 'NONE',  ( -35.05918829505000645, 27.97290950744599769, 17.25000000000000000 ) ) ;
#8378=VECTOR ( 'NONE', #4123, 1000.000000000000000 ) ;
#8381=ORIENTED_EDGE ( 'NONE', *, *, #1133, .F. ) ;
#8383=CARTESIAN_POINT ( 'NONE',  ( -14.88916620013386272, 30.14298388896176917, 59.78556834882314064 ) ) ;
#8386=EDGE_LOOP ( 'NONE', ( #11416, #2417, #5786, #8270 ) ) ;
#8387=ORIENTED_EDGE ( 'NONE', *, *, #13512, .T. ) ;
#8389=CARTESIAN_POINT ( 'NONE',  ( -19.71317847370539766, 12.84756053868127879, 53.85000000000000142 ) ) ;
#8392=DIRECTION ( 'NONE',  ( 0.000000000000000000, 0.000000000000000000, -1.000000000000000000 ) ) ;
#8393=DIRECTION ( 'NONE',  ( -0.4528443260392611136, -0.8915896008669277339, 0.000000000000000000 ) ) ;
#8394=CARTESIAN_POINT ( 'NONE',  ( -18.81733386491350046, 27.95698799050449423, 58.65942797322944813 ) ) ;
#8396=AXIS2_PLACEMENT_3D ( 'NONE', #2403, #12840, #4280 ) ;
#8397=FACE_OUTER_BOUND ( 'NONE', #1186, .T. ) ;
#8398=VERTEX_POINT ( 'NONE', #2796 ) ;
#8401=CONICAL_SURFACE ( 'NONE', #5719, 6.419999999999999929, 0.2165503049760889864 ) ;
#8405=CARTESIAN_POINT ( 'NONE',  ( -18.62921962108772789, 26.96311099516080034, 55.95402353264894657 ) ) ;
#8406=CARTESIAN_POINT ( 'NONE',  ( -15.05918829504999756, 10.97290950744599947, 116.8499999999999943 ) ) ;
#8409=DIRECTION ( 'NONE',  ( 0.000000000000000000, 0.000000000000000000, -1.000000000000000000 ) ) ;
#8416=AXIS2_PLACEMENT_3D ( 'NONE', #2788, #10246, #13505 ) ;
#8422=DIRECTION ( 'NONE',  ( -1.000000000000000000, 0.000000000000000000, 0.000000000000000000 ) ) ;
#8423=DIRECTION ( 'NONE',  ( 0.000000000000000000, 0.000000000000000000, 1.000000000000000000 ) ) ;
#8424=ORIENTED_EDGE ( 'NONE', *, *, #12125, .F. ) ;
#8425=DIRECTION ( 'NONE',  ( 1.000000000000000000, 0.000000000000000000, 0.000000000000000000 ) ) ;
#8426=LINE ( 'NONE', #5413, #7961 ) ;
#8430=AXIS2_PLACEMENT_3D ( 'NONE', #11727, #1102, #12985 ) ;
#8431=VECTOR ( 'NONE', #8468, 1000.000000000000000 ) ;
#8433=EDGE_CURVE ( 'NONE', #8341, #4986, #2085, .T. ) ;
#8435=VERTEX_POINT ( 'NONE', #96 ) ;
#8438=DIRECTION ( 'NONE',  ( -0.3202092937642119774, -0.6304490528084089052, 0.7071067811865507924 ) ) ;
#8440=VECTOR ( 'NONE', #5844, 1000.000000000000000 ) ;
#8443=VECTOR ( 'NONE', #10491, 1000.000000000000114 ) ;
#8444=DIRECTION ( 'NONE',  ( 0.000000000000000000, -1.000000000000000000, 3.387121092260456770E-15 ) ) ;
#8447=AXIS2_PLACEMENT_3D ( 'NONE', #5213, #4451, #9483 ) ;
#8449=AXIS2_PLACEMENT_3D ( 'NONE', #5007, #12483, #10534 ) ;
#8450=CARTESIAN_POINT ( 'NONE',  ( -14.31571447708356537, 30.05678106874812627, 56.42374946802869573 ) ) ;
#8451=ORIENTED_EDGE ( 'NONE', *, *, #8481, .F. ) ;
#8452=CYLINDRICAL_SURFACE ( 'NONE', #1471, 1.725000000000000755 ) ;
#8453=CARTESIAN_POINT ( 'NONE',  ( -12.70965068984842006, 8.255843551210428899, 57.35000000000000142 ) ) ;
#8456=LINE ( 'NONE', #4081, #8443 ) ;
#8457=CARTESIAN_POINT ( 'NONE',  ( -18.05918829504999223, 19.28555359244598932, 63.26601075299999621 ) ) ;
#8458=CYLINDRICAL_SURFACE ( 'NONE', #7576, 33.00000000000000000 ) ;
#8459=CIRCLE ( 'NONE', #6457, 2.700000000000001066 ) ;
#8465=ORIENTED_EDGE ( 'NONE', *, *, #12457, .F. ) ;
#8466=AXIS2_PLACEMENT_3D ( 'NONE', #2728, #6682, #2657 ) ;
#8467=VECTOR ( 'NONE', #5534, 1000.000000000000000 ) ;
#8468=DIRECTION ( 'NONE',  ( 0.000000000000000000, 0.000000000000000000, -1.000000000000000000 ) ) ;
#8470=ORIENTED_EDGE ( 'NONE', *, *, #4901, .F. ) ;
#8471=DIRECTION ( 'NONE',  ( 0.000000000000000000, 0.000000000000000000, -1.000000000000000000 ) ) ;
#8473=DIRECTION ( 'NONE',  ( -0.4528443260392609471, -0.8915896008669278450, 0.000000000000000000 ) ) ;
#8474=CARTESIAN_POINT ( 'NONE',  ( -35.05918829505000645, -6.027090492554000534, 64.85000000000000853 ) ) ;
#8477=AXIS2_PLACEMENT_3D ( 'NONE', #1400, #4617, #3293 ) ;
#8478=EDGE_CURVE ( 'NONE', #9965, #1667, #4372, .T. ) ;
#8481=EDGE_CURVE ( 'NONE', #10025, #12322, #5405, .T. ) ;
#8483=ADVANCED_FACE ( 'NONE', ( #165 ), #1211, .T. ) ;
#8485=VERTEX_POINT ( 'NONE', #12812 ) ;
#8487=EDGE_CURVE ( 'NONE', #13343, #5535, #9609, .T. ) ;
#8488=CARTESIAN_POINT ( 'NONE',  ( -7.241070169793063727, -7.867426463707971607, 5.250000000000000000 ) ) ;
#8490=CARTESIAN_POINT ( 'NONE',  ( -20.17834884677884943, 30.26343021279967616, 53.72583902890555407 ) ) ;
#8491=CIRCLE ( 'NONE', #3606, 33.00000000000000000 ) ;
#8493=CARTESIAN_POINT ( 'NONE',  ( -25.64433075620760150, -3.961216307075045240, 57.35000000000000142 ) ) ;
#8494=DIRECTION ( 'NONE',  ( 0.000000000000000000, 0.000000000000000000, -1.000000000000000000 ) ) ;
#8495=AXIS2_PLACEMENT_3D ( 'NONE', #6183, #10457, #8626 ) ;
#8496=CARTESIAN_POINT ( 'NONE',  ( -38.38077571930826082, -0.4981161769137699147, 5.250000000000000000 ) ) ;
#8497=DIRECTION ( 'NONE',  ( 0.000000000000000000, 0.000000000000000000, -1.000000000000000000 ) ) ;
#8499=ORIENTED_EDGE ( 'NONE', *, *, #12419, .F. ) ;
#8503=ORIENTED_EDGE ( 'NONE', *, *, #12957, .F. ) ;
#8504=CARTESIAN_POINT ( 'NONE',  ( -23.57208814848684852, -7.366404416634599883, 63.45000000000000284 ) ) ;
#8508=CARTESIAN_POINT ( 'NONE',  ( -14.75120793773922045, 7.223607444975439940, 68.84999999999999432 ) ) ;
#8512=DIRECTION ( 'NONE',  ( 0.000000000000000000, 0.000000000000000000, 1.000000000000000000 ) ) ;
#8513=AXIS2_PLACEMENT_3D ( 'NONE', #6066, #5021, #10681 ) ;
#8515=B_SPLINE_CURVE_WITH_KNOTS ( 'NONE', 3,
 ( #12573, #12499, #8163, #11381, #1741, #3083, #12428, #975, #11516, #7176, #9434, #13678, #7301, #4126, #4190, #8373, #10338, #9358, #6127 ),
 .UNSPECIFIED., .F., .F.,
 ( 4, 1, 1, 1, 2, 2, 1, 1, 1, 1, 2, 2, 4 ),
 ( 0.000000000000000000, 0.1249999999999810429, 0.1874999999999726608, 0.2187499999999669154, 0.2343749999999659717, 0.2499999999999650280, 0.3749999999999584777, 0.4374999999999563127, 0.4687499999999562572, 0.4843749999999562572, 0.4921874999999562017, 0.4999999999999562572, 1.000000000000000000 ),
 .UNSPECIFIED. ) ;
#8519=CARTESIAN_POINT ( 'NONE',  ( -15.65261761014314779, 30.23534695896283253, 53.96687795351272854 ) ) ;
#8520=ORIENTED_EDGE ( 'NONE', *, *, #8061, .T. ) ;
#8522=ORIENTED_EDGE ( 'NONE', *, *, #5865, .T. ) ;
#8525=DIRECTION ( 'NONE',  ( 0.000000000000000000, 0.000000000000000000, -1.000000000000000000 ) ) ;
#8526=ORIENTED_EDGE ( 'NONE', *, *, #6916, .F. ) ;
#8527=LINE ( 'NONE', #8661, #6207 ) ;
#8528=DIRECTION ( 'NONE',  ( 1.000000000000000000, 0.000000000000000000, 0.000000000000000000 ) ) ;
#8530=DIRECTION ( 'NONE',  ( 0.2148617826751194892, 0.000000000000000000, -0.9766444667050899753 ) ) ;
#8531=DIRECTION ( 'NONE',  ( 1.000000000000000000, 0.000000000000000000, 0.000000000000000000 ) ) ;
#8532=MECHANICAL_DESIGN_GEOMETRIC_PRESENTATION_REPRESENTATION('',(#11889),#2539);
#8533=ORIENTED_EDGE ( 'NONE', *, *, #9228, .T. ) ;
#8534=CARTESIAN_POINT ( 'NONE',  ( -18.05918829504999934, 10.97290950744599947, 60.60999999999999943 ) ) ;
#8537=VERTEX_POINT ( 'NONE', #8692 ) ;
#8538=CIRCLE ( 'NONE', #1635, 4.749999999999997335 ) ;
#8540=CARTESIAN_POINT ( 'NONE',  ( -12.26420230435512160, 9.417873376788568507, 64.85000000000000853 ) ) ;
#8541=ORIENTED_EDGE ( 'NONE', *, *, #11900, .F. ) ;
#8543=LINE ( 'NONE', #12744, #916 ) ;
#8545=EDGE_CURVE ( 'NONE', #5561, #3266, #5264, .T. ) ;
#8548=CARTESIAN_POINT ( 'NONE',  ( -18.05918829504999934, 10.97290950744599947, 60.40999999999999659 ) ) ;
#8550=CIRCLE ( 'NONE', #531, 34.69999999999999574 ) ;
#8553=CARTESIAN_POINT ( 'NONE',  ( -36.21615338608749823, 23.36596564213564875, 64.85000000000000853 ) ) ;
#8557=ORIENTED_EDGE ( 'NONE', *, *, #4412, .T. ) ;
#8558=LINE ( 'NONE', #2092, #6211 ) ;
#8559=CARTESIAN_POINT ( 'NONE',  ( -18.88016301897669891, 16.91647750172969822, 68.84999999999999432 ) ) ;
#8564=EDGE_CURVE ( 'NONE', #6589, #8284, #2434, .T. ) ;
#8565=ORIENTED_EDGE ( 'NONE', *, *, #8478, .F. ) ;
#8566=ORIENTED_EDGE ( 'NONE', *, *, #5149, .F. ) ;
#8568=ORIENTED_EDGE ( 'NONE', *, *, #3059, .T. ) ;
#8570=CARTESIAN_POINT ( 'NONE',  ( -12.78387628440563084, 8.959369023293000112, 68.21188696640926707 ) ) ;
#8571=DIRECTION ( 'NONE',  ( -1.000000000000000000, 0.000000000000000000, 0.000000000000000000 ) ) ;
#8573=CARTESIAN_POINT ( 'NONE',  ( -16.02867477244678796, 6.096508287340727250, 68.56773819352413568 ) ) ;
#8574=CARTESIAN_POINT ( 'NONE',  ( -6.600216501174549499, -2.179141222803650191, 62.14999999999999858 ) ) ;
#8575=DIRECTION ( 'NONE',  ( 0.000000000000000000, 0.000000000000000000, -1.000000000000000000 ) ) ;
#8576=EDGE_CURVE ( 'NONE', #7594, #10203, #3534, .T. ) ;
#8577=AXIS2_PLACEMENT_3D ( 'NONE', #5863, #9019, #12165 ) ;
#8580=ORIENTED_EDGE ( 'NONE', *, *, #718, .F. ) ;
#8581=CARTESIAN_POINT ( 'NONE',  ( -15.53825790700473064, 30.22311051619552558, 54.07754255955762801 ) ) ;
#8584=DIRECTION ( 'NONE',  ( 0.000000000000000000, 0.000000000000000000, 1.000000000000000000 ) ) ;
#8587=LINE ( 'NONE', #7666, #2743 ) ;
#8590=CARTESIAN_POINT ( 'NONE',  ( -18.05918829504999934, 10.97290950744599947, 61.85000000000000142 ) ) ;
#8592=EDGE_CURVE ( 'NONE', #3590, #2432, #372, .T. ) ;
#8593=FACE_OUTER_BOUND ( 'NONE', #11344, .T. ) ;
#8595=EDGE_LOOP ( 'NONE', ( #4477, #11957, #5279, #7513 ) ) ;
#8596=ORIENTED_EDGE ( 'NONE', *, *, #13245, .F. ) ;
#8602=ORIENTED_EDGE ( 'NONE', *, *, #7839, .T. ) ;
#8607=CIRCLE ( 'NONE', #3712, 17.00000000000000355 ) ;
#8608=CARTESIAN_POINT ( 'NONE',  ( -19.55918829504999934, 21.47290950744600124, 57.35000000000000142 ) ) ;
#8609=CARTESIAN_POINT ( 'NONE',  ( -19.15738950687221731, 26.93589173648236823, 56.32689553783452396 ) ) ;
#8611=DIRECTION ( 'NONE',  ( 0.000000000000000000, 0.000000000000000000, -1.000000000000000000 ) ) ;
#8613=DIRECTION ( 'NONE',  ( 0.000000000000000000, 0.000000000000000000, -1.000000000000000000 ) ) ;
#8615=ORIENTED_EDGE ( 'NONE', *, *, #9571, .T. ) ;
#8616=EDGE_CURVE ( 'NONE', #7294, #8989, #7471, .T. ) ;
#8619=CARTESIAN_POINT ( 'NONE',  ( -25.64433075620760150, -3.961216307075045240, 60.65000000000000568 ) ) ;
#8620=DIRECTION ( 'NONE',  ( -0.9496839325805417342, 0.3132098788326399541, 0.000000000000000000 ) ) ;
#8622=CARTESIAN_POINT ( 'NONE',  ( -20.78383927082655092, 30.19994085430307251, 54.29647360000282674 ) ) ;
#8623=CARTESIAN_POINT ( 'NONE',  ( 3.690811704950004657, 27.97290950744599769, 7.250000000000000000 ) ) ;
#8624=CARTESIAN_POINT ( 'NONE',  ( -3.743645030049981948, 3.815137874445994282, 61.70038048200006386 ) ) ;
#8626=DIRECTION ( 'NONE',  ( -1.000000000000000000, 0.000000000000000000, 0.000000000000000000 ) ) ;
#8630=TOROIDAL_SURFACE ( 'NONE', #12216, 3.000000000000000888, 2.000000000000000000 ) ;
#8631=ORIENTED_EDGE ( 'NONE', *, *, #12200, .T. ) ;
#8632=CARTESIAN_POINT ( 'NONE',  ( -8.964285665223000521, 0.3335619008453594714, 62.14999999999999858 ) ) ;
#8633=ORIENTED_EDGE ( 'NONE', *, *, #143, .T. ) ;
#8634=EDGE_CURVE ( 'NONE', #9938, #10214, #8607, .T. ) ;
#8635=ORIENTED_EDGE ( 'NONE', *, *, #504, .F. ) ;
#8637=FACE_OUTER_BOUND ( 'NONE', #10429, .T. ) ;
#8639=DIRECTION ( 'NONE',  ( -0.4528443260392609471, -0.8915896008669278450, 0.000000000000000000 ) ) ;
#8640=FACE_OUTER_BOUND ( 'NONE', #988, .T. ) ;
#8641=CARTESIAN_POINT ( 'NONE',  ( -21.16117192841894834, 4.865520741507539881, 63.64999999999999858 ) ) ;
#8642=DIRECTION ( 'NONE',  ( 0.000000000000000000, 2.732534507816520408E-15, 1.000000000000000000 ) ) ;
#8643=CARTESIAN_POINT ( 'NONE',  ( -18.05918829504999934, 10.97290950744599947, 64.85000000000000853 ) ) ;
#8644=DIRECTION ( 'NONE',  ( 0.4528443260392610026, 0.8915896008669278450, 0.000000000000000000 ) ) ;
#8645=AXIS2_PLACEMENT_3D ( 'NONE', #6948, #5953, #10175 ) ;
#8647=AXIS2_PLACEMENT_3D ( 'NONE', #11965, #6789, #4777 ) ;
#8648=CARTESIAN_POINT ( 'NONE',  ( -16.24661482249155497, 30.28946906235349346, 53.51494056959690937 ) ) ;
#8649=ORIENTED_EDGE ( 'NONE', *, *, #1847, .F. ) ;
#8651=EDGE_LOOP ( 'NONE', ( #9167, #6739 ) ) ;
#8653=CIRCLE ( 'NONE', #5091, 16.72262947720610171 ) ;
#8654=ADVANCED_FACE ( 'NONE', ( #1283 ), #8827, .T. ) ;
#8655=ORIENTED_EDGE ( 'NONE', *, *, #10756, .F. ) ;
#8656=PLANE ( 'NONE',  #4621 ) ;
#8657=AXIS2_PLACEMENT_3D ( 'NONE', #11548, #11753, #9595 ) ;
#8658=LINE ( 'NONE', #2405, #7566 ) ;
#8659=DIRECTION ( 'NONE',  ( 0.6615960714621574867, -0.7498604124941119498, 0.000000000000000000 ) ) ;
#8660=VERTEX_POINT ( 'NONE', #13163 ) ;
#8661=CARTESIAN_POINT ( 'NONE',  ( -25.33503448090910126, 29.19143287883919768, 7.250000000000000000 ) ) ;
#8662=CARTESIAN_POINT ( 'NONE',  ( -14.42040990200814043, 6.848677238728379635, 30.59999999999999787 ) ) ;
#8665=AXIS2_PLACEMENT_3D ( 'NONE', #6828, #548, #4807 ) ;
#8666=AXIS2_PLACEMENT_3D ( 'NONE', #8952, #3651, #12162 ) ;
#8668=AXIS2_PLACEMENT_3D ( 'NONE', #4141, #8392, #5906 ) ;
#8671=FACE_OUTER_BOUND ( 'NONE', #11189, .T. ) ;
#8672=ORIENTED_EDGE ( 'NONE', *, *, #7603, .T. ) ;
#8674=VERTEX_POINT ( 'NONE', #9825 ) ;
#8678=FACE_OUTER_BOUND ( 'NONE', #4547, .T. ) ;
#8679=EDGE_LOOP ( 'NONE', ( #3511, #12610 ) ) ;
#8682=AXIS2_PLACEMENT_3D ( 'NONE', #4286, #138, #10628 ) ;
#8684=CARTESIAN_POINT ( 'NONE',  ( -34.65718996104999405, 2.673908674445990119, 63.13003331700004850 ) ) ;
#8686=FACE_OUTER_BOUND ( 'NONE', #3810, .T. ) ;
#8688=DIRECTION ( 'NONE',  ( 0.000000000000000000, 0.000000000000000000, 1.000000000000000000 ) ) ;
#8689=AXIS2_PLACEMENT_3D ( 'NONE', #12057, #8988, #6878 ) ;
#8691=EDGE_CURVE ( 'NONE', #8302, #8943, #524, .T. ) ;
#8692=CARTESIAN_POINT ( 'NONE',  ( -5.309188295050000228, -6.027090492554000534, 64.35000000000000853 ) ) ;
#8698=CARTESIAN_POINT ( 'NONE',  ( -1.059188295049996231, 27.97290950744599769, 68.85549045786049760 ) ) ;
#8699=DIRECTION ( 'NONE',  ( 0.000000000000000000, 0.000000000000000000, 1.000000000000000000 ) ) ;
#8701=CARTESIAN_POINT ( 'NONE',  ( -18.05918829504999934, 10.97290950744599947, 68.84999999999999432 ) ) ;
#8702=ADVANCED_FACE ( 'NONE', ( #9894 ), #319, .T. ) ;
#8705=AXIS2_PLACEMENT_3D ( 'NONE', #11228, #6816, #11996 ) ;
#8706=CONICAL_SURFACE ( 'NONE', #9162, 5.000000000000000888, 0.7853981633974497223 ) ;
#8707=VECTOR ( 'NONE', #9738, 1000.000000000000000 ) ;
#8708=VERTEX_POINT ( 'NONE', #12952 ) ;
#8709=ORIENTED_EDGE ( 'NONE', *, *, #2366, .F. ) ;
#8714=CIRCLE ( 'NONE', #1579, 23.22993838181874793 ) ;
#8715=CIRCLE ( 'NONE', #6701, 10.00000000000000178 ) ;
#8717=ORIENTED_EDGE ( 'NONE', *, *, #5418, .T. ) ;
#8722=CARTESIAN_POINT ( 'NONE',  ( -18.05918829504999934, 10.00028003023991907, 63.45000000000000284 ) ) ;
#8723=DIRECTION ( 'NONE',  ( 0.000000000000000000, 0.000000000000000000, 1.000000000000000000 ) ) ;
#8724=ADVANCED_FACE ( 'NONE', ( #8906 ), #11139, .F. ) ;
#8725=LINE ( 'NONE', #11794, #7642 ) ;
#8726=CYLINDRICAL_SURFACE ( 'NONE', #8430, 2.700000000000001066 ) ;
#8731=CARTESIAN_POINT ( 'NONE',  ( -15.29419851136037067, 30.19514031481103089, 54.34376022666191375 ) ) ;
#8732=VERTEX_POINT ( 'NONE', #12261 ) ;
#8733=CYLINDRICAL_SURFACE ( 'NONE', #7059, 6.000000000000000888 ) ;
#8735=CARTESIAN_POINT ( 'NONE',  ( -30.32854245105399826, 27.54455229823479812, 64.85000000000000853 ) ) ;
#8736=CIRCLE ( 'NONE', #10525, 6.345833333000001630 ) ;
#8740=FACE_OUTER_BOUND ( 'NONE', #10807, .T. ) ;
#8741=CARTESIAN_POINT ( 'NONE',  ( -18.05918829504999223, 19.18892026044601096, 63.36264408500002787 ) ) ;
#8742=CARTESIAN_POINT ( 'NONE',  ( -39.30918829504999934, 27.97290950744599769, 64.35000000000000853 ) ) ;
#8743=ADVANCED_FACE ( 'NONE', ( #9374 ), #11602, .T. ) ;
#8744=EDGE_CURVE ( 'NONE', #2573, #8804, #4164, .T. ) ;
#8745=ORIENTED_EDGE ( 'NONE', *, *, #1465, .F. ) ;
#8746=DIRECTION ( 'NONE',  ( 0.000000000000000000, 0.000000000000000000, -1.000000000000000000 ) ) ;
#8749=ORIENTED_EDGE ( 'NONE', *, *, #4794, .F. ) ;
#8750=ADVANCED_BREP_SHAPE_REPRESENTATION ( '', ( #4352, #9410, #4601, #5147, #5212, #229, #13799, #6434 ), #5097 ) ;
#8751=ORIENTED_EDGE ( 'NONE', *, *, #1487, .T. ) ;
#8754=DIRECTION ( 'NONE',  ( 0.000000000000000000, 0.000000000000000000, 1.000000000000000000 ) ) ;
#8755=ORIENTED_EDGE ( 'NONE', *, *, #11243, .F. ) ;
#8757=DIRECTION ( 'NONE',  ( -1.000000000000000000, 0.000000000000000000, 0.000000000000000000 ) ) ;
#8761=EDGE_CURVE ( 'NONE', #4325, #6311, #2973, .T. ) ;
#8766=ORIENTED_EDGE ( 'NONE', *, *, #4918, .F. ) ;
#8768=DIRECTION ( 'NONE',  ( 0.000000000000000000, 0.000000000000000000, -1.000000000000000000 ) ) ;
#8770=DIRECTION ( 'NONE',  ( 0.000000000000000000, 0.000000000000000000, 1.000000000000000000 ) ) ;
#8771=CARTESIAN_POINT ( 'NONE',  ( -18.05918829504999934, 10.97290950744599947, 27.09999999999999787 ) ) ;
#8772=CARTESIAN_POINT ( 'NONE',  ( -19.71007448221605074, 30.30175501178326414, 53.41939229818840573 ) ) ;
#8773=B_SPLINE_CURVE_WITH_KNOTS ( 'NONE', 3,
 ( #9525, #10717, #90, #7339, #2009, #8609, #4366, #5196, #6380, #12604, #7409, #3056, #11552, #6241, #13710, #4157, #8405, #12673, #3125, #11629, #1005, #4427, #4502, #5667, #10018, #6523, #373, #10788, #1203, #7684, #8820, #10931, #7764, #8894, #1484, #10858, #7618, #11969, #6733 ),
 .UNSPECIFIED., .F., .F.,
 ( 4, 2, 2, 2, 2, 1, 1, 2, 2, 2, 2, 2, 2, 2, 1, 1, 1, 2, 2, 2, 2, 4 ),
 ( 0.000000000000000000, 0.1250000000000901501, 0.1875000000001344480, 0.2187500000001581513, 0.2343750000001693645, 0.2421875000001743050, 0.2460937500001758038, 0.2480468750001765255, 0.2500000000001772471, 0.3750000000001733058, 0.5000000000001693090, 0.6250000000001654232, 0.6875000000001656453, 0.7187500000001668665, 0.7343750000001686429, 0.7421875000001706413, 0.7460937500001703082, 0.7480468750001699751, 0.7500000000001697531, 0.8125000000001261213, 0.8750000000000824896, 1.000000000000000000 ),
 .UNSPECIFIED. ) ;
#8774=DIRECTION ( 'NONE',  ( 0.000000000000000000, 0.000000000000000000, -1.000000000000000000 ) ) ;
#8775=ORIENTED_EDGE ( 'NONE', *, *, #6086, .F. ) ;
#8776=CARTESIAN_POINT ( 'NONE',  ( -3.531395436049983960, 18.23680593644601089, 62.03182374100001084 ) ) ;
#8777=FACE_BOUND ( 'NONE', #6246, .T. ) ;
#8781=ADVANCED_FACE ( 'NONE', ( #4206 ), #8452, .T. ) ;
#8782=EDGE_LOOP ( 'NONE', ( #7882, #8844, #8566, #4798, #3115, #12855, #12255, #11801 ) ) ;
#8783=EDGE_CURVE ( 'NONE', #665, #4627, #10169, .T. ) ;
#8786=DIRECTION ( 'NONE',  ( 0.08563346120589268584, 0.000000000000000000, -0.9963267086261908823 ) ) ;
#8793=FACE_OUTER_BOUND ( 'NONE', #7649, .T. ) ;
#8794=CARTESIAN_POINT ( 'NONE',  ( -30.80918829504999934, -6.027090492554000534, 64.85000000000000853 ) ) ;
#8796=EDGE_CURVE ( 'NONE', #13262, #11891, #4611, .T. ) ;
#8797=ORIENTED_EDGE ( 'NONE', *, *, #13338, .T. ) ;
#8799=ORIENTED_EDGE ( 'NONE', *, *, #7012, .T. ) ;
#8800=CARTESIAN_POINT ( 'NONE',  ( -15.41280400920135030, 7.973467857469549891, 30.59999999999999787 ) ) ;
#8803=DIRECTION ( 'NONE',  ( 0.6615960714621574867, -0.7498604124941119498, 0.000000000000000000 ) ) ;
#8804=VERTEX_POINT ( 'NONE', #5105 ) ;
#8806=DIRECTION ( 'NONE',  ( 0.000000000000000000, 0.000000000000000000, -1.000000000000000000 ) ) ;
#8811=ORIENTED_EDGE ( 'NONE', *, *, #986, .F. ) ;
#8812=FACE_OUTER_BOUND ( 'NONE', #11044, .T. ) ;
#8813=ORIENTED_EDGE ( 'NONE', *, *, #5160, .T. ) ;
#8814=ORIENTED_EDGE ( 'NONE', *, *, #5261, .F. ) ;
#8816=DIRECTION ( 'NONE',  ( 0.000000000000000000, 0.000000000000000000, -1.000000000000000000 ) ) ;
#8817=ADVANCED_FACE ( 'NONE', ( #1978 ), #5175, .T. ) ;
#8818=CARTESIAN_POINT ( 'NONE',  ( -12.04995946920099925, -4.929579886311989512, 62.14999999999999858 ) ) ;
#8820=CARTESIAN_POINT ( 'NONE',  ( -17.19771031368804515, 26.94970066966654798, 56.12204914942099521 ) ) ;
#8821=FACE_OUTER_BOUND ( 'NONE', #9068, .T. ) ;
#8822=AXIS2_PLACEMENT_3D ( 'NONE', #8632, #4385, #1163 ) ;
#8825=VERTEX_POINT ( 'NONE', #4135 ) ;
#8826=AXIS2_PLACEMENT_3D ( 'NONE', #13450, #10255, #1931 ) ;
#8827=CYLINDRICAL_SURFACE ( 'NONE', #1482, 16.95000000000000284 ) ;
#8828=ORIENTED_EDGE ( 'NONE', *, *, #8942, .T. ) ;
#8830=ORIENTED_EDGE ( 'NONE', *, *, #4185, .T. ) ;
#8831=EDGE_CURVE ( 'NONE', #5137, #13422, #13297, .T. ) ;
#8832=CARTESIAN_POINT ( 'NONE',  ( -30.30918829504999934, -6.027090492554000534, 68.85549045786049760 ) ) ;
#8833=CARTESIAN_POINT ( 'NONE',  ( -20.92870944094807584, 30.18239061225282427, 60.22698406536613192 ) ) ;
#8836=LINE ( 'NONE', #6672, #13800 ) ;
#8839=CARTESIAN_POINT ( 'NONE',  ( -14.95720466168106100, 17.08029827338444662, 64.54999999999999716 ) ) ;
#8840=AXIS2_PLACEMENT_3D ( 'NONE', #6216, #9446, #13690 ) ;
#8841=ORIENTED_EDGE ( 'NONE', *, *, #10756, .T. ) ;
#8843=DIRECTION ( 'NONE',  ( 0.000000000000000000, 0.000000000000000000, -1.000000000000000000 ) ) ;
#8844=ORIENTED_EDGE ( 'NONE', *, *, #4399, .F. ) ;
#8848=ORIENTED_EDGE ( 'NONE', *, *, #8102, .F. ) ;
#8850=EDGE_CURVE ( 'NONE', #12622, #5356, #6298, .T. ) ;
#8851=CARTESIAN_POINT ( 'NONE',  ( -5.789834139046019956, -5.598733283342819611, 68.85549045786049760 ) ) ;
#8852=CIRCLE ( 'NONE', #6830, 6.449999999999997513 ) ;
#8860=DIRECTION ( 'NONE',  ( 0.000000000000000000, 0.000000000000000000, -1.000000000000000000 ) ) ;
#8861=CARTESIAN_POINT ( 'NONE',  ( 2.262399129208275017, -0.4981161769137599782, 17.25000000000000000 ) ) ;
#8862=ADVANCED_FACE ( 'NONE', ( #1110 ), #13060, .T. ) ;
#8863=ORIENTED_EDGE ( 'NONE', *, *, #8316, .T. ) ;
#8864=ORIENTED_EDGE ( 'NONE', *, *, #8796, .F. ) ;
#8867=ORIENTED_EDGE ( 'NONE', *, *, #13528, .F. ) ;
#8868=EDGE_CURVE ( 'NONE', #6506, #13804, #2336, .T. ) ;
#8870=CYLINDRICAL_SURFACE ( 'NONE', #2412, 4.749999999999997335 ) ;
#8874=AXIS2_PLACEMENT_3D ( 'NONE', #2577, #12129, #5752 ) ;
#8876=CIRCLE ( 'NONE', #10427, 4.250000000000000000 ) ;
#8878=EDGE_CURVE ( 'NONE', #6060, #1530, #4824, .T. ) ;
#8880=AXIS2_PLACEMENT_3D ( 'NONE', #5861, #6068, #8444 ) ;
#8882=AXIS2_PLACEMENT_3D ( 'NONE', #12288, #1452, #1387 ) ;
#8886=CARTESIAN_POINT ( 'NONE',  ( -17.01567291573902807, 30.33713881007578195, 61.54486793806091782 ) ) ;
#8892=ORIENTED_EDGE ( 'NONE', *, *, #2614, .T. ) ;
#8894=CARTESIAN_POINT ( 'NONE',  ( -16.99569662973183171, 26.93820700769395771, 56.28689761106198119 ) ) ;
#8895=AXIS2_PLACEMENT_3D ( 'NONE', #12174, #2626, #1555 ) ;
#8896=CIRCLE ( 'NONE', #11790, 3.450000000000001510 ) ;
#8897=CYLINDRICAL_SURFACE ( 'NONE', #8917, 3.000000000000001332 ) ;
#8898=CIRCLE ( 'NONE', #6203, 17.00000000000000355 ) ;
#8899=EDGE_CURVE ( 'NONE', #1219, #318, #10629, .T. ) ;
#8902=CARTESIAN_POINT ( 'NONE',  ( -16.41522250449391152, 5.755460197997838812, 68.40012421657081632 ) ) ;
#8905=CIRCLE ( 'NONE', #3123, 17.00000000000000355 ) ;
#8906=FACE_OUTER_BOUND ( 'NONE', #12106, .T. ) ;
#8908=CARTESIAN_POINT ( 'NONE',  ( -21.29754790531509201, 30.13344396834369832, 55.03342513115495649 ) ) ;
#8912=DIRECTION ( 'NONE',  ( 0.7071067811865500152, 0.000000000000000000, 0.7071067811865450192 ) ) ;
#8913=CARTESIAN_POINT ( 'NONE',  ( -18.05918829504999934, 10.97290950744599947, 60.04999999999999716 ) ) ;
#8915=CARTESIAN_POINT ( 'NONE',  ( -18.05918829504999934, 10.97290950744599947, 57.35000000000000142 ) ) ;
#8916=ORIENTED_EDGE ( 'NONE', *, *, #3026, .T. ) ;
#8917=AXIS2_PLACEMENT_3D ( 'NONE', #12179, #11135, #313 ) ;
#8918=CIRCLE ( 'NONE', #4466, 2.000000000000001776 ) ;
#8920=EDGE_CURVE ( 'NONE', #13687, #2345, #12417, .T. ) ;
#8921=ORIENTED_EDGE ( 'NONE', *, *, #4456, .T. ) ;
#8923=FACE_OUTER_BOUND ( 'NONE', #12931, .T. ) ;
#8928=FACE_OUTER_BOUND ( 'NONE', #9100, .T. ) ;
#8930=AXIS2_PLACEMENT_3D ( 'NONE', #11357, #13579, #5894 ) ;
#8932=DIRECTION ( 'NONE',  ( 0.000000000000000000, 0.000000000000000000, 1.000000000000000000 ) ) ;
#8933=DIRECTION ( 'NONE',  ( 0.000000000000000000, 0.000000000000000000, 1.000000000000000000 ) ) ;
#8935=CARTESIAN_POINT ( 'NONE',  ( -3.125062480528954634, 3.387767046288379991, 58.54999999999999716 ) ) ;
#8936=B_SPLINE_CURVE_WITH_KNOTS ( 'NONE', 3,
 ( #9455, #11409, #9312, #13561, #8186, #12595, #8394, #3043, #1695, #12660, #11539, #10230, #6999, #10497, #647, #12451, #5185, #13697 ),
 .UNSPECIFIED., .F., .F.,
 ( 4, 2, 2, 2, 2, 2, 2, 2, 4 ),
 ( 0.000000000000000000, 0.1250000000000000000, 0.2500000000000000000, 0.3750000000000000000, 0.5000000000000000000, 0.6250000000000000000, 0.7500000000000000000, 0.8750000000000000000, 1.000000000000000000 ),
 .UNSPECIFIED. ) ;
#8937=CARTESIAN_POINT ( 'NONE',  ( -18.05918829430470041, 19.27290950744890097, 63.15000000009349179 ) ) ;
#8938=EDGE_CURVE ( 'NONE', #8958, #3979, #6563, .T. ) ;
#8940=AXIS2_PLACEMENT_3D ( 'NONE', #10630, #10567, #995 ) ;
#8942=EDGE_CURVE ( 'NONE', #3923, #8965, #1248, .T. ) ;
#8943=VERTEX_POINT ( 'NONE', #9786 ) ;
#8949=ADVANCED_FACE ( 'NONE', ( #6707 ), #8733, .T. ) ;
#8951=DIRECTION ( 'NONE',  ( 1.000000000000000000, 0.000000000000000000, 0.000000000000000000 ) ) ;
#8952=CARTESIAN_POINT ( 'NONE',  ( 0.000000000000000000, 0.000000000000000000, 17.25000000000000000 ) ) ;
#8953=CIRCLE ( 'NONE', #2949, 18.00000000000000000 ) ;
#8957=EDGE_CURVE ( 'NONE', #2414, #8660, #598, .T. ) ;
#8958=VERTEX_POINT ( 'NONE', #10694 ) ;
#8959=CYLINDRICAL_SURFACE ( 'NONE', #1216, 1.500000000000001332 ) ;
#8960=AXIS2_PLACEMENT_3D ( 'NONE', #6050, #1801, #8357 ) ;
#8961=VECTOR ( 'NONE', #3199, 1000.000000000000000 ) ;
#8962=ORIENTED_EDGE ( 'NONE', *, *, #10641, .T. ) ;
#8963=ORIENTED_EDGE ( 'NONE', *, *, #2330, .T. ) ;
#8964=ADVANCED_FACE ( 'NONE', ( #69 ), #8656, .T. ) ;
#8965=VERTEX_POINT ( 'NONE', #6500 ) ;
#8967=EDGE_LOOP ( 'NONE', ( #335, #11328, #1971, #953, #3400, #4420, #2518, #9585, #3245, #1231, #10845, #12718, #6801 ) ) ;
#8969=ORIENTED_EDGE ( 'NONE', *, *, #9657, .F. ) ;
#8970=CARTESIAN_POINT ( 'NONE',  ( -18.05918829504999934, 10.97290950744599947, 64.85000000000000853 ) ) ;
#8972=DIRECTION ( 'NONE',  ( 0.000000000000000000, 0.000000000000000000, -1.000000000000000000 ) ) ;
#8973=FACE_OUTER_BOUND ( 'NONE', #495, .T. ) ;
#8976=VERTEX_POINT ( 'NONE', #1535 ) ;
#8978=EDGE_CURVE ( 'NONE', #5838, #6577, #3357, .T. ) ;
#8979=CIRCLE ( 'NONE', #11428, 3.800000000000002487 ) ;
#8981=ORIENTED_EDGE ( 'NONE', *, *, #4118, .F. ) ;
#8983=CARTESIAN_POINT ( 'NONE',  ( -21.03590444521807967, 30.16892808484258737, 54.61432211296680350 ) ) ;
#8984=( LENGTH_UNIT ( ) NAMED_UNIT ( * ) SI_UNIT ( .MILLI., .METRE. ) );
#8985=DIRECTION ( 'NONE',  ( 0.6615960714621574867, -0.7498604124941119498, 0.000000000000000000 ) ) ;
#8986=LINE ( 'NONE', #3475, #2894 ) ;
#8987=DIRECTION ( 'NONE',  ( 0.000000000000000000, 0.000000000000000000, -1.000000000000000000 ) ) ;
#8988=DIRECTION ( 'NONE',  ( 0.000000000000000000, 0.000000000000000000, -1.000000000000000000 ) ) ;
#8989=VERTEX_POINT ( 'NONE', #11109 ) ;
#8990=AXIS2_PLACEMENT_3D ( 'NONE', #5393, #12869, #2141 ) ;
#8993=DIRECTION ( 'NONE',  ( 0.000000000000000000, 0.000000000000000000, 1.000000000000000000 ) ) ;
#8996=DIRECTION ( 'NONE',  ( 0.000000000000000000, 0.000000000000000000, -1.000000000000000000 ) ) ;
#8997=CARTESIAN_POINT ( 'NONE',  ( -7.241070169793059286, 29.81324547859994922, 17.25000000000000000 ) ) ;
#8998=CONICAL_SURFACE ( 'NONE', #2552, 4.250000000000000000, 0.7853981633974524978 ) ;
#8999=CARTESIAN_POINT ( 'NONE',  ( -25.64433075620760150, -3.961216307075045240, 58.54999999999999716 ) ) ;
#9001=LINE ( 'NONE', #4677, #1080 ) ;
#9002=CYLINDRICAL_SURFACE ( 'NONE', #10006, 16.95000000000000284 ) ;
#9003=ADVANCED_FACE ( 'NONE', ( #2753 ), #8870, .T. ) ;
#9006=CARTESIAN_POINT ( 'NONE',  ( -1.396365658198039927, 10.97290950744599947, 17.25000000000000000 ) ) ;
#9007=AXIS2_PLACEMENT_3D ( 'NONE', #11165, #547, #1390 ) ;
#9010=EDGE_LOOP ( 'NONE', ( #12477, #5082, #3518, #8451 ) ) ;
#9011=FACE_OUTER_BOUND ( 'NONE', #10472, .T. ) ;
#9012=CARTESIAN_POINT ( 'NONE',  ( -35.05918829505000645, -6.027090492554000534, 5.250000000000000000 ) ) ;
#9014=DIRECTION ( 'NONE',  ( 0.000000000000000000, 0.000000000000000000, -1.000000000000000000 ) ) ;
#9016=DIRECTION ( 'NONE',  ( 1.000000000000000000, 0.000000000000000000, 0.000000000000000000 ) ) ;
#9017=DIRECTION ( 'NONE',  ( 0.000000000000000000, 0.000000000000000000, -1.000000000000000000 ) ) ;
#9019=DIRECTION ( 'NONE',  ( 0.000000000000000000, 0.000000000000000000, -1.000000000000000000 ) ) ;
#9023=CARTESIAN_POINT ( 'NONE',  ( -16.56453087281537861, 30.31214524168932201, 61.35958320581661951 ) ) ;
#9024=EDGE_LOOP ( 'NONE', ( #11617, #8179, #6003, #11542 ) ) ;
#9032=DIRECTION ( 'NONE',  ( 0.000000000000000000, 0.000000000000000000, -1.000000000000000000 ) ) ;
#9033=DIRECTION ( 'NONE',  ( 0.000000000000000000, 0.000000000000000000, 1.000000000000000000 ) ) ;
#9035=DIRECTION ( 'NONE',  ( -1.000000000000000000, 0.000000000000000000, 0.000000000000000000 ) ) ;
#9036=ADVANCED_FACE ( 'NONE', ( #13407 ), #9977, .T. ) ;
#9039=CARTESIAN_POINT ( 'NONE',  ( -11.74835982676941981, -4.028726038184999858, 62.14999999999999858 ) ) ;
#9043=CARTESIAN_POINT ( 'NONE',  ( -21.62809706959791356, 30.08448262671908324, 58.92298932101692088 ) ) ;
#9044=PLANE ( 'NONE',  #4092 ) ;
#9045=DIRECTION ( 'NONE',  ( 0.000000000000000000, 0.000000000000000000, -1.000000000000000000 ) ) ;
#9046=DIRECTION ( 'NONE',  ( 0.000000000000000000, 0.000000000000000000, -1.000000000000000000 ) ) ;
#9047=CARTESIAN_POINT ( 'NONE',  ( -24.06841712089904917, -4.929579886311989512, 62.14999999999999858 ) ) ;
#9049=ADVANCED_FACE ( 'NONE', ( #554 ), #8401, .T. ) ;
#9050=VECTOR ( 'NONE', #8142, 1000.000000000000000 ) ;
#9051=DIRECTION ( 'NONE',  ( 0.000000000000000000, 0.000000000000000000, -1.000000000000000000 ) ) ;
#9053=FACE_OUTER_BOUND ( 'NONE', #7255, .T. ) ;
#9055=DIRECTION ( 'NONE',  ( 0.000000000000000000, 0.000000000000000000, -1.000000000000000000 ) ) ;
#9056=CARTESIAN_POINT ( 'NONE',  ( -22.99102692894637556, 13.28949390873614078, 68.40321543070255927 ) ) ;
#9057=CARTESIAN_POINT ( 'NONE',  ( -18.05918829504999934, 10.97290950744599947, 64.85000000000000853 ) ) ;
#9058=CARTESIAN_POINT ( 'NONE',  ( -7.241070169793070832, 29.81324547859995278, 83.57661607529820458 ) ) ;
#9062=DIRECTION ( 'NONE',  ( 1.000000000000000000, 0.000000000000000000, 0.000000000000000000 ) ) ;
#9065=CIRCLE ( 'NONE', #3283, 16.95000000000000284 ) ;
#9067=DIRECTION ( 'NONE',  ( 0.000000000000000000, 0.000000000000000000, 1.000000000000000000 ) ) ;
#9068=EDGE_LOOP ( 'NONE', ( #550, #8814, #12538, #5119 ) ) ;
#9069=VERTEX_POINT ( 'NONE', #4893 ) ;
#9070=DIRECTION ( 'NONE',  ( 0.000000000000000000, 0.000000000000000000, -1.000000000000000000 ) ) ;
#9071=DIRECTION ( 'NONE',  ( 0.000000000000000000, 0.000000000000000000, -1.000000000000000000 ) ) ;
#9077=CARTESIAN_POINT ( 'NONE',  ( -18.05918829504999934, 28.64232754551664684, 58.85000000000000142 ) ) ;
#9079=ORIENTED_EDGE ( 'NONE', *, *, #7390, .T. ) ;
#9080=EDGE_CURVE ( 'NONE', #13429, #12769, #8852, .T. ) ;
#9082=ORIENTED_EDGE ( 'NONE', *, *, #3935, .F. ) ;
#9083=CARTESIAN_POINT ( 'NONE',  ( -8.930582367738718830, 12.35910059330153921, 64.85000000000000853 ) ) ;
#9085=ORIENTED_EDGE ( 'NONE', *, *, #10564, .F. ) ;
#9086=VECTOR ( 'NONE', #10730, 1000.000000000000000 ) ;
#9087=FACE_BOUND ( 'NONE', #4441, .T. ) ;
#9090=CARTESIAN_POINT ( 'NONE',  ( -18.05918829504999934, 10.97290950744599947, 5.250000000000000000 ) ) ;
#9091=CARTESIAN_POINT ( 'NONE',  ( -23.24102627739274851, -6.265087914666300328, 62.14999999999999858 ) ) ;
#9092=DIRECTION ( 'NONE',  ( 0.000000000000000000, 0.000000000000000000, -1.000000000000000000 ) ) ;
#9093=CARTESIAN_POINT ( 'NONE',  ( 2.262399129208274129, 22.44393519180576746, 5.250000000000000000 ) ) ;
#9094=EDGE_CURVE ( 'NONE', #12141, #10905, #6398, .T. ) ;
#9095=DIRECTION ( 'NONE',  ( 0.000000000000000000, 0.000000000000000000, -1.000000000000000000 ) ) ;
#9097=AXIS2_PLACEMENT_3D ( 'NONE', #1037, #5432, #8644 ) ;
#9100=EDGE_LOOP ( 'NONE', ( #7079, #4810, #5222, #1228 ) ) ;
#9101=EDGE_CURVE ( 'NONE', #12100, #11802, #9065, .T. ) ;
#9102=EDGE_CURVE ( 'NONE', #956, #4939, #6159, .T. ) ;
#9108=CIRCLE ( 'NONE', #3773, 4.250000000000000000 ) ;
#9109=AXIS2_PLACEMENT_3D ( 'NONE', #11062, #1478, #5728 ) ;
#9110=CIRCLE ( 'NONE', #12681, 4.750000000000000888 ) ;
#9114=CARTESIAN_POINT ( 'NONE',  ( -21.28806243134481591, 30.13477816395881703, 55.01643572729695109 ) ) ;
#9115=EDGE_CURVE ( 'NONE', #10360, #8485, #2177, .T. ) ;
#9117=FACE_OUTER_BOUND ( 'NONE', #5800, .T. ) ;
#9119=DIRECTION ( 'NONE',  ( -1.000000000000000000, 0.000000000000000000, 0.000000000000000000 ) ) ;
#9125=CIRCLE ( 'NONE', #7741, 34.70000000000000284 ) ;
#9126=EDGE_CURVE ( 'NONE', #9069, #6829, #10864, .T. ) ;
#9127=CARTESIAN_POINT ( 'NONE',  ( -14.32322260522609980, 18.32852371459815188, 63.64999999999999858 ) ) ;
#9130=FACE_OUTER_BOUND ( 'NONE', #13144, .T. ) ;
#9131=DIRECTION ( 'NONE',  ( 0.000000000000000000, 0.000000000000000000, 1.000000000000000000 ) ) ;
#9133=FACE_OUTER_BOUND ( 'NONE', #10256, .T. ) ;
#9134=FACE_OUTER_BOUND ( 'NONE', #787, .T. ) ;
#9135=CARTESIAN_POINT ( 'NONE',  ( -35.05918829505000645, 10.97290950744599947, 64.35000000000000853 ) ) ;
#9137=FACE_OUTER_BOUND ( 'NONE', #2798, .T. ) ;
#9138=DIRECTION ( 'NONE',  ( 0.000000000000000000, 0.000000000000000000, 1.000000000000000000 ) ) ;
#9140=CIRCLE ( 'NONE', #2246, 0.9499999999999995115 ) ;
#9143=ORIENTED_EDGE ( 'NONE', *, *, #8783, .F. ) ;
#9145=AXIS2_PLACEMENT_3D ( 'NONE', #1829, #13542, #12433 ) ;
#9146=ORIENTED_EDGE ( 'NONE', *, *, #345, .T. ) ;
#9147=DIRECTION ( 'NONE',  ( 0.4528443260392610026, 0.8915896008669278450, 0.000000000000000000 ) ) ;
#9148=ORIENTED_EDGE ( 'NONE', *, *, #234, .T. ) ;
#9149=AXIS2_PLACEMENT_3D ( 'NONE', #8548, #2081, #10647 ) ;
#9153=EDGE_CURVE ( 'NONE', #6090, #12804, #4390, .T. ) ;
#9156=LINE ( 'NONE', #9999, #13797 ) ;
#9157=CARTESIAN_POINT ( 'NONE',  ( -18.05918829504999223, 2.756898754446003963, 63.36264408500002787 ) ) ;
#9159=DIRECTION ( 'NONE',  ( 1.000000000000000000, 0.000000000000000000, 0.000000000000000000 ) ) ;
#9161=( BOUNDED_CURVE ( )  B_SPLINE_CURVE ( 3, ( #2975, #843, #7123, #7189 ),
 .UNSPECIFIED., .F., .F. ) 
 B_SPLINE_CURVE_WITH_KNOTS ( ( 4, 4 ),
 ( 0.06314145700000579897, 0.9368585430000010428 ),
 .UNSPECIFIED. ) 
 CURVE ( )  GEOMETRIC_REPRESENTATION_ITEM ( )  RATIONAL_B_SPLINE_CURVE ( ( 0.9565783021659900465, 0.7697947703959749921, 0.7697947703959759913, 0.9565783021659940433 ) ) 
 REPRESENTATION_ITEM ( '' )  );
#9162=AXIS2_PLACEMENT_3D ( 'NONE', #2546, #6775, #4064 ) ;
#9163=CIRCLE ( 'NONE', #13175, 6.449999999999997513 ) ;
#9164=ORIENTED_EDGE ( 'NONE', *, *, #7879, .T. ) ;
#9166=ORIENTED_EDGE ( 'NONE', *, *, #9571, .F. ) ;
#9167=ORIENTED_EDGE ( 'NONE', *, *, #9218, .F. ) ;
#9169=CIRCLE ( 'NONE', #2950, 0.9499999999999995115 ) ;
#9173=EDGE_LOOP ( 'NONE', ( #13601, #9476, #11245, #6144 ) ) ;
#9174=CARTESIAN_POINT ( 'NONE',  ( -18.05918829505001355, 3.709013078446008027, 62.03182374100007479 ) ) ;
#9176=DIRECTION ( 'NONE',  ( 0.000000000000000000, -1.000000000000000000, 0.000000000000000000 ) ) ;
#9180=EDGE_CURVE ( 'NONE', #1281, #1970, #8515, .T. ) ;
#9181=CARTESIAN_POINT ( 'NONE',  ( -35.05918829505000645, 27.97290950744599769, 17.25000000000000000 ) ) ;
#9184=AXIS2_PLACEMENT_3D ( 'NONE', #7408, #11755, #11696 ) ;
#9185=CIRCLE ( 'NONE', #3831, 7.150000000000001243 ) ;
#9187=ORIENTED_EDGE ( 'NONE', *, *, #11704, .T. ) ;
#9188=ORIENTED_EDGE ( 'NONE', *, *, #1770, .F. ) ;
#9189=DIRECTION ( 'NONE',  ( -0.8915896008669277339, 0.4528443260392608916, 0.000000000000000000 ) ) ;
#9192=FACE_BOUND ( 'NONE', #2299, .T. ) ;
#9195=EDGE_CURVE ( 'NONE', #8965, #2082, #7265, .T. ) ;
#9198=EDGE_CURVE ( 'NONE', #3141, #6919, #12645, .T. ) ;
#9199=ORIENTED_EDGE ( 'NONE', *, *, #9452, .T. ) ;
#9200=ADVANCED_FACE ( 'NONE', ( #6552 ), #118, .T. ) ;
#9201=CIRCLE ( 'NONE', #951, 12.00000000000000355 ) ;
#9202=LINE ( 'NONE', #1867, #9050 ) ;
#9204=ORIENTED_EDGE ( 'NONE', *, *, #12256, .F. ) ;
#9205=DIRECTION ( 'NONE',  ( 0.000000000000000000, 0.000000000000000000, -1.000000000000000000 ) ) ;
#9206=CARTESIAN_POINT ( 'NONE',  ( -18.05918829504999934, 10.97290950744599947, 64.35000000000000853 ) ) ;
#9207=CARTESIAN_POINT ( 'NONE',  ( -10.25088531517540069, -8.860076549334108265, 5.250000000000000000 ) ) ;
#9208=CARTESIAN_POINT ( 'NONE',  ( -18.05918829504999934, 10.97290950744599947, 64.85000000000000853 ) ) ;
#9209=CARTESIAN_POINT ( 'NONE',  ( -25.32001676333059947, -4.028726038184999858, 63.45000000000000284 ) ) ;
#9211=CARTESIAN_POINT ( 'NONE',  ( -18.05918829504999934, 10.97290950744599947, 58.35000000000000142 ) ) ;
#9213=DIRECTION ( 'NONE',  ( 0.000000000000000000, 0.000000000000000000, -1.000000000000000000 ) ) ;
#9216=FACE_OUTER_BOUND ( 'NONE', #6941, .T. ) ;
#9217=PRODUCT_DEFINITION_CONTEXT ( 'detailed design', #4054, 'design' ) ;
#9218=EDGE_CURVE ( 'NONE', #4939, #956, #13756, .T. ) ;
#9225=CYLINDRICAL_SURFACE ( 'NONE', #12728, 4.250000000000000000 ) ;
#9226=CARTESIAN_POINT ( 'NONE',  ( -18.05918829504999934, 10.97290950744599947, 56.84999999999999432 ) ) ;
#9227=CARTESIAN_POINT ( 'NONE',  ( -23.49332020752115113, 0.2738342970428629952, 57.35000000000000142 ) ) ;
#9228=EDGE_CURVE ( 'NONE', #12616, #7297, #1306, .T. ) ;
#9231=CARTESIAN_POINT ( 'NONE',  ( -5.631644894983189431, 10.97290950744599947, 7.250000000000000000 ) ) ;
#9232=CIRCLE ( 'NONE', #744, 17.00000000000000355 ) ;
#9234=ORIENTED_EDGE ( 'NONE', *, *, #13366, .F. ) ;
#9236=CARTESIAN_POINT ( 'NONE',  ( -15.80158631607083564, 30.25033399978765658, 60.86361540000825698 ) ) ;
#9237=VERTEX_POINT ( 'NONE', #6483 ) ;
#9239=( LENGTH_UNIT ( ) NAMED_UNIT ( * ) SI_UNIT ( .MILLI., .METRE. ) );
#9240=CARTESIAN_POINT ( 'NONE',  ( -18.05918829505000289, 3.688421942730967906, 61.99499741764299898 ) ) ;
#9241=ORIENTED_EDGE ( 'NONE', *, *, #2542, .F. ) ;
#9242=VERTEX_POINT ( 'NONE', #55 ) ;
#9243=DIRECTION ( 'NONE',  ( 0.000000000000000000, 0.000000000000000000, -1.000000000000000000 ) ) ;
#9244=DIRECTION ( 'NONE',  ( 1.000000000000000000, 0.000000000000000000, 0.000000000000000000 ) ) ;
#9245=EDGE_LOOP ( 'NONE', ( #4277, #3614, #8520, #4061 ) ) ;
#9246=CARTESIAN_POINT ( 'NONE',  ( -6.600216501174579697, -2.179141222803619993, 63.45000000000000284 ) ) ;
#9247=LINE ( 'NONE', #3875, #6542 ) ;
#9248=CARTESIAN_POINT ( 'NONE',  ( -35.05918829505000645, -6.027090492554000534, 64.35000000000000853 ) ) ;
#9256=DIRECTION ( 'NONE',  ( -0.6615960714621568206, 0.7498604124941127269, 0.000000000000000000 ) ) ;
#9258=FACE_OUTER_BOUND ( 'NONE', #9426, .T. ) ;
#9259=DIRECTION ( 'NONE',  ( 0.000000000000000000, 0.000000000000000000, -1.000000000000000000 ) ) ;
#9261=DIRECTION ( 'NONE',  ( 0.000000000000000000, 0.000000000000000000, 1.000000000000000000 ) ) ;
#9263=ORIENTED_EDGE ( 'NONE', *, *, #8356, .T. ) ;
#9264=EDGE_CURVE ( 'NONE', #2555, #8732, #12898, .T. ) ;
#9266=AXIS2_PLACEMENT_3D ( 'NONE', #4613, #6833, #10984 ) ;
#9270=CARTESIAN_POINT ( 'NONE',  ( -28.87730642030695094, -7.867426463707980488, 17.25000000000000000 ) ) ;
#9271=FACE_OUTER_BOUND ( 'NONE', #13324, .T. ) ;
#9273=CARTESIAN_POINT ( 'NONE',  ( -22.82340340075558771, 13.43738685772752994, 68.48657388181956662 ) ) ;
#9274=CARTESIAN_POINT ( 'NONE',  ( -18.05918829504999934, 19.07290950615085023, 63.35000000000700027 ) ) ;
#9277=LINE ( 'NONE', #1946, #7413 ) ;
#9279=AXIS2_PLACEMENT_3D ( 'NONE', #8453, #12586, #10623 ) ;
#9282=ADVANCED_FACE ( 'NONE', ( #8637 ), #3347, .T. ) ;
#9283=DIRECTION ( 'NONE',  ( 0.000000000000000000, 0.000000000000000000, -1.000000000000000000 ) ) ;
#9285=ADVANCED_FACE ( 'NONE', ( #6612 ), #10648, .T. ) ;
#9287=ORIENTED_EDGE ( 'NONE', *, *, #1227, .F. ) ;
#9288=CARTESIAN_POINT ( 'NONE',  ( -1.059188295049996231, 27.97290950744599769, 58.85000000000000142 ) ) ;
#9290=LINE ( 'NONE', #8237, #6713 ) ;
#9293=ADVANCED_FACE ( 'NONE', ( #7375 ), #5425, .T. ) ;
#9297=ORIENTED_EDGE ( 'NONE', *, *, #10369, .T. ) ;
#9299=ORIENTED_EDGE ( 'NONE', *, *, #11570, .T. ) ;
#9300=CARTESIAN_POINT ( 'NONE',  ( -15.05138143747856638, 30.16479851545970092, 54.66128400976000989 ) ) ;
#9301=EDGE_LOOP ( 'NONE', ( #4666, #3234, #10680, #6727 ) ) ;
#9302=ORIENTED_EDGE ( 'NONE', *, *, #3377, .T. ) ;
#9303=CARTESIAN_POINT ( 'NONE',  ( -5.631644894983189431, 10.97290950744599947, 5.250000000000000000 ) ) ;
#9305=DIRECTION ( 'NONE',  ( 1.000000000000000000, 0.000000000000000000, 0.000000000000000000 ) ) ;
#9308=CARTESIAN_POINT ( 'NONE',  ( -35.05918829505000645, -6.027090492554000534, 7.250000000000000000 ) ) ;
#9309=EDGE_CURVE ( 'NONE', #9632, #11638, #11199, .T. ) ;
#9311=DIRECTION ( 'NONE',  ( 0.000000000000000000, 0.000000000000000000, -1.000000000000000000 ) ) ;
#9312=CARTESIAN_POINT ( 'NONE',  ( -19.52085246506412730, 27.91012756408683515, 57.74101035145125849 ) ) ;
#9314=VECTOR ( 'NONE', #9976, 1000.000000000000000 ) ;
#9316=VERTEX_POINT ( 'NONE', #7432 ) ;
#9317=CARTESIAN_POINT ( 'NONE',  ( -18.05918829504999934, 10.97290950744599947, 6.250000000000000000 ) ) ;
#9318=ORIENTED_EDGE ( 'NONE', *, *, #12598, .F. ) ;
#9320=CARTESIAN_POINT ( 'NONE',  ( -19.47982319660919615, 30.31714196969473463, 61.39763971179084479 ) ) ;
#9322=CARTESIAN_POINT ( 'NONE',  ( -25.33503448090910126, 29.19143287883919768, 64.85000000000000853 ) ) ;
#9323=AXIS2_PLACEMENT_3D ( 'NONE', #13456, #3900, #308 ) ;
#9324=CARTESIAN_POINT ( 'NONE',  ( -14.95720466168106100, 17.08029827338444662, 64.54999999999999716 ) ) ;
#9328=ORIENTED_EDGE ( 'NONE', *, *, #9386, .F. ) ;
#9329=ORIENTED_EDGE ( 'NONE', *, *, #3433, .F. ) ;
#9330=ORIENTED_EDGE ( 'NONE', *, *, #13261, .F. ) ;
#9332=AXIS2_PLACEMENT_3D ( 'NONE', #5601, #232, #2352 ) ;
#9333=LINE ( 'NONE', #12348, #11289 ) ;
#9335=ORIENTED_EDGE ( 'NONE', *, *, #10369, .F. ) ;
#9336=DIRECTION ( 'NONE',  ( -0.000000000000000000, -0.000000000000000000, 1.000000000000000000 ) ) ;
#9337=CYLINDRICAL_SURFACE ( 'NONE', #394, 2.700000000000000178 ) ;
#9338=CARTESIAN_POINT ( 'NONE',  ( -21.36716865236079954, 14.72221156991656166, 68.84999999999999432 ) ) ;
#9344=SURFACE_SIDE_STYLE ('',( #9425 ) ) ;
#9346=ORIENTED_EDGE ( 'NONE', *, *, #331, .T. ) ;
#9348=AXIS2_PLACEMENT_3D ( 'NONE', #4759, #9014, #13268 ) ;
#9349=AXIS2_PLACEMENT_3D ( 'NONE', #5148, #9423, #6054 ) ;
#9350=ADVANCED_FACE ( 'NONE', ( #1511 ), #2590, .F. ) ;
#9351=ADVANCED_FACE ( 'NONE', ( #2458 ), #9532, .T. ) ;
#9353=ORIENTED_EDGE ( 'NONE', *, *, #3213, .T. ) ;
#9358=CARTESIAN_POINT ( 'NONE',  ( -19.30446081463740882, 16.54212282176263926, 68.16277745478451777 ) ) ;
#9360=CIRCLE ( 'NONE', #10702, 6.000000000000002665 ) ;
#9363=DIRECTION ( 'NONE',  ( 0.000000000000000000, 0.000000000000000000, 1.000000000000000000 ) ) ;
#9364=CYLINDRICAL_SURFACE ( 'NONE', #12492, 23.22993838181875148 ) ;
#9365=EDGE_CURVE ( 'NONE', #3252, #1604, #7931, .T. ) ;
#9368=ORIENTED_EDGE ( 'NONE', *, *, #8487, .F. ) ;
#9370=CARTESIAN_POINT ( 'NONE',  ( -14.53639149466098957, 30.09164131421196942, 55.64423375431439212 ) ) ;
#9371=ORIENTED_EDGE ( 'NONE', *, *, #8634, .T. ) ;
#9372=ORIENTED_EDGE ( 'NONE', *, *, #11243, .T. ) ;
#9373=ORIENTED_EDGE ( 'NONE', *, *, #497, .F. ) ;
#9374=FACE_OUTER_BOUND ( 'NONE', #12362, .T. ) ;
#9375=CARTESIAN_POINT ( 'NONE',  ( -18.05918829504999934, 28.64232754551664684, 57.35000000000000142 ) ) ;
#9377=CARTESIAN_POINT ( 'NONE',  ( -10.47404583389237942, 25.90703532196704728, 58.54999999999999716 ) ) ;
#9378=CARTESIAN_POINT ( 'NONE',  ( -3.125062480528954634, 3.387767046288379991, 61.85000000000000142 ) ) ;
#9380=CARTESIAN_POINT ( 'NONE',  ( -18.05918829504999934, 10.97290950744599947, 116.8499999999999943 ) ) ;
#9381=CIRCLE ( 'NONE', #6472, 4.750000000000000888 ) ;
#9382=AXIS2_PLACEMENT_3D ( 'NONE', #6426, #5372, #6628 ) ;
#9385=CARTESIAN_POINT ( 'NONE',  ( -18.05918829504999934, 10.97290950744599947, 57.35000000000000142 ) ) ;
#9386=EDGE_CURVE ( 'NONE', #2748, #1420, #3689, .T. ) ;
#9387=CARTESIAN_POINT ( 'NONE',  ( -39.80918829504999934, 27.97290950744599769, 64.85000000000000853 ) ) ;
#9388=EDGE_CURVE ( 'NONE', #6784, #6589, #1446, .T. ) ;
#9390=ADVANCED_FACE ( 'NONE', ( #2659 ), #13249, .F. ) ;
#9393=AXIS2_PLACEMENT_3D ( 'NONE', #8052, #13293, #11209 ) ;
#9395=ORIENTED_EDGE ( 'NONE', *, *, #9198, .F. ) ;
#9396=ORIENTED_EDGE ( 'NONE', *, *, #2714, .F. ) ;
#9397=ORIENTED_EDGE ( 'NONE', *, *, #9820, .T. ) ;
#9399=DIRECTION ( 'NONE',  ( 0.000000000000000000, -2.202823461557850341E-15, 1.000000000000000000 ) ) ;
#9400=LINE ( 'NONE', #10435, #2774 ) ;
#9402=LINE ( 'NONE', #1789, #6505 ) ;
#9405=AXIS2_PLACEMENT_3D ( 'NONE', #1838, #2831, #13490 ) ;
#9406=AXIS2_PLACEMENT_3D ( 'NONE', #151, #6582, #5323 ) ;
#9408=VECTOR ( 'NONE', #8298, 1000.000000000000000 ) ;
#9410=MANIFOLD_SOLID_BREP ( 'NONE', #2812 ) ;
#9413=DIRECTION ( 'NONE',  ( -0.6615960714621564875, 0.7498604124941129490, 0.000000000000000000 ) ) ;
#9414=AXIS2_PLACEMENT_3D ( 'NONE', #1483, #516, #2630 ) ;
#9415=ORIENTED_EDGE ( 'NONE', *, *, #1161, .T. ) ;
#9416=ORIENTED_EDGE ( 'NONE', *, *, #6645, .F. ) ;
#9418=CARTESIAN_POINT ( 'NONE',  ( -18.05918829504999934, 10.97290950744599947, 23.90000000000000213 ) ) ;
#9419=FACE_BOUND ( 'NONE', #3080, .T. ) ;
#9421=ORIENTED_EDGE ( 'NONE', *, *, #12814, .F. ) ;
#9423=DIRECTION ( 'NONE',  ( 0.000000000000000000, 0.000000000000000000, 1.000000000000000000 ) ) ;
#9425=SURFACE_STYLE_FILL_AREA ( #10390 ) ;
#9426=EDGE_LOOP ( 'NONE', ( #4633, #4154, #13418, #7143, #12633, #7068 ) ) ;
#9428=ORIENTED_EDGE ( 'NONE', *, *, #10317, .F. ) ;
#9429=ORIENTED_EDGE ( 'NONE', *, *, #6857, .F. ) ;
#9433=VERTEX_POINT ( 'NONE', #668 ) ;
#9434=CARTESIAN_POINT ( 'NONE',  ( -20.26454227913669115, 15.69505033385297921, 68.63899161578964936 ) ) ;
#9435=CIRCLE ( 'NONE', #4960, 3.800000000000002487 ) ;
#9436=CARTESIAN_POINT ( 'NONE',  ( -22.64501676333060232, -4.028726038184999858, 62.14999999999999858 ) ) ;
#9437=EDGE_LOOP ( 'NONE', ( #83, #2110 ) ) ;
#9438=DIRECTION ( 'NONE',  ( 0.000000000000000000, 0.000000000000000000, 1.000000000000000000 ) ) ;
#9440=ORIENTED_EDGE ( 'NONE', *, *, #7142, .T. ) ;
#9441=CARTESIAN_POINT ( 'NONE',  ( -14.50040334037220369, 30.08605482697782918, 58.95214850063695167 ) ) ;
#9445=ORIENTED_EDGE ( 'NONE', *, *, #10856, .T. ) ;
#9446=DIRECTION ( 'NONE',  ( 0.000000000000000000, 0.000000000000000000, -1.000000000000000000 ) ) ;
#9448=ORIENTED_EDGE ( 'NONE', *, *, #4685, .F. ) ;
#9451=CARTESIAN_POINT ( 'NONE',  ( -35.05918829505000645, 10.97290950744599947, 63.54999999999999716 ) ) ;
#9452=EDGE_CURVE ( 'NONE', #9897, #6357, #13664, .T. ) ;
#9453=CARTESIAN_POINT ( 'NONE',  ( -39.30918829504999934, -6.027090492554000534, 58.85000000000000142 ) ) ;
#9454=AXIS2_PLACEMENT_3D ( 'NONE', #199, #4084, #12526 ) ;
#9455=CARTESIAN_POINT ( 'NONE',  ( -19.55918829504999934, 27.90660372932210009, 57.35000000000000142 ) ) ;
#9457=AXIS2_PLACEMENT_3D ( 'NONE', #3907, #2946, #751 ) ;
#9459=EDGE_CURVE ( 'NONE', #5647, #12210, #5496, .T. ) ;
#9462=VERTEX_POINT ( 'NONE', #1721 ) ;
#9465=CARTESIAN_POINT ( 'NONE',  ( -20.04118352984052720, 30.27579076659624135, 61.07633196088716687 ) ) ;
#9466=CARTESIAN_POINT ( 'NONE',  ( -35.05918829505000645, 27.97290950744599769, 64.85000000000000853 ) ) ;
#9476=ORIENTED_EDGE ( 'NONE', *, *, #754, .T. ) ;
#9479=FACE_OUTER_BOUND ( 'NONE', #12021, .T. ) ;
#9480=FACE_OUTER_BOUND ( 'NONE', #10273, .T. ) ;
#9481=ORIENTED_EDGE ( 'NONE', *, *, #8831, .T. ) ;
#9482=CARTESIAN_POINT ( 'NONE',  ( -11.74835982676941981, -4.028726038184999858, 62.14999999999999858 ) ) ;
#9483=DIRECTION ( 'NONE',  ( 1.000000000000000000, 0.000000000000000000, 0.000000000000000000 ) ) ;
#9484=DIRECTION ( 'NONE',  ( 1.000000000000000000, 0.000000000000000000, 0.000000000000000000 ) ) ;
#9489=EDGE_LOOP ( 'NONE', ( #637, #9765, #5085, #5589 ) ) ;
#9492=DIRECTION ( 'NONE',  ( 0.000000000000000000, 0.000000000000000000, -1.000000000000000000 ) ) ;
#9493=VERTEX_POINT ( 'NONE', #13384 ) ;
#9495=CARTESIAN_POINT ( 'NONE',  ( -30.30918829504999934, -6.027090492554000534, 7.250000000000000000 ) ) ;
#9496=CARTESIAN_POINT ( 'NONE',  ( -14.96009381531125015, 7.039309042655558457, 68.84999999999999432 ) ) ;
#9497=AXIS2_PLACEMENT_3D ( 'NONE', #10136, #5783, #12013 ) ;
#9498=CARTESIAN_POINT ( 'NONE',  ( -28.87730642030695094, -7.867426463707980488, 5.250000000000000000 ) ) ;
#9499=EDGE_CURVE ( 'NONE', #4952, #11290, #9754, .T. ) ;
#9501=CARTESIAN_POINT ( 'NONE',  ( -15.29370303376928852, 30.19507513566514234, 60.35551381422868644 ) ) ;
#9502=ORIENTED_EDGE ( 'NONE', *, *, #12632, .T. ) ;
#9507=DIRECTION ( 'NONE',  ( -1.000000000000000000, 0.000000000000000000, 0.000000000000000000 ) ) ;
#9509=CARTESIAN_POINT ( 'NONE',  ( -19.71317847370539766, 12.84756053868127879, 67.84999999999999432 ) ) ;
#9510=FACE_OUTER_BOUND ( 'NONE', #3481, .T. ) ;
#9511=CARTESIAN_POINT ( 'NONE',  ( -18.05918829504999223, 2.756898754446003963, 63.36264408500002787 ) ) ;
#9513=CARTESIAN_POINT ( 'NONE',  ( -9.759188295050000406, 10.97290950744599947, 61.86500000000000199 ) ) ;
#9514=ADVANCED_FACE ( 'NONE', ( #806 ), #5208, .F. ) ;
#9515=EDGE_CURVE ( 'NONE', #4114, #3872, #2024, .T. ) ;
#9519=ORIENTED_EDGE ( 'NONE', *, *, #8938, .T. ) ;
#9524=PLANE ( 'NONE',  #12310 ) ;
#9525=CARTESIAN_POINT ( 'NONE',  ( -19.47340185742309870, 26.91028695795525039, 56.84999999999999432 ) ) ;
#9526=DIRECTION ( 'NONE',  ( 0.000000000000000000, 0.000000000000000000, 1.000000000000000000 ) ) ;
#9527=CARTESIAN_POINT ( 'NONE',  ( -18.05918829504999934, 10.97290950744599947, 62.14999999999999858 ) ) ;
#9532=CONICAL_SURFACE ( 'NONE', #5280, 2.800000000000000266, 0.7853981633974419507 ) ;
#9533=EDGE_CURVE ( 'NONE', #1281, #11638, #10877, .T. ) ;
#9534=VERTEX_POINT ( 'NONE', #8293 ) ;
#9536=ADVANCED_FACE ( 'NONE', ( #11366 ), #10211, .T. ) ;
#9540=VECTOR ( 'NONE', #7165, 1000.000000000000000 ) ;
#9541=LINE ( 'NONE', #12618, #6934 ) ;
#9543=CIRCLE ( 'NONE', #2873, 6.000000000000002665 ) ;
#9544=DIRECTION ( 'NONE',  ( 0.4528443260392608360, 0.8915896008669278450, 0.000000000000000000 ) ) ;
#9545=EDGE_LOOP ( 'NONE', ( #6578, #10509, #9902, #3067 ) ) ;
#9546=FACE_OUTER_BOUND ( 'NONE', #11126, .T. ) ;
#9548=DIRECTION ( 'NONE',  ( 0.000000000000000000, 0.000000000000000000, -1.000000000000000000 ) ) ;
#9550=VERTEX_POINT ( 'NONE', #5003 ) ;
#9551=ADVANCED_FACE ( 'NONE', ( #9271 ), #9337, .F. ) ;
#9552=AXIS2_PLACEMENT_3D ( 'NONE', #10478, #11670, #6205 ) ;
#9555=AXIS2_PLACEMENT_3D ( 'NONE', #1785, #4852, #13368 ) ;
#9556=VERTEX_POINT ( 'NONE', #8215 ) ;
#9557=EDGE_CURVE ( 'NONE', #5483, #5782, #11988, .T. ) ;
#9559=CARTESIAN_POINT ( 'NONE',  ( -13.45272330285627582, 8.369250445964327767, 68.55863802020633102 ) ) ;
#9560=DIRECTION ( 'NONE',  ( 0.000000000000000000, 0.000000000000000000, -1.000000000000000000 ) ) ;
#9562=DIRECTION ( 'NONE',  ( -1.000000000000000000, 0.000000000000000000, 0.000000000000000000 ) ) ;
#9564=CIRCLE ( 'NONE', #4891, 0.9499999999999995115 ) ;
#9565=CARTESIAN_POINT ( 'NONE',  ( -15.27817205863298256, 6.758671056314481618, 68.81396957244685098 ) ) ;
#9567=DIRECTION ( 'NONE',  ( -1.000000000000000000, 0.000000000000000000, 0.000000000000000000 ) ) ;
#9570=AXIS2_PLACEMENT_3D ( 'NONE', #12227, #358, #7813 ) ;
#9571=EDGE_CURVE ( 'NONE', #10203, #1958, #8876, .T. ) ;
#9573=ORIENTED_EDGE ( 'NONE', *, *, #12093, .F. ) ;
#9575=DIRECTION ( 'NONE',  ( 0.000000000000000000, 0.000000000000000000, -1.000000000000000000 ) ) ;
#9577=CARTESIAN_POINT ( 'NONE',  ( -18.05918829504999934, 10.97290950744599947, 7.250000000000000000 ) ) ;
#9579=DIRECTION ( 'NONE',  ( 0.000000000000000000, 0.000000000000000000, 1.000000000000000000 ) ) ;
#9582=VECTOR ( 'NONE', #4249, 1000.000000000000114 ) ;
#9583=ORIENTED_EDGE ( 'NONE', *, *, #5217, .F. ) ;
#9585=ORIENTED_EDGE ( 'NONE', *, *, #13776, .T. ) ;
#9586=DIRECTION ( 'NONE',  ( -0.3132098788326386218, -0.9496839325805422893, 0.000000000000000000 ) ) ;
#9588=VERTEX_POINT ( 'NONE', #6391 ) ;
#9593=LINE ( 'NONE', #24, #7306 ) ;
#9594=EDGE_CURVE ( 'NONE', #7101, #10854, #11114, .T. ) ;
#9595=DIRECTION ( 'NONE',  ( 1.000000000000000000, 0.000000000000000000, 0.000000000000000000 ) ) ;
#9597=LINE ( 'NONE', #2354, #1368 ) ;
#9598=CARTESIAN_POINT ( 'NONE',  ( -24.80918829504999934, 10.97290950744599947, 63.35000000000000142 ) ) ;
#9599=EDGE_CURVE ( 'NONE', #4496, #12910, #9543, .T. ) ;
#9600=DIRECTION ( 'NONE',  ( 0.000000000000000000, 0.000000000000000000, -1.000000000000000000 ) ) ;
#9601=DIRECTION ( 'NONE',  ( 1.000000000000000000, 0.000000000000000000, 0.000000000000000000 ) ) ;
#9605=AXIS2_PLACEMENT_3D ( 'NONE', #13248, #12203, #6550 ) ;
#9606=CIRCLE ( 'NONE', #4042, 4.250000000000000000 ) ;
#9608=ORIENTED_EDGE ( 'NONE', *, *, #12434, .F. ) ;
#9609=LINE ( 'NONE', #10727, #12629 ) ;
#9610=LINE ( 'NONE', #3329, #5495 ) ;
#9614=CARTESIAN_POINT ( 'NONE',  ( -19.98782365351838664, 30.28009008643348210, 53.58950411947810721 ) ) ;
#9615=VECTOR ( 'NONE', #4078, 1000.000000000000000 ) ;
#9621=AXIS2_PLACEMENT_3D ( 'NONE', #8701, #11775, #1158 ) ;
#9622=EDGE_CURVE ( 'NONE', #8225, #12769, #9685, .T. ) ;
#9624=CARTESIAN_POINT ( 'NONE',  ( -26.35918829505000005, 10.97290950744599947, 63.14999999999999858 ) ) ;
#9625=ORIENTED_EDGE ( 'NONE', *, *, #7691, .F. ) ;
#9629=VECTOR ( 'NONE', #8525, 1000.000000000000000 ) ;
#9630=CIRCLE ( 'NONE', #4727, 6.299999999999998046 ) ;
#9631=CIRCLE ( 'NONE', #5375, 16.75000000000000355 ) ;
#9632=VERTEX_POINT ( 'NONE', #12817 ) ;
#9634=ORIENTED_EDGE ( 'NONE', *, *, #10096, .F. ) ;
#9636=ORIENTED_EDGE ( 'NONE', *, *, #8285, .F. ) ;
#9641=FACE_OUTER_BOUND ( 'NONE', #1078, .T. ) ;
#9643=CARTESIAN_POINT ( 'NONE',  ( -10.38347696868452097, 26.08535324214045303, 57.54999999999999716 ) ) ;
#9644=DIRECTION ( 'NONE',  ( -0.000000000000000000, -0.000000000000000000, -1.000000000000000000 ) ) ;
#9647=DIRECTION ( 'NONE',  ( 1.000000000000000000, 0.000000000000000000, 0.000000000000000000 ) ) ;
#9648=ORIENTED_EDGE ( 'NONE', *, *, #828, .F. ) ;
#9651=EDGE_CURVE ( 'NONE', #2296, #5838, #12442, .T. ) ;
#9653=CARTESIAN_POINT ( 'NONE',  ( -1.059188295049996231, 27.97290950744599769, 5.250000000000000000 ) ) ;
#9654=CARTESIAN_POINT ( 'NONE',  ( -22.95314638948480379, -5.307421391215619622, 62.14999999999999858 ) ) ;
#9657=EDGE_CURVE ( 'NONE', #4563, #707, #4859, .T. ) ;
#9658=DIRECTION ( 'NONE',  ( -1.000000000000000000, 0.000000000000000000, 0.000000000000000000 ) ) ;
#9661=EDGE_LOOP ( 'NONE', ( #12648, #10636, #10204, #8969, #13220, #4847, #12930, #3291, #2280 ) ) ;
#9664=ORIENTED_EDGE ( 'NONE', *, *, #3168, .F. ) ;
#9668=ORIENTED_EDGE ( 'NONE', *, *, #9386, .T. ) ;
#9672=FACE_BOUND ( 'NONE', #13402, .T. ) ;
#9675=DIRECTION ( 'NONE',  ( 0.4528443260392607250, 0.8915896008669278450, 0.000000000000000000 ) ) ;
#9676=DIRECTION ( 'NONE',  ( 0.000000000000000000, 0.000000000000000000, 1.000000000000000000 ) ) ;
#9678=VECTOR ( 'NONE', #12834, 1000.000000000000000 ) ;
#9679=EDGE_CURVE ( 'NONE', #2014, #4651, #3269, .T. ) ;
#9682=EDGE_LOOP ( 'NONE', ( #1293, #12393 ) ) ;
#9685=LINE ( 'NONE', #3138, #9086 ) ;
#9686=CARTESIAN_POINT ( 'NONE',  ( -20.51890800742826571, 30.22967062585348685, 54.01748261881041913 ) ) ;
#9687=DIRECTION ( 'NONE',  ( 0.000000000000000000, 0.000000000000000000, -1.000000000000000000 ) ) ;
#9688=ORIENTED_EDGE ( 'NONE', *, *, #11038, .T. ) ;
#9689=DIRECTION ( 'NONE',  ( 1.000000000000000000, 0.000000000000000000, 0.000000000000000000 ) ) ;
#9691=DIRECTION ( 'NONE',  ( 0.6615960714621572647, -0.7498604124941123938, 0.000000000000000000 ) ) ;
#9696=ORIENTED_EDGE ( 'NONE', *, *, #10071, .T. ) ;
#9697=CARTESIAN_POINT ( 'NONE',  ( -30.80918829504999934, 27.97290950744599769, 64.85000000000000853 ) ) ;
#9698=ORIENTED_EDGE ( 'NONE', *, *, #7658, .T. ) ;
#9700=DIRECTION ( 'NONE',  ( -1.000000000000000000, 0.000000000000000000, 0.000000000000000000 ) ) ;
#9701=CARTESIAN_POINT ( 'NONE',  ( 2.262399129208279902, 22.44393519180574970, 17.25000000000000000 ) ) ;
#9702=CARTESIAN_POINT ( 'NONE',  ( -11.38420496205000099, 17.64789284044599782, 60.40999999999999659 ) ) ;
#9704=DIRECTION ( 'NONE',  ( 0.000000000000000000, 0.000000000000000000, -1.000000000000000000 ) ) ;
#9705=CARTESIAN_POINT ( 'NONE',  ( -18.05918829504999934, 10.97290950744599947, 5.250000000000000000 ) ) ;
#9707=LINE ( 'NONE', #10687, #1990 ) ;
#9708=CONICAL_SURFACE ( 'NONE', #7230, 4.250000000000000000, 0.7853981633974518317 ) ;
#9711=CARTESIAN_POINT ( 'NONE',  ( -15.83529908340206305, 30.25357667928068750, 53.80883379359870133 ) ) ;
#9712=ORIENTED_EDGE ( 'NONE', *, *, #5706, .F. ) ;
#9713=DIRECTION ( 'NONE',  ( 0.000000000000000000, 1.000000000000000000, 0.000000000000000000 ) ) ;
#9714=EDGE_CURVE ( 'NONE', #2711, #6329, #1494, .T. ) ;
#9720=FACE_OUTER_BOUND ( 'NONE', #4844, .T. ) ;
#9722=EDGE_CURVE ( 'NONE', #6494, #4217, #6177, .T. ) ;
#9723=AXIS2_PLACEMENT_3D ( 'NONE', #11363, #877, #2933 ) ;
#9724=ORIENTED_EDGE ( 'NONE', *, *, #2823, .F. ) ;
#9725=CARTESIAN_POINT ( 'NONE',  ( -18.05918829504999934, 2.872909508741170015, 63.35000000000700027 ) ) ;
#9728=ORIENTED_EDGE ( 'NONE', *, *, #7822, .F. ) ;
#9735=FACE_OUTER_BOUND ( 'NONE', #4691, .T. ) ;
#9736=CARTESIAN_POINT ( 'NONE',  ( -18.05918829504999934, 19.05294282444599929, 63.34900083300000517 ) ) ;
#9737=DIRECTION ( 'NONE',  ( 0.000000000000000000, 0.000000000000000000, -1.000000000000000000 ) ) ;
#9738=DIRECTION ( 'NONE',  ( 0.000000000000000000, 0.000000000000000000, -1.000000000000000000 ) ) ;
#9747=CARTESIAN_POINT ( 'NONE',  ( -20.26821253650571464, 30.25500104533646706, 53.79675021559635439 ) ) ;
#9751=CARTESIAN_POINT ( 'NONE',  ( -18.05918829504999934, 18.59295644444599915, 61.63595870800000398 ) ) ;
#9752=DIRECTION ( 'NONE',  ( 0.000000000000000000, 0.000000000000000000, 1.000000000000000000 ) ) ;
#9754=CIRCLE ( 'NONE', #6841, 17.00000000000000355 ) ;
#9755=DIRECTION ( 'NONE',  ( -0.2878798879079283446, 0.9576665234506834823, 0.000000000000000000 ) ) ;
#9756=CIRCLE ( 'NONE', #13760, 2.000000000000001776 ) ;
#9758=CIRCLE ( 'NONE', #11543, 8.250000000000001776 ) ;
#9760=EDGE_CURVE ( 'NONE', #7877, #11930, #382, .T. ) ;
#9764=FACE_OUTER_BOUND ( 'NONE', #10336, .T. ) ;
#9765=ORIENTED_EDGE ( 'NONE', *, *, #8301, .F. ) ;
#9766=CARTESIAN_POINT ( 'NONE',  ( -18.05918829504999934, 10.97290950744599947, 118.8499999999999943 ) ) ;
#9767=CARTESIAN_POINT ( 'NONE',  ( -19.55918829504999934, 27.40458623260099813, 57.35000000000000142 ) ) ;
#9768=DIRECTION ( 'NONE',  ( -1.000000000000000000, 0.000000000000000000, 0.000000000000000000 ) ) ;
#9773=CARTESIAN_POINT ( 'NONE',  ( -18.05918829504999934, 10.97290950744599947, 64.85000000000000853 ) ) ;
#9775=DIRECTION ( 'NONE',  ( 0.000000000000000000, 0.000000000000000000, -1.000000000000000000 ) ) ;
#9780=ORIENTED_EDGE ( 'NONE', *, *, #13638, .F. ) ;
#9781=CARTESIAN_POINT ( 'NONE',  ( -15.18966715138324020, 30.18239061250415034, 54.47301593183773605 ) ) ;
#9782=AXIS2_PLACEMENT_3D ( 'NONE', #63, #3356, #1175 ) ;
#9784=VECTOR ( 'NONE', #2045, 1000.000000000000000 ) ;
#9786=CARTESIAN_POINT ( 'NONE',  ( -41.50918829505000218, 27.97290950744599769, 5.250000000000000000 ) ) ;
#9787=CIRCLE ( 'NONE', #2896, 6.450000000000001066 ) ;
#9789=CARTESIAN_POINT ( 'NONE',  ( -18.05918829504999934, 7.130333642789880244, 83.57661607529820458 ) ) ;
#9793=EDGE_CURVE ( 'NONE', #6107, #1219, #10947, .T. ) ;
#9794=FACE_OUTER_BOUND ( 'NONE', #5506, .T. ) ;
#9796=STYLED_ITEM ( 'NONE', ( #4049 ), #13799 ) ;
#9798=VECTOR ( 'NONE', #3905, 1000.000000000000000 ) ;
#9799=VECTOR ( 'NONE', #5473, 1000.000000000000000 ) ;
#9800=ADVANCED_FACE ( 'NONE', ( #1431 ), #8630, .T. ) ;
#9801=B_SPLINE_CURVE_WITH_KNOTS ( 'NONE', 3,
 ( #1313, #9496, #9565, #1101, #13743, #12709, #11669, #7378, #8573, #2111, #8902, #3286, #4269 ),
 .UNSPECIFIED., .F., .F.,
 ( 4, 1, 1, 1, 1, 1, 2, 2, 4 ),
 ( 0.000000000000000000, 0.2500000000000021649, 0.3750000000000038303, 0.4375000000000054401, 0.4687500000000050515, 0.4843750000000056621, 0.4921875000000059397, 0.5000000000000062172, 1.000000000000000000 ),
 .UNSPECIFIED. ) ;
#9803=ORIENTED_EDGE ( 'NONE', *, *, #6916, .T. ) ;
#9804=DIRECTION ( 'NONE',  ( 1.000000000000000000, 0.000000000000000000, 0.000000000000000000 ) ) ;
#9806=ORIENTED_EDGE ( 'NONE', *, *, #7389, .F. ) ;
#9807=( NAMED_UNIT ( * ) PLANE_ANGLE_UNIT ( ) SI_UNIT ( $, .RADIAN. ) );
#9809=DIRECTION ( 'NONE',  ( 0.000000000000000000, 1.000000000000000000, 0.000000000000000000 ) ) ;
#9810=EDGE_CURVE ( 'NONE', #9989, #6506, #3053, .T. ) ;
#9811=EDGE_LOOP ( 'NONE', ( #8148, #5403, #9085, #7892 ) ) ;
#9812=FACE_OUTER_BOUND ( 'NONE', #12458, .T. ) ;
#9813=AXIS2_PLACEMENT_3D ( 'NONE', #1486, #5734, #446 ) ;
#9814=CARTESIAN_POINT ( 'NONE',  ( -1.059188295049996231, -6.027090492554000534, 64.35000000000000853 ) ) ;
#9815=FACE_BOUND ( 'NONE', #557, .T. ) ;
#9816=FACE_OUTER_BOUND ( 'NONE', #3863, .T. ) ;
#9817=EDGE_CURVE ( 'NONE', #5387, #6884, #7964, .T. ) ;
#9820=EDGE_CURVE ( 'NONE', #8318, #2826, #9758, .T. ) ;
#9824=ORIENTED_EDGE ( 'NONE', *, *, #10133, .T. ) ;
#9825=CARTESIAN_POINT ( 'NONE',  ( -29.51816008892539855, -2.179141222803634648, 62.14999999999999858 ) ) ;
#9826=ORIENTED_EDGE ( 'NONE', *, *, #9760, .F. ) ;
#9827=FACE_OUTER_BOUND ( 'NONE', #4263, .T. ) ;
#9832=CARTESIAN_POINT ( 'NONE',  ( -19.59368177784231335, 30.30953598072430921, 53.36020361897907804 ) ) ;
#9835=CARTESIAN_POINT ( 'NONE',  ( -25.89252162804999813, 10.97290950744599947, 60.04999999999999716 ) ) ;
#9836=LINE ( 'NONE', #107, #260 ) ;
#9837=CARTESIAN_POINT ( 'NONE',  ( -13.05918829504999756, 10.97290950744599947, 118.8499999999999943 ) ) ;
#9838=CIRCLE ( 'NONE', #3805, 6.449999999999997513 ) ;
#9839=CIRCLE ( 'NONE', #5572, 23.22993838181875148 ) ;
#9841=CIRCLE ( 'NONE', #5573, 4.750000000000000888 ) ;
#9842=ORIENTED_EDGE ( 'NONE', *, *, #428, .T. ) ;
#9843=VECTOR ( 'NONE', #5569, 1000.000000000000000 ) ;
#9844=EDGE_CURVE ( 'NONE', #2384, #12622, #614, .T. ) ;
#9846=ORIENTED_EDGE ( 'NONE', *, *, #7645, .T. ) ;
#9848=AXIS2_PLACEMENT_3D ( 'NONE', #2368, #12955, #3468 ) ;
#9849=FACE_OUTER_BOUND ( 'NONE', #9010, .T. ) ;
#9850=AXIS2_PLACEMENT_3D ( 'NONE', #10609, #1961, #8571 ) ;
#9851=AXIS2_PLACEMENT_3D ( 'NONE', #5702, #484, #6826 ) ;
#9854=DIRECTION ( 'NONE',  ( 0.6615960714621565986, -0.7498604124941126159, 0.000000000000000000 ) ) ;
#9856=CARTESIAN_POINT ( 'NONE',  ( -24.37001676333060018, -4.028726038184999858, 63.45000000000000284 ) ) ;
#9858=DIRECTION ( 'NONE',  ( -1.000000000000000000, 0.000000000000000000, 0.000000000000000000 ) ) ;
#9859=DIRECTION ( 'NONE',  ( -0.7071067811865474617, 8.659560562354903276E-17, 0.7071067811865474617 ) ) ;
#9863=ORIENTED_EDGE ( 'NONE', *, *, #12732, .T. ) ;
#9865=CARTESIAN_POINT ( 'NONE',  ( -17.23229456089049805, 30.34555471844711505, 53.09492650809716707 ) ) ;
#9866=DIRECTION ( 'NONE',  ( 0.000000000000000000, 0.000000000000000000, 1.000000000000000000 ) ) ;
#9868=FACE_OUTER_BOUND ( 'NONE', #11450, .T. ) ;
#9870=CYLINDRICAL_SURFACE ( 'NONE', #2507, 4.749999999999997335 ) ;
#9871=AXIS2_PLACEMENT_3D ( 'NONE', #154, #12871, #1007 ) ;
#9873=DIRECTION ( 'NONE',  ( 0.000000000000000000, 0.000000000000000000, 1.000000000000000000 ) ) ;
#9875=MECHANICAL_DESIGN_GEOMETRIC_PRESENTATION_REPRESENTATION('',(#7617),#2535);
#9879=CARTESIAN_POINT ( 'NONE',  ( -18.05918829504999934, 10.97290950744599947, 57.35000000000000142 ) ) ;
#9882=ORIENTED_EDGE ( 'NONE', *, *, #3243, .F. ) ;
#9883=VERTEX_POINT ( 'NONE', #13647 ) ;
#9885=CARTESIAN_POINT ( 'NONE',  ( -18.05918829504999934, 10.97290950744599947, 27.09999999999999787 ) ) ;
#9888=DIRECTION ( 'NONE',  ( 1.000000000000000000, 0.000000000000000000, 0.000000000000000000 ) ) ;
#9890=FACE_OUTER_BOUND ( 'NONE', #4400, .T. ) ;
#9891=CARTESIAN_POINT ( 'NONE',  ( -1.059188295049996231, -6.027090492554000534, 64.85000000000000853 ) ) ;
#9894=FACE_OUTER_BOUND ( 'NONE', #8024, .T. ) ;
#9895=EDGE_LOOP ( 'NONE', ( #4218, #3880, #10715, #1957 ) ) ;
#9897=VERTEX_POINT ( 'NONE', #1640 ) ;
#9899=EDGE_CURVE ( 'NONE', #918, #6678, #8210, .T. ) ;
#9900=CARTESIAN_POINT ( 'NONE',  ( -21.30549241498041013, 30.13232420323818062, 59.65220830260756202 ) ) ;
#9901=( BOUNDED_CURVE ( )  B_SPLINE_CURVE ( 3, ( #11384, #11457, #6285, #5165 ),
 .UNSPECIFIED., .F., .F. ) 
 B_SPLINE_CURVE_WITH_KNOTS ( ( 4, 4 ),
 ( 0.000000000000000000, 1.000000000000000000 ),
 .UNSPECIFIED. ) 
 CURVE ( )  GEOMETRIC_REPRESENTATION_ITEM ( )  RATIONAL_B_SPLINE_CURVE ( ( 0.9565783017328499671, 0.3188594339109500075, 0.3188594339109500075, 0.9565783017328499671 ) ) 
 REPRESENTATION_ITEM ( '' )  );
#9902=ORIENTED_EDGE ( 'NONE', *, *, #11721, .T. ) ;
#9905=DIRECTION ( 'NONE',  ( 0.7071067811865505703, 0.000000000000000000, 0.7071067811865444641 ) ) ;
#9907=LINE ( 'NONE', #4525, #2705 ) ;
#9908=EDGE_CURVE ( 'NONE', #10213, #12141, #6094, .T. ) ;
#9909=ORIENTED_EDGE ( 'NONE', *, *, #2071, .T. ) ;
#9911=VERTEX_POINT ( 'NONE', #8064 ) ;
#9912=CARTESIAN_POINT ( 'NONE',  ( -38.38077571930826082, 22.44393519180575680, 83.57661607529820458 ) ) ;
#9914=VECTOR ( 'NONE', #12516, 1000.000000000000000 ) ;
#9915=CARTESIAN_POINT ( 'NONE',  ( -18.05918829504999934, 10.97290950744599947, 61.85000000000000142 ) ) ;
#9917=DIRECTION ( 'NONE',  ( 1.000000000000000000, 0.000000000000000000, 0.000000000000000000 ) ) ;
#9918=DIRECTION ( 'NONE',  ( 0.000000000000000000, 0.000000000000000000, 1.000000000000000000 ) ) ;
#9919=PLANE ( 'NONE',  #4735 ) ;
#9920=CARTESIAN_POINT ( 'NONE',  ( -18.05918829504999934, 10.97290950744599947, 57.35000000000000142 ) ) ;
#9921=CARTESIAN_POINT ( 'NONE',  ( -25.86749127492460332, 30.80589556422609476, 5.250000000000000000 ) ) ;
#9922=CARTESIAN_POINT ( 'NONE',  ( -16.64497473267689998, 26.91028695795525039, 56.84999999999999432 ) ) ;
#9923=CARTESIAN_POINT ( 'NONE',  ( -39.80918829504999934, 27.97290950744599769, 7.250000000000000000 ) ) ;
#9927=DIRECTION ( 'NONE',  ( 0.000000000000000000, 0.000000000000000000, -1.000000000000000000 ) ) ;
#9928=ADVANCED_FACE ( 'NONE', ( #6028 ), #12396, .T. ) ;
#9929=DIRECTION ( 'NONE',  ( 1.000000000000000000, 0.000000000000000000, 0.000000000000000000 ) ) ;
#9931=CARTESIAN_POINT ( 'NONE',  ( -18.05918829504999934, 10.97290950744599947, 57.35000000000000142 ) ) ;
#9934=DIRECTION ( 'NONE',  ( 0.000000000000000000, 0.000000000000000000, -1.000000000000000000 ) ) ;
#9935=ORIENTED_EDGE ( 'NONE', *, *, #11594, .F. ) ;
#9936=CIRCLE ( 'NONE', #8367, 0.9499999999999995115 ) ;
#9937=FACE_OUTER_BOUND ( 'NONE', #10849, .T. ) ;
#9938=VERTEX_POINT ( 'NONE', #725 ) ;
#9939=ORIENTED_EDGE ( 'NONE', *, *, #11090, .F. ) ;
#9941=CARTESIAN_POINT ( 'NONE',  ( -18.05918829504999934, 3.815137874446000055, 61.70038048199999281 ) ) ;
#9944=CARTESIAN_POINT ( 'NONE',  ( -18.05918829504999934, 19.07290950615085023, 63.35000000000700027 ) ) ;
#9946=EDGE_CURVE ( 'NONE', #2296, #9588, #6160, .T. ) ;
#9950=CARTESIAN_POINT ( 'NONE',  ( -5.789834139046019956, -5.598733283342819611, 64.85000000000000853 ) ) ;
#9951=EDGE_CURVE ( 'NONE', #3112, #1146, #12892, .T. ) ;
#9955=ORIENTED_EDGE ( 'NONE', *, *, #9651, .F. ) ;
#9957=CARTESIAN_POINT ( 'NONE',  ( -20.63590450610939087, 30.21696533308443122, 60.56576002470140452 ) ) ;
#9958=ORIENTED_EDGE ( 'NONE', *, *, #8003, .T. ) ;
#9959=CARTESIAN_POINT ( 'NONE',  ( 3.190811704950004657, -6.027090492554000534, 64.35000000000000853 ) ) ;
#9961=PLANE ( 'NONE',  #695 ) ;
#9963=DIRECTION ( 'NONE',  ( -1.000000000000000000, 0.000000000000000000, 0.000000000000000000 ) ) ;
#9965=VERTEX_POINT ( 'NONE', #8540 ) ;
#9966=ORIENTED_EDGE ( 'NONE', *, *, #8335, .T. ) ;
#9967=VECTOR ( 'NONE', #3236, 1000.000000000000000 ) ;
#9971=VERTEX_POINT ( 'NONE', #12803 ) ;
#9973=CARTESIAN_POINT ( 'NONE',  ( -16.40519811639460102, 9.098258476210720147, 67.84999999999999432 ) ) ;
#9976=DIRECTION ( 'NONE',  ( 3.441911658684139926E-17, 0.000000000000000000, 1.000000000000000000 ) ) ;
#9977=TOROIDAL_SURFACE ( 'NONE', #12849, 10.00000000000000000, 2.000000000000000000 ) ;
#9978=DIRECTION ( 'NONE',  ( 0.000000000000000000, 0.000000000000000000, -1.000000000000000000 ) ) ;
#9979=CARTESIAN_POINT ( 'NONE',  ( -10.78334210919089919, -7.245613863947199640, 64.85000000000000853 ) ) ;
#9986=DIRECTION ( 'NONE',  ( 1.000000000000000000, 0.000000000000000000, 0.000000000000000000 ) ) ;
#9987=ADVANCED_FACE ( 'NONE', ( #8678 ), #7752, .T. ) ;
#9989=VERTEX_POINT ( 'NONE', #3254 ) ;
#9991=FACE_BOUND ( 'NONE', #11524, .T. ) ;
#9993=ORIENTED_EDGE ( 'NONE', *, *, #6271, .F. ) ;
#9996=CIRCLE ( 'NONE', #3971, 6.449999999999997513 ) ;
#9997=DIRECTION ( 'NONE',  ( -1.000000000000000000, 0.000000000000000000, 0.000000000000000000 ) ) ;
#9998=AXIS2_PLACEMENT_3D ( 'NONE', #10574, #4873, #4224 ) ;
#9999=CARTESIAN_POINT ( 'NONE',  ( -7.241070169793059286, -7.867426463707969830, 17.25000000000000000 ) ) ;
#10000=AXIS2_PLACEMENT_3D ( 'NONE', #8771, #7700, #4787 ) ;
#10005=AXIS2_PLACEMENT_3D ( 'NONE', #11469, #1906, #6145 ) ;
#10006=AXIS2_PLACEMENT_3D ( 'NONE', #9920, #6765, #6894 ) ;
#10007=AXIS2_PLACEMENT_3D ( 'NONE', #9317, #863, #5124 ) ;
#10008=CARTESIAN_POINT ( 'NONE',  ( -34.25918829536686872, 19.07290950803865215, 63.35000000001154774 ) ) ;
#10011=ORIENTED_EDGE ( 'NONE', *, *, #11452, .F. ) ;
#10012=VERTEX_POINT ( 'NONE', #7538 ) ;
#10014=FACE_OUTER_BOUND ( 'NONE', #11308, .T. ) ;
#10016=DIRECTION ( 'NONE',  ( 1.000000000000000000, 0.000000000000000000, 0.000000000000000000 ) ) ;
#10017=AXIS2_PLACEMENT_3D ( 'NONE', #8017, #12292, #9986 ) ;
#10018=CARTESIAN_POINT ( 'NONE',  ( -17.33982109643458003, 26.95666986121975484, 56.03305621834116579 ) ) ;
#10019=AXIS2_PLACEMENT_3D ( 'NONE', #12522, #708, #2978 ) ;
#10020=AXIS2_PLACEMENT_3D ( 'NONE', #3013, #4116, #5907 ) ;
#10021=CYLINDRICAL_SURFACE ( 'NONE', #4020, 4.250000000000000000 ) ;
#10022=AXIS2_PLACEMENT_3D ( 'NONE', #846, #2979, #7192 ) ;
#10023=DIRECTION ( 'NONE',  ( 1.000000000000000000, 0.000000000000000000, 0.000000000000000000 ) ) ;
#10024=VERTEX_POINT ( 'NONE', #11827 ) ;
#10025=VERTEX_POINT ( 'NONE', #6447 ) ;
#10027=EDGE_CURVE ( 'NONE', #1852, #12322, #2214, .T. ) ;
#10029=ORIENTED_EDGE ( 'NONE', *, *, #12613, .T. ) ;
#10036=DIRECTION ( 'NONE',  ( 0.000000000000000000, 0.000000000000000000, -1.000000000000000000 ) ) ;
#10037=CARTESIAN_POINT ( 'NONE',  ( -21.57405949846663873, 30.09282919895730046, 55.62766450024737708 ) ) ;
#10038=FILL_AREA_STYLE_COLOUR ( '', #7627 ) ;
#10039=CARTESIAN_POINT ( 'NONE',  ( -35.05918829505000645, 27.97290950744599769, 64.85000000000000853 ) ) ;
#10040=DIRECTION ( 'NONE',  ( 0.000000000000000000, -1.000000000000000000, 0.000000000000000000 ) ) ;
#10041=DIRECTION ( 'NONE',  ( 1.000000000000000000, 1.460819769243626736E-15, 0.000000000000000000 ) ) ;
#10042=CARTESIAN_POINT ( 'NONE',  ( -1.059188295049996231, 27.97290950744599769, 17.25000000000000000 ) ) ;
#10043=ORIENTED_EDGE ( 'NONE', *, *, #9264, .T. ) ;
#10045=AXIS2_PLACEMENT_3D ( 'NONE', #11197, #7052, #7122 ) ;
#10047=ORIENTED_EDGE ( 'NONE', *, *, #6744, .F. ) ;
#10052=DIRECTION ( 'NONE',  ( 0.6615960714621574867, -0.7498604124941119498, 0.000000000000000000 ) ) ;
#10053=DIRECTION ( 'NONE',  ( -0.4528443260392610581, -0.8915896008669277339, 0.000000000000000000 ) ) ;
#10056=AXIS2_PLACEMENT_3D ( 'NONE', #13018, #13230, #7906 ) ;
#10057=CARTESIAN_POINT ( 'NONE',  ( -18.05918829504999934, 7.130333642789880244, 17.25000000000000000 ) ) ;
#10058=CARTESIAN_POINT ( 'NONE',  ( -1.059188295049996231, -6.027090492554000534, 64.85000000000000853 ) ) ;
#10063=CARTESIAN_POINT ( 'NONE',  ( -5.309188295050000228, -6.027090492554000534, 64.85000000000000853 ) ) ;
#10064=AXIS2_PLACEMENT_3D ( 'NONE', #1653, #9336, #11432 ) ;
#10065=CIRCLE ( 'NONE', #9382, 4.749999999999997335 ) ;
#10067=EDGE_CURVE ( 'NONE', #129, #11446, #149, .T. ) ;
#10071=EDGE_CURVE ( 'NONE', #13343, #2711, #1071, .T. ) ;
#10073=PLANE ( 'NONE',  #929 ) ;
#10074=ORIENTED_EDGE ( 'NONE', *, *, #12496, .T. ) ;
#10078=CIRCLE ( 'NONE', #6261, 6.449999999999997513 ) ;
#10079=CARTESIAN_POINT ( 'NONE',  ( -34.49120980104999035, 19.18892026044596832, 63.36264408499989287 ) ) ;
#10081=DIRECTION ( 'NONE',  ( -1.000000000000000000, 0.000000000000000000, 0.000000000000000000 ) ) ;
#10082=CARTESIAN_POINT ( 'NONE',  ( -18.05918829504999934, 10.97290950744599947, 27.09999999999999787 ) ) ;
#10083=ORIENTED_EDGE ( 'NONE', *, *, #5254, .F. ) ;
#10086=CARTESIAN_POINT ( 'NONE',  ( -16.62028905529726330, 30.31569702815750134, 61.38640438266109101 ) ) ;
#10088=AXIS2_PLACEMENT_3D ( 'NONE', #12343, #11286, #2789 ) ;
#10089=ORIENTED_EDGE ( 'NONE', *, *, #2971, .F. ) ;
#10090=ORIENTED_EDGE ( 'NONE', *, *, #11023, .T. ) ;
#10094=DIRECTION ( 'NONE',  ( 0.000000000000000000, 2.732534507816520408E-15, 1.000000000000000000 ) ) ;
#10096=EDGE_CURVE ( 'NONE', #13375, #12141, #4207, .T. ) ;
#10098=CARTESIAN_POINT ( 'NONE',  ( -14.95720466168106100, 17.08029827338444662, 63.64999999999999858 ) ) ;
#10099=DIRECTION ( 'NONE',  ( 0.000000000000000000, 0.000000000000000000, 1.000000000000000000 ) ) ;
#10102=ORIENTED_EDGE ( 'NONE', *, *, #1810, .F. ) ;
#10107=CARTESIAN_POINT ( 'NONE',  ( -21.17876435844129546, 30.15001770343124221, 59.87185067995086740 ) ) ;
#10108=ORIENTED_EDGE ( 'NONE', *, *, #3550, .T. ) ;
#10109=( GEOMETRIC_REPRESENTATION_CONTEXT ( 3 ) GLOBAL_UNCERTAINTY_ASSIGNED_CONTEXT ( ( #7943 ) ) GLOBAL_UNIT_ASSIGNED_CONTEXT ( ( #9239, #6988, #10153 ) ) REPRESENTATION_CONTEXT ( 'NONE', 'WORKASPACE' ) );
#10110=CYLINDRICAL_SURFACE ( 'NONE', #8990, 6.850000000000002309 ) ;
#10116=ORIENTED_EDGE ( 'NONE', *, *, #9309, .F. ) ;
#10117=EDGE_CURVE ( 'NONE', #129, #11449, #4418, .T. ) ;
#10119=DIRECTION ( 'NONE',  ( 0.3132098788326420080, 0.9496839325805410681, 0.000000000000000000 ) ) ;
#10120=CARTESIAN_POINT ( 'NONE',  ( -39.80918829504999934, -6.027090492554000534, 68.85549045786049760 ) ) ;
#10121=EDGE_LOOP ( 'NONE', ( #11703, #10287, #7494 ) ) ;
#10132=DIRECTION ( 'NONE',  ( 1.000000000000000000, 0.000000000000000000, 0.000000000000000000 ) ) ;
#10133=EDGE_CURVE ( 'NONE', #1440, #1848, #4712, .T. ) ;
#10136=CARTESIAN_POINT ( 'NONE',  ( -18.05918829504999934, 10.97290950744599947, 17.25000000000000000 ) ) ;
#10141=DIRECTION ( 'NONE',  ( 0.000000000000000000, 0.000000000000000000, -1.000000000000000000 ) ) ;
#10142=CARTESIAN_POINT ( 'NONE',  ( -34.21925492805003444, 19.05294282444601706, 63.34900083300006202 ) ) ;
#10143=DIRECTION ( 'NONE',  ( 0.000000000000000000, 0.000000000000000000, -1.000000000000000000 ) ) ;
#10144=EDGE_CURVE ( 'NONE', #7594, #11171, #10899, .T. ) ;
#10145=CARTESIAN_POINT ( 'NONE',  ( -18.05918829504999934, 10.97290950744599947, 24.10000000000000142 ) ) ;
#10146=EDGE_CURVE ( 'NONE', #4307, #8435, #1525, .T. ) ;
#10149=ADVANCED_FACE ( 'NONE', ( #10014 ), #6729, .T. ) ;
#10150=DIRECTION ( 'NONE',  ( 0.000000000000000000, 0.000000000000000000, 1.000000000000000000 ) ) ;
#10151=VERTEX_POINT ( 'NONE', #370 ) ;
#10153=( NAMED_UNIT ( * ) SI_UNIT ( $, .STERADIAN. ) SOLID_ANGLE_UNIT ( ) );
#10154=VERTEX_POINT ( 'NONE', #5730 ) ;
#10157=DIRECTION ( 'NONE',  ( 1.000000000000000000, 0.000000000000000000, 0.000000000000000000 ) ) ;
#10159=DIRECTION ( 'NONE',  ( -0.000000000000000000, -0.000000000000000000, -1.000000000000000000 ) ) ;
#10161=EDGE_CURVE ( 'NONE', #6357, #129, #10670, .T. ) ;
#10163=CIRCLE ( 'NONE', #101, 17.00000000000000355 ) ;
#10164=EDGE_CURVE ( 'NONE', #2082, #8965, #10439, .T. ) ;
#10169=LINE ( 'NONE', #4850, #12640 ) ;
#10171=CARTESIAN_POINT ( 'NONE',  ( -13.53074503465739831, 19.88880551611529768, 62.85000000000000142 ) ) ;
#10172=TOROIDAL_SURFACE ( 'NONE', #3480, 16.66282263685194920, 1.000000000000000000 ) ;
#10173=CARTESIAN_POINT ( 'NONE',  ( -20.88744887221551494, 30.18746625240332904, 60.27899883312479545 ) ) ;
#10175=DIRECTION ( 'NONE',  ( -1.000000000000000000, 0.000000000000000000, 0.000000000000000000 ) ) ;
#10176=DIRECTION ( 'NONE',  ( 0.000000000000000000, 0.000000000000000000, -1.000000000000000000 ) ) ;
#10180=VECTOR ( 'NONE', #11151, 999.9999999999998863 ) ;
#10183=CARTESIAN_POINT ( 'NONE',  ( -10.78334210919089919, -7.245613863947189870, 7.250000000000000000 ) ) ;
#10184=PLANE ( 'NONE',  #4913 ) ;
#10186=DIRECTION ( 'NONE',  ( -1.000000000000000000, 0.000000000000000000, 0.000000000000000000 ) ) ;
#10188=LINE ( 'NONE', #605, #8199 ) ;
#10190=CARTESIAN_POINT ( 'NONE',  ( -10.78334210919089919, 29.19143287883919768, 7.250000000000000000 ) ) ;
#10192=CARTESIAN_POINT ( 'NONE',  ( -18.05918829309690210, 18.59099508048574734, 61.65955166400529919 ) ) ;
#10193=CARTESIAN_POINT ( 'NONE',  ( -1.059188295049996231, -6.027090492554000534, 64.35000000000000853 ) ) ;
#10197=UNCERTAINTY_MEASURE_WITH_UNIT (LENGTH_MEASURE( 1.000000000000000082E-05 ), #3271, 'distance_accuracy_value', 'NONE');
#10200=CARTESIAN_POINT ( 'NONE',  ( -11.56214829504999919, 4.475869507446000206, 64.85000000000000853 ) ) ;
#10201=EDGE_CURVE ( 'NONE', #2189, #2730, #4499, .T. ) ;
#10203=VERTEX_POINT ( 'NONE', #4565 ) ;
#10204=ORIENTED_EDGE ( 'NONE', *, *, #6551, .F. ) ;
#10206=FACE_OUTER_BOUND ( 'NONE', #7333, .T. ) ;
#10209=CARTESIAN_POINT ( 'NONE',  ( -30.48673169511680214, 10.97290950744599947, 17.25000000000000000 ) ) ;
#10210=DIRECTION ( 'NONE',  ( 0.000000000000000000, 0.000000000000000000, 1.000000000000000000 ) ) ;
#10211=CONICAL_SURFACE ( 'NONE', #4184, 16.75000000000000355, 0.7853981633974461696 ) ;
#10212=FACE_OUTER_BOUND ( 'NONE', #2208, .T. ) ;
#10213=VERTEX_POINT ( 'NONE', #12037 ) ;
#10214=VERTEX_POINT ( 'NONE', #8818 ) ;
#10215=CARTESIAN_POINT ( 'NONE',  ( -16.07267548837544879, 30.27520963107377838, 61.07113917507989242 ) ) ;
#10216=AXIS2_PLACEMENT_3D ( 'NONE', #1204, #4231, #10515 ) ;
#10217=EDGE_LOOP ( 'NONE', ( #1460, #425, #12639, #3849 ) ) ;
#10219=VERTEX_POINT ( 'NONE', #7834 ) ;
#10221=CARTESIAN_POINT ( 'NONE',  ( 2.262399129208274573, -0.4981161769137525952, 17.25000000000000000 ) ) ;
#10222=LINE ( 'NONE', #639, #6922 ) ;
#10223=ORIENTED_EDGE ( 'NONE', *, *, #4589, .F. ) ;
#10225=DIRECTION ( 'NONE',  ( 0.4528443260392610026, 0.8915896008669278450, 0.000000000000000000 ) ) ;
#10229=DIRECTION ( 'NONE',  ( -1.000000000000000000, 0.000000000000000000, 0.000000000000000000 ) ) ;
#10230=CARTESIAN_POINT ( 'NONE',  ( -17.30244591831155887, 27.95705352479190964, 58.66032464001973779 ) ) ;
#10231=FACE_OUTER_BOUND ( 'NONE', #6312, .T. ) ;
#10232=AXIS2_PLACEMENT_3D ( 'NONE', #12835, #3288, #7502 ) ;
#10233=VECTOR ( 'NONE', #3600, 1000.000000000000114 ) ;
#10234=ORIENTED_EDGE ( 'NONE', *, *, #7727, .T. ) ;
#10235=ORIENTED_EDGE ( 'NONE', *, *, #4395, .T. ) ;
#10237=EDGE_CURVE ( 'NONE', #11902, #7831, #5807, .T. ) ;
#10238=( GEOMETRIC_REPRESENTATION_CONTEXT ( 3 ) GLOBAL_UNCERTAINTY_ASSIGNED_CONTEXT ( ( #1392 ) ) GLOBAL_UNIT_ASSIGNED_CONTEXT ( ( #1947, #8364, #12627 ) ) REPRESENTATION_CONTEXT ( 'NONE', 'WORKASPACE' ) );
#10240=AXIS2_PLACEMENT_3D ( 'NONE', #11791, #8512, #2392 ) ;
#10241=DIRECTION ( 'NONE',  ( 0.000000000000000000, 0.000000000000000000, -1.000000000000000000 ) ) ;
#10242=AXIS2_PLACEMENT_3D ( 'NONE', #4285, #6431, #8 ) ;
#10243=CARTESIAN_POINT ( 'NONE',  ( -18.05918829504999934, 30.36027202460864771, 61.70913974837019822 ) ) ;
#10245=LINE ( 'NONE', #9322, #6070 ) ;
#10246=DIRECTION ( 'NONE',  ( 0.000000000000000000, 0.000000000000000000, 1.000000000000000000 ) ) ;
#10247=CARTESIAN_POINT ( 'NONE',  ( -13.53074503465739831, 19.88880551611529768, 64.85000000000000853 ) ) ;
#10248=EDGE_CURVE ( 'NONE', #6548, #8825, #3554, .T. ) ;
#10249=CARTESIAN_POINT ( 'NONE',  ( -5.809188295050001116, 27.97290950744599769, 68.85549045786049760 ) ) ;
#10253=VECTOR ( 'NONE', #11145, 1000.000000000000000 ) ;
#10254=EDGE_CURVE ( 'NONE', #6577, #9588, #13783, .T. ) ;
#10255=DIRECTION ( 'NONE',  ( 0.000000000000000000, 0.000000000000000000, 1.000000000000000000 ) ) ;
#10256=EDGE_LOOP ( 'NONE', ( #3791, #11223, #3378, #968, #9335 ) ) ;
#10260=CARTESIAN_POINT ( 'NONE',  ( -35.05918829505000645, -6.027090492554000534, 7.250000000000000000 ) ) ;
#10262=DIRECTION ( 'NONE',  ( -0.9496839325805410681, 0.3132098788326420080, 0.000000000000000000 ) ) ;
#10264=CARTESIAN_POINT ( 'NONE',  ( -39.80918829504999934, -6.027090492554000534, 7.250000000000000000 ) ) ;
#10272=LINE ( 'NONE', #1955, #8378 ) ;
#10273=EDGE_LOOP ( 'NONE', ( #12016, #271, #13178, #4752, #4826 ) ) ;
#10275=DIRECTION ( 'NONE',  ( 0.000000000000000000, 0.000000000000000000, -1.000000000000000000 ) ) ;
#10277=FACE_OUTER_BOUND ( 'NONE', #5708, .T. ) ;
#10279=DIRECTION ( 'NONE',  ( 0.000000000000000000, 0.000000000000000000, 1.000000000000000000 ) ) ;
#10280=CARTESIAN_POINT ( 'NONE',  ( -10.82033510625394079, -2.574630058508199593, 62.14999999999999858 ) ) ;
#10281=DIRECTION ( 'NONE',  ( -1.000000000000000000, 0.000000000000000000, 0.000000000000000000 ) ) ;
#10282=CIRCLE ( 'NONE', #10064, 34.69999999999999574 ) ;
#10283=AXIS2_PLACEMENT_3D ( 'NONE', #6075, #10350, #842 ) ;
#10284=TOROIDAL_SURFACE ( 'NONE', #6927, 3.000000000000000888, 2.000000000000000000 ) ;
#10287=ORIENTED_EDGE ( 'NONE', *, *, #4324, .F. ) ;
#10288=CARTESIAN_POINT ( 'NONE',  ( -15.27956492296077329, 30.19337278779117284, 60.33853848387425245 ) ) ;
#10294=ORIENTED_EDGE ( 'NONE', *, *, #5935, .T. ) ;
#10295=DIRECTION ( 'NONE',  ( -1.000000000000000000, 0.000000000000000000, 0.000000000000000000 ) ) ;
#10298=CARTESIAN_POINT ( 'NONE',  ( -18.05918829504999934, 10.97290950744599947, 64.85000000000000853 ) ) ;
#10304=ORIENTED_EDGE ( 'NONE', *, *, #12908, .T. ) ;
#10307=CIRCLE ( 'NONE', #11422, 24.92993838181874722 ) ;
#10308=DIRECTION ( 'NONE',  ( -1.000000000000000000, 0.000000000000000000, 0.000000000000000000 ) ) ;
#10317=EDGE_CURVE ( 'NONE', #12584, #2746, #11351, .T. ) ;
#10321=CARTESIAN_POINT ( 'NONE',  ( -18.05918829504999934, 10.97290950744599947, 60.65000000000000568 ) ) ;
#10322=DIRECTION ( 'NONE',  ( 0.000000000000000000, 0.000000000000000000, -1.000000000000000000 ) ) ;
#10324=FACE_OUTER_BOUND ( 'NONE', #8291, .T. ) ;
#10327=DIRECTION ( 'NONE',  ( 0.000000000000000000, 0.000000000000000000, -1.000000000000000000 ) ) ;
#10328=AXIS2_PLACEMENT_3D ( 'NONE', #8069, #13576, #7007 ) ;
#10330=EDGE_CURVE ( 'NONE', #1108, #2279, #8228, .T. ) ;
#10332=EDGE_CURVE ( 'NONE', #12635, #6090, #3111, .T. ) ;
#10334=ORIENTED_EDGE ( 'NONE', *, *, #10936, .T. ) ;
#10335=CARTESIAN_POINT ( 'NONE',  ( -10.25088531517539714, 30.80589556422609832, 5.250000000000000000 ) ) ;
#10336=EDGE_LOOP ( 'NONE', ( #3147, #12798, #2857, #4181, #11695 ) ) ;
#10337=VERTEX_POINT ( 'NONE', #11406 ) ;
#10338=CARTESIAN_POINT ( 'NONE',  ( -19.70293766808219615, 16.19054976041004679, 68.39999137210355684 ) ) ;
#10342=DIRECTION ( 'NONE',  ( 1.000000000000000000, 0.000000000000000000, 0.000000000000000000 ) ) ;
#10344=AXIS2_PLACEMENT_3D ( 'NONE', #4948, #11372, #4119 ) ;
#10347=ORIENTED_EDGE ( 'NONE', *, *, #4853, .T. ) ;
#10348=CARTESIAN_POINT ( 'NONE',  ( -14.87621594265382363, 30.14123926869076442, 54.93378218723427153 ) ) ;
#10349=ORIENTED_EDGE ( 'NONE', *, *, #206, .T. ) ;
#10350=DIRECTION ( 'NONE',  ( 0.000000000000000000, 0.000000000000000000, -1.000000000000000000 ) ) ;
#10353=FACE_OUTER_BOUND ( 'NONE', #9024, .T. ) ;
#10355=CYLINDRICAL_SURFACE ( 'NONE', #2272, 3.449999999999999734 ) ;
#10356=CYLINDRICAL_SURFACE ( 'NONE', #6327, 16.00000000000000355 ) ;
#10360=VERTEX_POINT ( 'NONE', #576 ) ;
#10361=ORIENTED_EDGE ( 'NONE', *, *, #4934, .T. ) ;
#10362=ORIENTED_EDGE ( 'NONE', *, *, #8744, .T. ) ;
#10363=EDGE_CURVE ( 'NONE', #7637, #8318, #2905, .T. ) ;
#10364=ADVANCED_FACE ( 'NONE', ( #12523 ), #6079, .T. ) ;
#10365=DIRECTION ( 'NONE',  ( 0.000000000000000000, 0.000000000000000000, 1.000000000000000000 ) ) ;
#10367=CARTESIAN_POINT ( 'NONE',  ( -19.61493467298536331, 30.30811942209248500, 61.32902609463271659 ) ) ;
#10368=CARTESIAN_POINT ( 'NONE',  ( -18.05918829504999934, 10.97290950744599947, 61.85000000000000142 ) ) ;
#10369=EDGE_CURVE ( 'NONE', #9632, #9965, #641, .T. ) ;
#10371=CYLINDRICAL_SURFACE ( 'NONE', #2745, 17.00000000000000000 ) ;
#10373=CARTESIAN_POINT ( 'NONE',  ( -20.04397650943645459, 13.22249074492834175, 27.09999999999999787 ) ) ;
#10376=CIRCLE ( 'NONE', #113, 12.00000000000000355 ) ;
#10377=CARTESIAN_POINT ( 'NONE',  ( -18.05918829504999934, 10.97290950744599947, 60.65000000000000568 ) ) ;
#10378=ORIENTED_EDGE ( 'NONE', *, *, #4279, .T. ) ;
#10380=DIRECTION ( 'NONE',  ( 0.000000000000000000, 0.000000000000000000, 1.000000000000000000 ) ) ;
#10381=ADVANCED_FACE ( 'NONE', ( #1692 ), #11203, .T. ) ;
#10384=CARTESIAN_POINT ( 'NONE',  ( -22.69945727585292872, 13.54674356991320394, 68.54372738201359994 ) ) ;
#10386=PLANE ( 'NONE',  #9349 ) ;
#10388=ADVANCED_FACE ( 'NONE', ( #11470, #3871 ), #5036, .F. ) ;
#10389=DIRECTION ( 'NONE',  ( 0.000000000000000000, 0.000000000000000000, -1.000000000000000000 ) ) ;
#10390=FILL_AREA_STYLE ('',( #814 ) ) ;
#10396=ORIENTED_EDGE ( 'NONE', *, *, #6939, .F. ) ;
#10398=VERTEX_POINT ( 'NONE', #9091 ) ;
#10403=CARTESIAN_POINT ( 'NONE',  ( -11.06274345774342116, 24.74796884084004844, 58.54999999999999716 ) ) ;
#10405=DIRECTION ( 'NONE',  ( -1.000000000000000000, 0.000000000000000000, 0.000000000000000000 ) ) ;
#10407=AXIS2_PLACEMENT_3D ( 'NONE', #11313, #12638, #4959 ) ;
#10408=ORIENTED_EDGE ( 'NONE', *, *, #12167, .F. ) ;
#10409=CARTESIAN_POINT ( 'NONE',  ( -14.97129325674108991, 30.15419697592694348, 59.91884240419840069 ) ) ;
#10410=ORIENTED_EDGE ( 'NONE', *, *, #6699, .F. ) ;
#10415=CYLINDRICAL_SURFACE ( 'NONE', #9405, 6.299999999999999822 ) ;
#10417=CARTESIAN_POINT ( 'NONE',  ( -18.05918829504999934, 14.81548537210212046, 17.25000000000000000 ) ) ;
#10422=DIRECTION ( 'NONE',  ( 0.000000000000000000, 0.000000000000000000, 1.000000000000000000 ) ) ;
#10423=ADVANCED_FACE ( 'NONE', ( #9510 ), #1047, .F. ) ;
#10424=CARTESIAN_POINT ( 'NONE',  ( -25.86749127492459976, 30.80589556422609832, 17.25000000000000000 ) ) ;
#10425=VERTEX_POINT ( 'NONE', #11739 ) ;
#10426=VERTEX_POINT ( 'NONE', #7326 ) ;
#10427=AXIS2_PLACEMENT_3D ( 'NONE', #6176, #7478, #7354 ) ;
#10428=VERTEX_POINT ( 'NONE', #9451 ) ;
#10429=EDGE_LOOP ( 'NONE', ( #4774, #2624, #1489 ) ) ;
#10430=ORIENTED_EDGE ( 'NONE', *, *, #8634, .F. ) ;
#10433=CARTESIAN_POINT ( 'NONE',  ( -19.73609606983273324, 30.29966228794214089, 61.26430342259844508 ) ) ;
#10435=CARTESIAN_POINT ( 'NONE',  ( -19.55918829504999934, 21.47290950744600124, 57.35000000000000142 ) ) ;
#10437=CARTESIAN_POINT ( 'NONE',  ( -16.55918829504999579, 21.47290950744600124, 57.35000000000000142 ) ) ;
#10438=DIRECTION ( 'NONE',  ( 0.000000000000000000, 0.000000000000000000, 1.000000000000000000 ) ) ;
#10439=CIRCLE ( 'NONE', #9332, 0.9499999999999995115 ) ;
#10447=CIRCLE ( 'NONE', #12234, 2.700000000000001066 ) ;
#10448=CIRCLE ( 'NONE', #4432, 4.750000000000000000 ) ;
#10449=DIRECTION ( 'NONE',  ( 0.000000000000000000, 0.000000000000000000, -1.000000000000000000 ) ) ;
#10450=DIRECTION ( 'NONE',  ( 0.3132098788326367900, -0.9496839325805428444, 0.000000000000000000 ) ) ;
#10451=VERTEX_POINT ( 'NONE', #1984 ) ;
#10453=DIRECTION ( 'NONE',  ( 0.000000000000000000, 0.000000000000000000, 1.000000000000000000 ) ) ;
#10455=DIRECTION ( 'NONE',  ( 0.000000000000000000, 0.000000000000000000, 1.000000000000000000 ) ) ;
#10457=DIRECTION ( 'NONE',  ( 0.000000000000000000, 0.000000000000000000, -1.000000000000000000 ) ) ;
#10458=CARTESIAN_POINT ( 'NONE',  ( -40.33164489498318517, 10.97290950744599947, 5.250000000000000000 ) ) ;
#10462=AXIS2_PLACEMENT_3D ( 'NONE', #9577, #3240, #11952 ) ;
#10464=EDGE_CURVE ( 'NONE', #9989, #1735, #10907, .T. ) ;
#10471=ORIENTED_EDGE ( 'NONE', *, *, #9722, .T. ) ;
#10472=EDGE_LOOP ( 'NONE', ( #11088, #5983, #3704, #10961 ) ) ;
#10473=CARTESIAN_POINT ( 'NONE',  ( -1.059188295049996231, 27.97290950744599769, 64.85000000000000853 ) ) ;
#10475=ADVANCED_FACE ( 'NONE', ( #2191 ), #11607, .T. ) ;
#10478=CARTESIAN_POINT ( 'NONE',  ( -18.05918829504999934, 10.97290950744599947, 64.85000000000000853 ) ) ;
#10479=EDGE_CURVE ( 'NONE', #2105, #5663, #12791, .T. ) ;
#10481=ORIENTED_EDGE ( 'NONE', *, *, #10598, .T. ) ;
#10482=CARTESIAN_POINT ( 'NONE',  ( -14.82082868479300508, 30.13344396834445860, 59.66657486885861772 ) ) ;
#10485=CARTESIAN_POINT ( 'NONE',  ( -18.05918829504999934, 10.97290950744599947, 57.35000000000000142 ) ) ;
#10490=DIRECTION ( 'NONE',  ( 0.4528443260392608360, 0.8915896008669277339, 0.000000000000000000 ) ) ;
#10491=DIRECTION ( 'NONE',  ( -0.4678190685372728419, 0.5302313826179317902, 0.7071067811865437980 ) ) ;
#10493=DIRECTION ( 'NONE',  ( 0.000000000000000000, -1.000000000000000000, 3.387121092260456770E-15 ) ) ;
#10495=VECTOR ( 'NONE', #4961, 1000.000000000000114 ) ;
#10496=FACE_OUTER_BOUND ( 'NONE', #13008, .T. ) ;
#10497=CARTESIAN_POINT ( 'NONE',  ( -16.85849676537586461, 27.93104124342158912, 58.27085874777026930 ) ) ;
#10500=ADVANCED_FACE ( 'NONE', ( #2123, #6365 ), #5377, .F. ) ;
#10501=ORIENTED_EDGE ( 'NONE', *, *, #5149, .T. ) ;
#10503=( BOUNDED_CURVE ( )  B_SPLINE_CURVE ( 3, ( #11402, #12381, #9240, #3868 ),
 .UNSPECIFIED., .F., .F. ) 
 B_SPLINE_CURVE_WITH_KNOTS ( ( 4, 4 ),
 ( 0.04873315200000170183, 0.9512668479999960569 ),
 .UNSPECIFIED. ) 
 CURVE ( )  GEOMETRIC_REPRESENTATION_ITEM ( )  RATIONAL_B_SPLINE_CURVE ( ( 0.9230982619916300314, 0.4726811441755540133, 0.4726811441755530141, 0.9230982619916260346 ) ) 
 REPRESENTATION_ITEM ( '' )  );
#10505=AXIS2_PLACEMENT_3D ( 'NONE', #12851, #7522, #1911 ) ;
#10506=EDGE_LOOP ( 'NONE', ( #11781, #13417, #5322, #13279 ) ) ;
#10507=VERTEX_POINT ( 'NONE', #993 ) ;
#10509=ORIENTED_EDGE ( 'NONE', *, *, #8081, .F. ) ;
#10511=PLANE ( 'NONE',  #11112 ) ;
#10513=DIRECTION ( 'NONE',  ( 0.000000000000000000, 0.000000000000000000, -1.000000000000000000 ) ) ;
#10515=DIRECTION ( 'NONE',  ( -1.000000000000000000, 0.000000000000000000, 0.000000000000000000 ) ) ;
#10518=AXIS2_PLACEMENT_3D ( 'NONE', #6362, #6565, #8659 ) ;
#10519=VECTOR ( 'NONE', #1004, 1000.000000000000000 ) ;
#10521=CIRCLE ( 'NONE', #8495, 6.449999999999997513 ) ;
#10522=ORIENTED_EDGE ( 'NONE', *, *, #1528, .F. ) ;
#10523=ORIENTED_EDGE ( 'NONE', *, *, #1051, .T. ) ;
#10525=AXIS2_PLACEMENT_3D ( 'NONE', #13080, #1558, #9888 ) ;
#10528=ORIENTED_EDGE ( 'NONE', *, *, #11052, .T. ) ;
#10529=DIRECTION ( 'NONE',  ( 1.000000000000000000, 0.000000000000000000, 0.000000000000000000 ) ) ;
#10531=CARTESIAN_POINT ( 'NONE',  ( -1.059188295049996231, 27.97290950744599769, 64.35000000000000853 ) ) ;
#10532=CARTESIAN_POINT ( 'NONE',  ( -16.20671929495594910, 8.873300352462479168, 23.90000000000000213 ) ) ;
#10534=DIRECTION ( 'NONE',  ( -0.4528443260392610581, -0.8915896008669277339, 0.000000000000000000 ) ) ;
#10535=DIRECTION ( 'NONE',  ( 0.000000000000000000, 0.000000000000000000, -1.000000000000000000 ) ) ;
#10536=EDGE_CURVE ( 'NONE', #10337, #5356, #633, .T. ) ;
#10537=CARTESIAN_POINT ( 'NONE',  ( -1.059188295049996231, -6.027090492554000534, 58.85000000000000142 ) ) ;
#10539=CARTESIAN_POINT ( 'NONE',  ( -28.87730642030694739, -7.867426463707978712, 5.250000000000000000 ) ) ;
#10542=DIRECTION ( 'NONE',  ( 0.000000000000000000, 0.000000000000000000, -1.000000000000000000 ) ) ;
#10546=VECTOR ( 'NONE', #808, 1000.000000000000000 ) ;
#10547=DIRECTION ( 'NONE',  ( -0.000000000000000000, -0.000000000000000000, 1.000000000000000000 ) ) ;
#10549=EDGE_CURVE ( 'NONE', #11675, #4278, #8456, .T. ) ;
#10551=ADVANCED_FACE ( 'NONE', ( #921 ), #5180, .T. ) ;
#10552=DIRECTION ( 'NONE',  ( 0.000000000000000000, 0.000000000000000000, 1.000000000000000000 ) ) ;
#10553=EDGE_CURVE ( 'NONE', #10426, #7735, #9001, .T. ) ;
#10554=CIRCLE ( 'NONE', #10328, 8.300000000000000711 ) ;
#10555=CARTESIAN_POINT ( 'NONE',  ( -14.82335591628575777, 30.13379967402607562, 59.67111322632907644 ) ) ;
#10556=ORIENTED_EDGE ( 'NONE', *, *, #2714, .T. ) ;
#10559=CARTESIAN_POINT ( 'NONE',  ( -12.62505638257885998, 21.67198471784914915, 57.35000000000000142 ) ) ;
#10561=CARTESIAN_POINT ( 'NONE',  ( -21.05918829505000289, 10.97290950744599947, 118.8499999999999943 ) ) ;
#10563=DIRECTION ( 'NONE',  ( 0.000000000000000000, 0.000000000000000000, -1.000000000000000000 ) ) ;
#10564=EDGE_CURVE ( 'NONE', #2075, #1834, #10448, .T. ) ;
#10565=VECTOR ( 'NONE', #4336, 1000.000000000000000 ) ;
#10566=CARTESIAN_POINT ( 'NONE',  ( -11.63918829504999941, 10.97290950744599947, 64.85000000000000853 ) ) ;
#10567=DIRECTION ( 'NONE',  ( 0.000000000000000000, 0.000000000000000000, 1.000000000000000000 ) ) ;
#10568=EDGE_CURVE ( 'NONE', #642, #1042, #4216, .T. ) ;
#10569=EDGE_CURVE ( 'NONE', #11868, #2414, #8898, .T. ) ;
#10570=ORIENTED_EDGE ( 'NONE', *, *, #50, .F. ) ;
#10573=EDGE_LOOP ( 'NONE', ( #8557, #4937, #589, #1361, #4310, #11668 ) ) ;
#10574=CARTESIAN_POINT ( 'NONE',  ( -18.05918829504999934, 10.97290950744599947, 53.85000000000000142 ) ) ;
#10578=CARTESIAN_POINT ( 'NONE',  ( -21.16117192841894834, 4.865520741507539881, 64.54999999999999716 ) ) ;
#10579=DIRECTION ( 'NONE',  ( 1.000000000000000000, 0.000000000000000000, 0.000000000000000000 ) ) ;
#10581=CARTESIAN_POINT ( 'NONE',  ( -11.63918829504999941, 10.97290950744599947, 64.85000000000000853 ) ) ;
#10582=EDGE_CURVE ( 'NONE', #2781, #5561, #9787, .T. ) ;
#10586=ORIENTED_EDGE ( 'NONE', *, *, #11520, .F. ) ;
#10588=FACE_OUTER_BOUND ( 'NONE', #5723, .T. ) ;
#10591=SURFACE_SIDE_STYLE ('',( #6337 ) ) ;
#10597=LINE ( 'NONE', #5416, #7550 ) ;
#10598=EDGE_CURVE ( 'NONE', #1636, #803, #1659, .T. ) ;
#10600=VERTEX_POINT ( 'NONE', #1516 ) ;
#10601=AXIS2_PLACEMENT_3D ( 'NONE', #4769, #5797, #5659 ) ;
#10602=EDGE_LOOP ( 'NONE', ( #9287, #5118, #9329, #9395, #815, #9416 ) ) ;
#10608=CARTESIAN_POINT ( 'NONE',  ( -13.43623923775013651, 8.383794209755873084, 68.55139394072084258 ) ) ;
#10609=CARTESIAN_POINT ( 'NONE',  ( -18.05918829504999934, 10.97290950744599947, 17.25000000000000000 ) ) ;
#10610=DIRECTION ( 'NONE',  ( 0.000000000000000000, 0.000000000000000000, 1.000000000000000000 ) ) ;
#10611=DIRECTION ( 'NONE',  ( 0.000000000000000000, -1.000000000000000000, 0.000000000000000000 ) ) ;
#10614=UNCERTAINTY_MEASURE_WITH_UNIT (LENGTH_MEASURE( 1.000000000000000082E-05 ), #5489, 'distance_accuracy_value', 'NONE');
#10616=ORIENTED_EDGE ( 'NONE', *, *, #7451, .F. ) ;
#10617=EDGE_CURVE ( 'NONE', #1687, #2014, #13342, .T. ) ;
#10619=CARTESIAN_POINT ( 'NONE',  ( -16.50344191708178343, 30.30811942209297882, 53.37097390537915942 ) ) ;
#10622=DIRECTION ( 'NONE',  ( 0.000000000000000000, 0.000000000000000000, -1.000000000000000000 ) ) ;
#10623=DIRECTION ( 'NONE',  ( 1.000000000000000000, 0.000000000000000000, 0.000000000000000000 ) ) ;
#10628=DIRECTION ( 'NONE',  ( 1.000000000000000000, 0.000000000000000000, 0.000000000000000000 ) ) ;
#10629=CIRCLE ( 'NONE', #8396, 6.345833333000001630 ) ;
#10630=CARTESIAN_POINT ( 'NONE',  ( -18.05918829504999934, 10.97290950744599947, 27.30000000000000071 ) ) ;
#10631=ORIENTED_EDGE ( 'NONE', *, *, #2732, .T. ) ;
#10633=CARTESIAN_POINT ( 'NONE',  ( -18.05918829504999934, 10.97290950744599947, 61.72253826518770836 ) ) ;
#10634=ORIENTED_EDGE ( 'NONE', *, *, #9810, .T. ) ;
#10636=ORIENTED_EDGE ( 'NONE', *, *, #12852, .F. ) ;
#10638=ORIENTED_EDGE ( 'NONE', *, *, #8061, .F. ) ;
#10641=EDGE_CURVE ( 'NONE', #7297, #12897, #3529, .T. ) ;
#10643=DIRECTION ( 'NONE',  ( -1.000000000000000000, 0.000000000000000000, 0.000000000000000000 ) ) ;
#10646=DIRECTION ( 'NONE',  ( -0.6615960714621568206, 0.7498604124941127269, 0.000000000000000000 ) ) ;
#10647=DIRECTION ( 'NONE',  ( -1.000000000000000000, 0.000000000000000000, 0.000000000000000000 ) ) ;
#10648=CONICAL_SURFACE ( 'NONE', #12875, 5.500000000000002665, 0.7853981633974433940 ) ;
#10653=AXIS2_PLACEMENT_3D ( 'NONE', #11285, #12342, #4993 ) ;
#10657=CARTESIAN_POINT ( 'NONE',  ( -24.37001676333060018, -4.028726038184999858, 62.14999999999999858 ) ) ;
#10659=CARTESIAN_POINT ( 'NONE',  ( -20.28116495117919271, 30.25376030680740769, 53.80727490026070825 ) ) ;
#10661=DIRECTION ( 'NONE',  ( 0.000000000000000000, 0.000000000000000000, 1.000000000000000000 ) ) ;
#10662=CARTESIAN_POINT ( 'NONE',  ( -22.58763155544259860, 2.057013498776719906, 64.85000000000000853 ) ) ;
#10665=ORIENTED_EDGE ( 'NONE', *, *, #6939, .T. ) ;
#10666=CIRCLE ( 'NONE', #4649, 17.66282263685195275 ) ;
#10668=AXIS2_PLACEMENT_3D ( 'NONE', #6692, #5568, #9858 ) ;
#10670=CIRCLE ( 'NONE', #4867, 1.500000000000001332 ) ;
#10672=ORIENTED_EDGE ( 'NONE', *, *, #3227, .F. ) ;
#10673=DIRECTION ( 'NONE',  ( -1.000000000000000000, 0.000000000000000000, 0.000000000000000000 ) ) ;
#10675=ORIENTED_EDGE ( 'NONE', *, *, #2542, .T. ) ;
#10676=EDGE_LOOP ( 'NONE', ( #2932, #5537, #1396, #723, #9204 ) ) ;
#10677=DIRECTION ( 'NONE',  ( 0.000000000000000000, 0.000000000000000000, 1.000000000000000000 ) ) ;
#10678=EDGE_CURVE ( 'NONE', #3389, #10425, #2737, .T. ) ;
#10680=ORIENTED_EDGE ( 'NONE', *, *, #12457, .T. ) ;
#10681=DIRECTION ( 'NONE',  ( -1.000000000000000000, 0.000000000000000000, 0.000000000000000000 ) ) ;
#10682=ORIENTED_EDGE ( 'NONE', *, *, #2034, .T. ) ;
#10686=AXIS2_PLACEMENT_3D ( 'NONE', #8590, #10563, #12846 ) ;
#10687=CARTESIAN_POINT ( 'NONE',  ( -28.87730642030695094, 29.81324547859994922, 17.25000000000000000 ) ) ;
#10691=CARTESIAN_POINT ( 'NONE',  ( -15.48247209720144113, 30.21696533453561173, 54.13423996167696828 ) ) ;
#10694=CARTESIAN_POINT ( 'NONE',  ( -7.241070169793076161, -7.867426463707975159, 17.25000000000000000 ) ) ;
#10695=DIRECTION ( 'NONE',  ( 0.000000000000000000, 0.000000000000000000, -1.000000000000000000 ) ) ;
#10696=LINE ( 'NONE', #4348, #12080 ) ;
#10701=DIRECTION ( 'NONE',  ( 0.000000000000000000, 0.000000000000000000, -1.000000000000000000 ) ) ;
#10702=AXIS2_PLACEMENT_3D ( 'NONE', #9385, #13496, #3938 ) ;
#10704=VERTEX_POINT ( 'NONE', #7360 ) ;
#10705=ORIENTED_EDGE ( 'NONE', *, *, #6820, .F. ) ;
#10707=VERTEX_POINT ( 'NONE', #9274 ) ;
#10713=CARTESIAN_POINT ( 'NONE',  ( -22.71804201037815218, -4.525318844826149878, 62.14999999999999858 ) ) ;
#10715=ORIENTED_EDGE ( 'NONE', *, *, #7658, .F. ) ;
#10716=DIRECTION ( 'NONE',  ( 0.000000000000000000, 1.000000000000000000, 0.000000000000000000 ) ) ;
#10717=CARTESIAN_POINT ( 'NONE',  ( -19.46048213834016494, 26.91143339763804221, 56.81345751610173522 ) ) ;
#10718=CARTESIAN_POINT ( 'NONE',  ( -13.05918829504999756, 10.97290950744599947, 68.84999999999999432 ) ) ;
#10719=DIRECTION ( 'NONE',  ( 0.000000000000000000, 0.000000000000000000, -1.000000000000000000 ) ) ;
#10720=ADVANCED_FACE ( 'NONE', ( #8149 ), #13726, .F. ) ;
#10722=VERTEX_POINT ( 'NONE', #12560 ) ;
#10723=AXIS2_PLACEMENT_3D ( 'NONE', #9915, #9205, #2862 ) ;
#10725=VECTOR ( 'NONE', #9092, 1000.000000000000000 ) ;
#10726=ORIENTED_EDGE ( 'NONE', *, *, #13277, .T. ) ;
#10727=CARTESIAN_POINT ( 'NONE',  ( -10.47404583389237942, 25.90703532196704728, 61.85000000000000142 ) ) ;
#10730=DIRECTION ( 'NONE',  ( 0.000000000000000000, 0.000000000000000000, -1.000000000000000000 ) ) ;
#10731=CARTESIAN_POINT ( 'NONE',  ( -18.52354985390699937, 30.35570588519016155, 53.02278649370575181 ) ) ;
#10734=ORIENTED_EDGE ( 'NONE', *, *, #5610, .F. ) ;
#10735=FACE_OUTER_BOUND ( 'NONE', #4203, .T. ) ;
#10736=AXIS2_PLACEMENT_3D ( 'NONE', #5475, #5343, #10953 ) ;
#10738=FACE_OUTER_BOUND ( 'NONE', #3345, .T. ) ;
#10750=VERTEX_POINT ( 'NONE', #1806 ) ;
#10753=CARTESIAN_POINT ( 'NONE',  ( -18.05918829504999934, 10.00028003023991907, 62.14999999999999858 ) ) ;
#10756=EDGE_CURVE ( 'NONE', #1633, #7102, #648, .T. ) ;
#10758=DIRECTION ( 'NONE',  ( 0.000000000000000000, 0.000000000000000000, -1.000000000000000000 ) ) ;
#10759=FACE_OUTER_BOUND ( 'NONE', #11605, .T. ) ;
#10760=EDGE_CURVE ( 'NONE', #3796, #8205, #1733, .T. ) ;
#10763=CARTESIAN_POINT ( 'NONE',  ( -15.83390592052727186, 30.25344248475043685, 53.80997457889011315 ) ) ;
#10764=ORIENTED_EDGE ( 'NONE', *, *, #5349, .T. ) ;
#10767=CARTESIAN_POINT ( 'NONE',  ( 2.262399129208279902, 22.44393519180574970, 5.250000000000000000 ) ) ;
#10768=( NAMED_UNIT ( * ) PLANE_ANGLE_UNIT ( ) SI_UNIT ( $, .RADIAN. ) );
#10771=CARTESIAN_POINT ( 'NONE',  ( -1.627166789049998563, 2.756898754446010180, 63.36264408499989287 ) ) ;
#10775=EDGE_CURVE ( 'NONE', #703, #223, #962, .T. ) ;
#10776=ORIENTED_EDGE ( 'NONE', *, *, #11900, .T. ) ;
#10779=CARTESIAN_POINT ( 'NONE',  ( -5.173045190668890569, -15.68519459986890041, 17.25000000000000000 ) ) ;
#10781=VERTEX_POINT ( 'NONE', #11437 ) ;
#10783=CIRCLE ( 'NONE', #11897, 4.250000000000000000 ) ;
#10787=CARTESIAN_POINT ( 'NONE',  ( -18.05918829504999934, 10.97290950744599947, 61.65955166399999854 ) ) ;
#10788=CARTESIAN_POINT ( 'NONE',  ( -17.22489654692306971, 26.95114159751178562, 56.10333731137770741 ) ) ;
#10790=CARTESIAN_POINT ( 'NONE',  ( -18.05918829504999934, 10.97290950744599947, 60.60999999999999943 ) ) ;
#10791=CARTESIAN_POINT ( 'NONE',  ( -18.05918829504999934, 10.97290950744599947, 63.45000000000000284 ) ) ;
#10795=EDGE_CURVE ( 'NONE', #3923, #7555, #5952, .T. ) ;
#10796=ADVANCED_FACE ( 'NONE', ( #7288 ), #5293, .F. ) ;
#10797=ORIENTED_EDGE ( 'NONE', *, *, #10553, .F. ) ;
#10798=VERTEX_POINT ( 'NONE', #5145 ) ;
#10800=DIRECTION ( 'NONE',  ( 0.000000000000000000, 0.000000000000000000, -1.000000000000000000 ) ) ;
#10801=DIRECTION ( 'NONE',  ( -1.000000000000000000, 0.000000000000000000, 0.000000000000000000 ) ) ;
#10803=ORIENTED_EDGE ( 'NONE', *, *, #4424, .F. ) ;
#10806=DIRECTION ( 'NONE',  ( 0.000000000000000000, 0.000000000000000000, -1.000000000000000000 ) ) ;
#10807=EDGE_LOOP ( 'NONE', ( #9143, #11828, #12102, #13621 ) ) ;
#10808=CARTESIAN_POINT ( 'NONE',  ( -18.05918829505001355, 18.58149382944599992, 61.98378871700002435 ) ) ;
#10810=CARTESIAN_POINT ( 'NONE',  ( -18.05918829488915023, 18.13901823688300396, 61.72253826514069175 ) ) ;
#10812=EDGE_CURVE ( 'NONE', #7807, #6311, #2303, .T. ) ;
#10817=CARTESIAN_POINT ( 'NONE',  ( -1.059188295049996231, -6.027090492554000534, 68.85549045786049760 ) ) ;
#10818=ADVANCED_FACE ( 'NONE', ( #12886 ), #7531, .F. ) ;
#10820=LINE ( 'NONE', #7377, #6511 ) ;
#10822=DIRECTION ( 'NONE',  ( 0.000000000000000000, -1.000000000000000000, 2.732534507816519619E-15 ) ) ;
#10823=DIRECTION ( 'NONE',  ( 0.6615960714621565986, -0.7498604124941128379, 0.000000000000000000 ) ) ;
#10824=EDGE_CURVE ( 'NONE', #5798, #9556, #1316, .T. ) ;
#10826=AXIS2_PLACEMENT_3D ( 'NONE', #4823, #3711, #12231 ) ;
#10827=EDGE_CURVE ( 'NONE', #9556, #9938, #8905, .T. ) ;
#10829=CARTESIAN_POINT ( 'NONE',  ( -15.39172992069172174, 30.20666037739588461, 54.23161053768875917 ) ) ;
#10831=CARTESIAN_POINT ( 'NONE',  ( -7.241070169793063727, -7.867426463707971607, 83.57661607529820458 ) ) ;
#10832=CIRCLE ( 'NONE', #8822, 3.449999999999999734 ) ;
#10833=ADVANCED_FACE ( 'NONE', ( #13791 ), #11583, .F. ) ;
#10837=EDGE_LOOP ( 'NONE', ( #9241, #13494, #12461, #8253 ) ) ;
#10839=EDGE_CURVE ( 'NONE', #9550, #5017, #430, .T. ) ;
#10840=CARTESIAN_POINT ( 'NONE',  ( -18.05918829504999934, 10.97290950744599947, 57.54999999999999716 ) ) ;
#10843=VERTEX_POINT ( 'NONE', #9835 ) ;
#10845=ORIENTED_EDGE ( 'NONE', *, *, #8592, .T. ) ;
#10847=VERTEX_POINT ( 'NONE', #7703 ) ;
#10849=EDGE_LOOP ( 'NONE', ( #7971, #9199, #6021, #12700, #3340, #13421, #13347, #3959, #6147 ) ) ;
#10851=ORIENTED_EDGE ( 'NONE', *, *, #12294, .F. ) ;
#10854=VERTEX_POINT ( 'NONE', #2230 ) ;
#10855=VECTOR ( 'NONE', #10988, 1000.000000000000227 ) ;
#10856=EDGE_CURVE ( 'NONE', #10507, #13375, #8558, .T. ) ;
#10857=DIRECTION ( 'NONE',  ( 0.000000000000000000, -1.000000000000000000, 0.000000000000000000 ) ) ;
#10858=CARTESIAN_POINT ( 'NONE',  ( -16.80552491324057485, 26.92504221762977679, 56.52280737812468203 ) ) ;
#10859=CARTESIAN_POINT ( 'NONE',  ( -34.68447646404997897, 2.660265422446006500, 63.26601075299999621 ) ) ;
#10860=DIRECTION ( 'NONE',  ( 0.000000000000000000, 0.000000000000000000, -1.000000000000000000 ) ) ;
#10861=DIRECTION ( 'NONE',  ( 0.000000000000000000, 0.000000000000000000, -1.000000000000000000 ) ) ;
#10864=CIRCLE ( 'NONE', #3508, 2.700000000000000178 ) ;
#10869=ORIENTED_EDGE ( 'NONE', *, *, #9622, .T. ) ;
#10870=DIRECTION ( 'NONE',  ( 0.6615960714621568206, -0.7498604124941127269, 0.000000000000000000 ) ) ;
#10871=DIRECTION ( 'NONE',  ( 0.000000000000000000, 0.000000000000000000, -1.000000000000000000 ) ) ;
#10873=LINE ( 'NONE', #1218, #13671 ) ;
#10874=DIRECTION ( 'NONE',  ( 0.000000000000000000, 0.000000000000000000, 1.000000000000000000 ) ) ;
#10876=CARTESIAN_POINT ( 'NONE',  ( -2.059188295050000228, 10.97290950744599947, 56.84999999999999432 ) ) ;
#10877=CIRCLE ( 'NONE', #4845, 5.000000000000000888 ) ;
#10878=CARTESIAN_POINT ( 'NONE',  ( -25.22529702413155306, 10.97290950744599947, 61.72253826518770836 ) ) ;
#10880=ADVANCED_FACE ( 'NONE', ( #9546 ), #4244, .T. ) ;
#10881=VECTOR ( 'NONE', #1643, 1000.000000000000000 ) ;
#10882=ORIENTED_EDGE ( 'NONE', *, *, #11933, .F. ) ;
#10884=VECTOR ( 'NONE', #10036, 1000.000000000000000 ) ;
#10892=DIRECTION ( 'NONE',  ( -0.6615960714621564875, 0.7498604124941129490, 0.000000000000000000 ) ) ;
#10895=DIRECTION ( 'NONE',  ( -0.4528443260392611136, -0.8915896008669277339, 0.000000000000000000 ) ) ;
#10898=EDGE_CURVE ( 'NONE', #12210, #11722, #11713, .T. ) ;
#10899=CIRCLE ( 'NONE', #2887, 4.250000000000000000 ) ;
#10900=ORIENTED_EDGE ( 'NONE', *, *, #13366, .T. ) ;
#10901=CARTESIAN_POINT ( 'NONE',  ( -17.79660873271074095, 30.36027202460864416, 52.99086025162979752 ) ) ;
#10902=VECTOR ( 'NONE', #4881, 1000.000000000000000 ) ;
#10904=AXIS2_PLACEMENT_3D ( 'NONE', #196, #9704, #7437 ) ;
#10905=VERTEX_POINT ( 'NONE', #4318 ) ;
#10906=DIRECTION ( 'NONE',  ( 1.000000000000000000, 0.000000000000000000, 0.000000000000000000 ) ) ;
#10907=CIRCLE ( 'NONE', #6882, 24.92993838181874722 ) ;
#10912=EDGE_CURVE ( 'NONE', #3167, #13219, #9125, .T. ) ;
#10914=AXIS2_PLACEMENT_3D ( 'NONE', #10790, #7974, #2776 ) ;
#10916=AXIS2_PLACEMENT_3D ( 'NONE', #963, #2231, #12822 ) ;
#10917=AXIS2_PLACEMENT_3D ( 'NONE', #13521, #6112, #8425 ) ;
#10918=ORIENTED_EDGE ( 'NONE', *, *, #2910, .T. ) ;
#10919=ADVANCED_FACE ( 'NONE', ( #10735 ), #7073, .F. ) ;
#10920=VERTEX_POINT ( 'NONE', #11080 ) ;
#10921=DIRECTION ( 'NONE',  ( -0.9496839325805417342, 0.3132098788326399541, 0.000000000000000000 ) ) ;
#10922=EDGE_LOOP ( 'NONE', ( #8811, #9519, #4461, #10102 ) ) ;
#10927=DIRECTION ( 'NONE',  ( 0.000000000000000000, 1.000000000000000000, 0.000000000000000000 ) ) ;
#10928=ORIENTED_EDGE ( 'NONE', *, *, #6645, .T. ) ;
#10931=CARTESIAN_POINT ( 'NONE',  ( -17.19663385324080807, 26.94964292449384402, 56.12280092792923369 ) ) ;
#10932=CIRCLE ( 'NONE', #3807, 24.92993838181874722 ) ;
#10933=CARTESIAN_POINT ( 'NONE',  ( -18.05918829504999934, 10.97290950744599947, 63.45000000000000284 ) ) ;
#10934=AXIS2_PLACEMENT_3D ( 'NONE', #2223, #1213, #3267 ) ;
#10935=CARTESIAN_POINT ( 'NONE',  ( -19.47340185742309870, 26.91028695795525039, 56.84999999999999432 ) ) ;
#10936=EDGE_CURVE ( 'NONE', #7051, #9534, #13101, .T. ) ;
#10938=ORIENTED_EDGE ( 'NONE', *, *, #3227, .T. ) ;
#10941=AXIS2_PLACEMENT_3D ( 'NONE', #11833, #12748, #8613 ) ;
#10943=ORIENTED_EDGE ( 'NONE', *, *, #11700, .T. ) ;
#10944=LINE ( 'NONE', #8039, #6780 ) ;
#10947=LINE ( 'NONE', #12051, #6863 ) ;
#10948=CARTESIAN_POINT ( 'NONE',  ( -21.59115454767725240, 30.09020406746190446, 55.67294371425958843 ) ) ;
#10950=ORIENTED_EDGE ( 'NONE', *, *, #9557, .T. ) ;
#10953=DIRECTION ( 'NONE',  ( -1.000000000000000000, 0.000000000000000000, 0.000000000000000000 ) ) ;
#10954=DIRECTION ( 'NONE',  ( -0.000000000000000000, -0.000000000000000000, -1.000000000000000000 ) ) ;
#10960=EDGE_CURVE ( 'NONE', #7761, #2189, #8836, .T. ) ;
#10961=ORIENTED_EDGE ( 'NONE', *, *, #998, .T. ) ;
#10962=VERTEX_POINT ( 'NONE', #458 ) ;
#10964=( BOUNDED_CURVE ( )  B_SPLINE_CURVE ( 3, ( #9725, #1412, #10008, #3716 ),
 .UNSPECIFIED., .F., .F. ) 
 B_SPLINE_CURVE_WITH_KNOTS ( ( 4, 4 ),
 ( 0.000000000000000000, 1.000000000000000000 ),
 .UNSPECIFIED. ) 
 CURVE ( )  GEOMETRIC_REPRESENTATION_ITEM ( )  RATIONAL_B_SPLINE_CURVE ( ( 0.9565783017328519655, 0.3188594339109505071, 0.3188594339109505071, 0.9565783017328519655 ) ) 
 REPRESENTATION_ITEM ( '' )  );
#10966=AXIS2_PLACEMENT_3D ( 'NONE', #606, #4874, #11096 ) ;
#10967=LINE ( 'NONE', #10120, #3798 ) ;
#10968=AXIS2_PLACEMENT_3D ( 'NONE', #4878, #13463, #1728 ) ;
#10973=CARTESIAN_POINT ( 'NONE',  ( -18.05918829504999934, 10.97290950744599947, 53.85000000000000142 ) ) ;
#10974=CARTESIAN_POINT ( 'NONE',  ( -3.759188295049999518, 27.97290950744599769, 64.85000000000000853 ) ) ;
#10977=CARTESIAN_POINT ( 'NONE',  ( -25.33503448090910126, 29.19143287883919768, 7.250000000000000000 ) ) ;
#10979=DIRECTION ( 'NONE',  ( -1.000000000000000000, 0.000000000000000000, 0.000000000000000000 ) ) ;
#10980=DIRECTION ( 'NONE',  ( 0.000000000000000000, 0.000000000000000000, 1.000000000000000000 ) ) ;
#10981=CIRCLE ( 'NONE', #692, 1.500000000000001332 ) ;
#10982=CIRCLE ( 'NONE', #4936, 4.250000000000000000 ) ;
#10983=AXIS2_PLACEMENT_3D ( 'NONE', #5198, #12545, #12676 ) ;
#10984=DIRECTION ( 'NONE',  ( 1.000000000000000000, 0.000000000000000000, 0.000000000000000000 ) ) ;
#10985=ADVANCED_FACE ( 'NONE', ( #11144 ), #4729, .T. ) ;
#10986=ADVANCED_FACE ( 'NONE', ( #1572 ), #3570, .F. ) ;
#10988=DIRECTION ( 'NONE',  ( -0.9496839325805432885, 0.3132098788326353467, 0.000000000000000000 ) ) ;
#10993=DIRECTION ( 'NONE',  ( -1.000000000000000000, 0.000000000000000000, 0.000000000000000000 ) ) ;
#10994=COLOUR_RGB ( '', 0.66274510, 0.83137255, 0.94901961) ;
#10996=DIRECTION ( 'NONE',  ( -0.7498604124941127269, -0.6615960714621567096, 0.000000000000000000 ) ) ;
#10997=VERTEX_POINT ( 'NONE', #326 ) ;
#11001=CARTESIAN_POINT ( 'NONE',  ( -19.55918829504999934, 27.90660372932210009, 57.35000000000000142 ) ) ;
#11002=DIRECTION ( 'NONE',  ( 0.7498604124941127269, 0.6615960714621567096, 0.000000000000000000 ) ) ;
#11006=CARTESIAN_POINT ( 'NONE',  ( -30.30918829504999934, 27.97290950744599769, 7.250000000000000000 ) ) ;
#11011=AXIS2_PLACEMENT_3D ( 'NONE', #6931, #7061, #10229 ) ;
#11014=VERTEX_POINT ( 'NONE', #7780 ) ;
#11015=DIRECTION ( 'NONE',  ( 0.000000000000000000, 0.000000000000000000, 1.000000000000000000 ) ) ;
#11017=ADVANCED_FACE ( 'NONE', ( #12054 ), #11020, .T. ) ;
#11018=CARTESIAN_POINT ( 'NONE',  ( -21.62262619219993454, 30.08533272846090512, 55.76115953722869989 ) ) ;
#11019=DIRECTION ( 'NONE',  ( 0.000000000000000000, 0.000000000000000000, -1.000000000000000000 ) ) ;
#11020=CYLINDRICAL_SURFACE ( 'NONE', #12674, 6.449999999999997513 ) ;
#11021=LINE ( 'NONE', #5753, #13798 ) ;
#11022=FACE_OUTER_BOUND ( 'NONE', #8679, .T. ) ;
#11023=EDGE_CURVE ( 'NONE', #12924, #2075, #5680, .T. ) ;
#11024=AXIS2_PLACEMENT_3D ( 'NONE', #611, #10389, #813 ) ;
#11026=EDGE_LOOP ( 'NONE', ( #2068, #1850, #11244, #8615 ) ) ;
#11027=ORIENTED_EDGE ( 'NONE', *, *, #2178, .T. ) ;
#11028=CARTESIAN_POINT ( 'NONE',  ( -1.059188295049996231, 27.97290950744599769, 83.57661607529820458 ) ) ;
#11031=DIRECTION ( 'NONE',  ( 0.000000000000000000, 0.000000000000000000, 1.000000000000000000 ) ) ;
#11032=DIRECTION ( 'NONE',  ( 0.000000000000000000, 0.000000000000000000, 1.000000000000000000 ) ) ;
#11033=DIRECTION ( 'NONE',  ( 0.000000000000000000, -1.000000000000000000, 0.000000000000000000 ) ) ;
#11034=CARTESIAN_POINT ( 'NONE',  ( -40.33164489498318517, 10.97290950744599947, 83.57661607529820458 ) ) ;
#11037=DIRECTION ( 'NONE',  ( 0.000000000000000000, 0.000000000000000000, -1.000000000000000000 ) ) ;
#11038=EDGE_CURVE ( 'NONE', #8205, #3796, #2883, .T. ) ;
#11039=DIRECTION ( 'NONE',  ( 0.4528443260392610026, 0.8915896008669278450, 0.000000000000000000 ) ) ;
#11042=EDGE_LOOP ( 'NONE', ( #2772, #12859, #9846, #3832 ) ) ;
#11043=DIRECTION ( 'NONE',  ( 0.000000000000000000, 1.000000000000000000, 0.000000000000000000 ) ) ;
#11044=EDGE_LOOP ( 'NONE', ( #3150, #10089, #4438, #567 ) ) ;
#11045=VERTEX_POINT ( 'NONE', #8997 ) ;
#11046=CARTESIAN_POINT ( 'NONE',  ( -3.759188295049999518, -6.027090492554000534, 58.85000000000000142 ) ) ;
#11048=CARTESIAN_POINT ( 'NONE',  ( -21.69796668809184936, 15.09714177616359798, 30.59999999999999787 ) ) ;
#11049=AXIS2_PLACEMENT_3D ( 'NONE', #4356, #219, #9804 ) ;
#11050=CARTESIAN_POINT ( 'NONE',  ( -1.461186629049982422, 2.673908674445990119, 63.13003331700004850 ) ) ;
#11052=EDGE_CURVE ( 'NONE', #6829, #7790, #12144, .T. ) ;
#11055=EDGE_CURVE ( 'NONE', #1279, #2935, #4650, .T. ) ;
#11056=AXIS2_PLACEMENT_3D ( 'NONE', #2674, #9067, #1397 ) ;
#11057=DIRECTION ( 'NONE',  ( -1.000000000000000000, 0.000000000000000000, 0.000000000000000000 ) ) ;
#11061=ORIENTED_EDGE ( 'NONE', *, *, #13497, .T. ) ;
#11062=CARTESIAN_POINT ( 'NONE',  ( -18.05918829504999934, 10.97290950744599947, 68.84999999999999432 ) ) ;
#11063=CARTESIAN_POINT ( 'NONE',  ( -18.05918829504999934, 28.64232754551664684, 57.35000000000000142 ) ) ;
#11066=CARTESIAN_POINT ( 'NONE',  ( -25.86749127492459976, 30.80589556422609832, 17.25000000000000000 ) ) ;
#11067=DIRECTION ( 'NONE',  ( 1.000000000000000000, 0.000000000000000000, 0.000000000000000000 ) ) ;
#11078=CARTESIAN_POINT ( 'NONE',  ( -20.85091026108096557, 30.19191053445972628, 60.32389291502525452 ) ) ;
#11079=CYLINDRICAL_SURFACE ( 'NONE', #12097, 4.750000000000000888 ) ;
#11080=CARTESIAN_POINT ( 'NONE',  ( -25.86749127492460332, 30.80589556422609832, 17.25000000000000000 ) ) ;
#11085=ORIENTED_EDGE ( 'NONE', *, *, #1854, .F. ) ;
#11088=ORIENTED_EDGE ( 'NONE', *, *, #6323, .F. ) ;
#11090=EDGE_CURVE ( 'NONE', #1604, #8398, #168, .T. ) ;
#11094=PRESENTATION_STYLE_ASSIGNMENT (( #6957 ) ) ;
#11096=DIRECTION ( 'NONE',  ( -1.000000000000000000, 0.000000000000000000, 0.000000000000000000 ) ) ;
#11099=DIRECTION ( 'NONE',  ( 0.000000000000000000, 0.000000000000000000, -1.000000000000000000 ) ) ;
#11100=CARTESIAN_POINT ( 'NONE',  ( 2.262399129208274129, 22.44393519180576746, 17.25000000000000000 ) ) ;
#11101=CYLINDRICAL_SURFACE ( 'NONE', #6546, 6.449999999999997513 ) ;
#11102=DIRECTION ( 'NONE',  ( 0.000000000000000000, 0.000000000000000000, 1.000000000000000000 ) ) ;
#11104=AXIS2_PLACEMENT_3D ( 'NONE', #5968, #10453, #2863 ) ;
#11106=ORIENTED_EDGE ( 'NONE', *, *, #10536, .T. ) ;
#11108=ORIENTED_EDGE ( 'NONE', *, *, #2393, .T. ) ;
#11109=CARTESIAN_POINT ( 'NONE',  ( -40.33164489498319938, 10.97290950744599947, 17.25000000000000000 ) ) ;
#11112=AXIS2_PLACEMENT_3D ( 'NONE', #11693, #13706, #3835 ) ;
#11113=CARTESIAN_POINT ( 'NONE',  ( -20.57325336660620252, 13.82237907492362083, 27.09999999999999787 ) ) ;
#11114=CIRCLE ( 'NONE', #1734, 8.395833332999997012 ) ;
#11117=CONICAL_SURFACE ( 'NONE', #5088, 5.000000000000000888, 0.7853981633974497223 ) ;
#11121=ORIENTED_EDGE ( 'NONE', *, *, #130, .T. ) ;
#11124=CARTESIAN_POINT ( 'NONE',  ( -16.40830210679616741, 30.30175501171254382, 61.28060770126166545 ) ) ;
#11125=ORIENTED_EDGE ( 'NONE', *, *, #2906, .T. ) ;
#11126=EDGE_LOOP ( 'NONE', ( #6646, #5472, #9803, #11546 ) ) ;
#11128=CARTESIAN_POINT ( 'NONE',  ( -18.05918829505001355, 18.58149382944599992, 61.98378871700002435 ) ) ;
#11129=ADVANCED_FACE ( 'NONE', ( #1590 ), #1287, .T. ) ;
#11131=ORIENTED_EDGE ( 'NONE', *, *, #1969, .T. ) ;
#11132=CARTESIAN_POINT ( 'NONE',  ( -14.08961186627706041, 6.473747032481329988, 64.85000000000000853 ) ) ;
#11133=CARTESIAN_POINT ( 'NONE',  ( -18.05918829504999934, 10.97290950744599947, 64.85000000000000853 ) ) ;
#11134=AXIS2_PLACEMENT_3D ( 'NONE', #2611, #9438, #11519 ) ;
#11135=DIRECTION ( 'NONE',  ( 0.000000000000000000, 0.000000000000000000, -1.000000000000000000 ) ) ;
#11137=LINE ( 'NONE', #1563, #8707 ) ;
#11139=CYLINDRICAL_SURFACE ( 'NONE', #12184, 0.9499999999999995115 ) ;
#11142=CARTESIAN_POINT ( 'NONE',  ( -21.72501355060861528, 30.06926057631531535, 58.60720357358517418 ) ) ;
#11143=CARTESIAN_POINT ( 'NONE',  ( -12.62505638257885998, 21.67198471784914915, 61.85000000000000142 ) ) ;
#11144=FACE_OUTER_BOUND ( 'NONE', #12768, .T. ) ;
#11145=DIRECTION ( 'NONE',  ( 0.000000000000000000, 0.000000000000000000, -1.000000000000000000 ) ) ;
#11149=AXIS2_PLACEMENT_3D ( 'NONE', #12504, #10210, #5024 ) ;
#11151=DIRECTION ( 'NONE',  ( 0.4678190685372678459, -0.5302313826179257950, 0.7071067811865516806 ) ) ;
#11153=CYLINDRICAL_SURFACE ( 'NONE', #5799, 16.95000000000000284 ) ;
#11158=AXIS2_PLACEMENT_3D ( 'NONE', #11028, #8005, #13381 ) ;
#11160=DIRECTION ( 'NONE',  ( 0.6615960714621564875, -0.7498604124941129490, 0.000000000000000000 ) ) ;
#11162=CARTESIAN_POINT ( 'NONE',  ( -7.241070169793063727, -7.867426463707971607, 5.250000000000000000 ) ) ;
#11163=CARTESIAN_POINT ( 'NONE',  ( -20.04397650943645459, 13.22249074492834175, 27.09999999999999787 ) ) ;
#11165=CARTESIAN_POINT ( 'NONE',  ( -18.05918829504999934, 10.97290950744599947, 57.35000000000000142 ) ) ;
#11167=ADVANCED_FACE ( 'NONE', ( #1448 ), #7791, .F. ) ;
#11169=AXIS2_PLACEMENT_3D ( 'NONE', #5187, #11685, #1050 ) ;
#11171=VERTEX_POINT ( 'NONE', #5697 ) ;
#11172=EDGE_LOOP ( 'NONE', ( #12171, #2557, #8751, #9396 ) ) ;
#11173=CARTESIAN_POINT ( 'NONE',  ( -1.059188295049996231, -6.027090492554000534, 64.85000000000000853 ) ) ;
#11180=FACE_OUTER_BOUND ( 'NONE', #10602, .T. ) ;
#11181=AXIS2_PLACEMENT_3D ( 'NONE', #13721, #4171, #12686 ) ;
#11184=VECTOR ( 'NONE', #12695, 1000.000000000000000 ) ;
#11186=EDGE_CURVE ( 'NONE', #13219, #11645, #2652, .T. ) ;
#11187=FACE_OUTER_BOUND ( 'NONE', #7315, .T. ) ;
#11189=EDGE_LOOP ( 'NONE', ( #7317, #4594, #6373, #7901 ) ) ;
#11190=( GEOMETRIC_REPRESENTATION_CONTEXT ( 3 ) GLOBAL_UNCERTAINTY_ASSIGNED_CONTEXT ( ( #1527 ) ) GLOBAL_UNIT_ASSIGNED_CONTEXT ( ( #2265, #10768, #12788 ) ) REPRESENTATION_CONTEXT ( 'NONE', 'WORKASPACE' ) );
#11192=CARTESIAN_POINT ( 'NONE',  ( -16.13055293506123888, 30.28009008632742649, 61.11049587954376960 ) ) ;
#11193=CIRCLE ( 'NONE', #5169, 18.00000000000000000 ) ;
#11195=ORIENTED_EDGE ( 'NONE', *, *, #10824, .T. ) ;
#11196=ORIENTED_EDGE ( 'NONE', *, *, #9908, .T. ) ;
#11197=CARTESIAN_POINT ( 'NONE',  ( -5.631644894983189431, 10.97290950744599947, 83.57661607529820458 ) ) ;
#11198=ORIENTED_EDGE ( 'NONE', *, *, #5254, .T. ) ;
#11199=B_SPLINE_CURVE_WITH_KNOTS ( 'NONE', 3,
 ( #273, #13044, #8570, #11664, #6347, #3223, #12774, #10608, #5286, #9559, #13796, #4266, #8508 ),
 .UNSPECIFIED., .F., .F.,
 ( 4, 1, 1, 1, 1, 1, 2, 2, 4 ),
 ( 0.000000000000000000, 0.2499999999999915623, 0.3749999999999858447, 0.4374999999999851785, 0.4687499999999875100, 0.4843749999999908407, 0.4921874999999919509, 0.4999999999999930056, 1.000000000000000000 ),
 .UNSPECIFIED. ) ;
#11201=ORIENTED_EDGE ( 'NONE', *, *, #12117, .F. ) ;
#11202=CARTESIAN_POINT ( 'NONE',  ( -33.27635693905001801, 3.364325185445997679, 61.98378871700000303 ) ) ;
#11203=CYLINDRICAL_SURFACE ( 'NONE', #10022, 6.449999999999997513 ) ;
#11204=ORIENTED_EDGE ( 'NONE', *, *, #2198, .F. ) ;
#11206=CARTESIAN_POINT ( 'NONE',  ( -32.35918829505000360, 27.97290950744599769, 7.250000000000000000 ) ) ;
#11207=DIRECTION ( 'NONE',  ( 0.000000000000000000, 0.000000000000000000, -1.000000000000000000 ) ) ;
#11209=DIRECTION ( 'NONE',  ( -1.000000000000000000, 0.000000000000000000, 0.000000000000000000 ) ) ;
#11213=ORIENTED_EDGE ( 'NONE', *, *, #2502, .F. ) ;
#11218=CARTESIAN_POINT ( 'NONE',  ( -21.80266211316538616, 30.05678106875573263, 58.27625053142192968 ) ) ;
#11219=DIRECTION ( 'NONE',  ( 1.000000000000000000, 0.000000000000000000, 0.000000000000000000 ) ) ;
#11220=DIRECTION ( 'NONE',  ( -0.7071067811865505703, 8.659560562354931626E-17, 0.7071067811865444641 ) ) ;
#11221=CARTESIAN_POINT ( 'NONE',  ( -18.05918829504999934, 10.97290950744599947, 61.86500000000000199 ) ) ;
#11223=ORIENTED_EDGE ( 'NONE', *, *, #12294, .T. ) ;
#11224=CIRCLE ( 'NONE', #12113, 2.700000000000001066 ) ;
#11225=EDGE_CURVE ( 'NONE', #10360, #1687, #393, .T. ) ;
#11227=LINE ( 'NONE', #7084, #13731 ) ;
#11228=CARTESIAN_POINT ( 'NONE',  ( -18.05918829504999934, 10.00028003023991907, 62.14999999999999858 ) ) ;
#11229=ORIENTED_EDGE ( 'NONE', *, *, #2264, .F. ) ;
#11230=DIRECTION ( 'NONE',  ( -0.9496839325805421783, 0.3132098788326385663, 0.000000000000000000 ) ) ;
#11233=CIRCLE ( 'NONE', #12354, 5.000000000000000888 ) ;
#11234=DIRECTION ( 'NONE',  ( 0.000000000000000000, 0.000000000000000000, -1.000000000000000000 ) ) ;
#11237=DIRECTION ( 'NONE',  ( 0.3202092937642119774, 0.6304490528084099044, -0.7071067811865499042 ) ) ;
#11240=DIRECTION ( 'NONE',  ( 0.000000000000000000, 0.000000000000000000, 1.000000000000000000 ) ) ;
#11241=EDGE_CURVE ( 'NONE', #11264, #11802, #10188, .T. ) ;
#11243=EDGE_CURVE ( 'NONE', #10451, #322, #2196, .T. ) ;
#11244=ORIENTED_EDGE ( 'NONE', *, *, #8576, .T. ) ;
#11245=ORIENTED_EDGE ( 'NONE', *, *, #5603, .F. ) ;
#11247=DIRECTION ( 'NONE',  ( 0.000000000000000000, 0.000000000000000000, 1.000000000000000000 ) ) ;
#11248=EDGE_LOOP ( 'NONE', ( #12187, #8755, #8328, #8921 ) ) ;
#11250=ORIENTED_EDGE ( 'NONE', *, *, #11570, .F. ) ;
#11252=EDGE_CURVE ( 'NONE', #506, #5782, #6375, .T. ) ;
#11254=EDGE_CURVE ( 'NONE', #2443, #2279, #3191, .T. ) ;
#11257=DIRECTION ( 'NONE',  ( -1.000000000000000000, 0.000000000000000000, 0.000000000000000000 ) ) ;
#11263=CARTESIAN_POINT ( 'NONE',  ( -17.79480846713035902, 30.35913048975401551, 61.70128263341860020 ) ) ;
#11264=VERTEX_POINT ( 'NONE', #5192 ) ;
#11265=EDGE_CURVE ( 'NONE', #8057, #12302, #6236, .T. ) ;
#11267=DIRECTION ( 'NONE',  ( 0.000000000000000000, 0.000000000000000000, -1.000000000000000000 ) ) ;
#11268=DIRECTION ( 'NONE',  ( 0.9496839325805432885, -0.3132098788326352912, 0.000000000000000000 ) ) ;
#11270=CARTESIAN_POINT ( 'NONE',  ( -10.47404583389237942, 25.90703532196704728, 60.65000000000000568 ) ) ;
#11272=CARTESIAN_POINT ( 'NONE',  ( -35.05918829505000645, 27.97290950744599769, 68.85549045786049760 ) ) ;
#11274=EDGE_CURVE ( 'NONE', #803, #12773, #4204, .T. ) ;
#11279=ADVANCED_FACE ( 'NONE', ( #9133 ), #10511, .F. ) ;
#11282=CONICAL_SURFACE ( 'NONE', #6803, 4.546599999999997976, 1.029744258676653645 ) ;
#11283=CARTESIAN_POINT ( 'NONE',  ( -20.51961422855616490, 30.22970645148964763, 60.68279484739409924 ) ) ;
#11285=CARTESIAN_POINT ( 'NONE',  ( -35.05918829505000645, 27.97290950744599769, 64.85000000000000853 ) ) ;
#11286=DIRECTION ( 'NONE',  ( 0.000000000000000000, 0.000000000000000000, -1.000000000000000000 ) ) ;
#11289=VECTOR ( 'NONE', #8287, 1000.000000000000000 ) ;
#11290=VERTEX_POINT ( 'NONE', #1001 ) ;
#11293=ORIENTED_EDGE ( 'NONE', *, *, #12890, .F. ) ;
#11294=DIRECTION ( 'NONE',  ( 0.000000000000000000, 0.000000000000000000, 1.000000000000000000 ) ) ;
#11299=DIRECTION ( 'NONE',  ( 0.000000000000000000, 0.000000000000000000, -1.000000000000000000 ) ) ;
#11303=CARTESIAN_POINT ( 'NONE',  ( 1.629816981350590055, -4.941769416738769571, 17.25000000000000000 ) ) ;
#11304=VECTOR ( 'NONE', #1360, 1000.000000000000000 ) ;
#11308=EDGE_LOOP ( 'NONE', ( #1549, #4089 ) ) ;
#11311=DIRECTION ( 'NONE',  ( -1.000000000000000000, 0.000000000000000000, 0.000000000000000000 ) ) ;
#11312=ORIENTED_EDGE ( 'NONE', *, *, #4407, .F. ) ;
#11313=CARTESIAN_POINT ( 'NONE',  ( -1.059188295049996231, -6.027090492554000534, 7.250000000000000000 ) ) ;
#11314=DIRECTION ( 'NONE',  ( 0.000000000000000000, 0.000000000000000000, 1.000000000000000000 ) ) ;
#11317=CARTESIAN_POINT ( 'NONE',  ( -35.05918829505000645, 27.97290950744599769, 7.250000000000000000 ) ) ;
#11318=EDGE_CURVE ( 'NONE', #10704, #4651, #5737, .T. ) ;
#11324=CARTESIAN_POINT ( 'NONE',  ( -14.81806704493275184, 30.13305483532533913, 55.03841218677168712 ) ) ;
#11328=ORIENTED_EDGE ( 'NONE', *, *, #2274, .T. ) ;
#11329=VECTOR ( 'NONE', #5820, 1000.000000000000000 ) ;
#11331=CYLINDRICAL_SURFACE ( 'NONE', #3379, 33.00000000000000000 ) ;
#11332=VERTEX_POINT ( 'NONE', #9207 ) ;
#11335=EDGE_CURVE ( 'NONE', #6329, #5535, #7504, .T. ) ;
#11336=CARTESIAN_POINT ( 'NONE',  ( -18.05918829504999934, 10.97290950744599947, 64.85000000000000853 ) ) ;
#11340=AXIS2_PLACEMENT_3D ( 'NONE', #11458, #9775, #9567 ) ;
#11344=EDGE_LOOP ( 'NONE', ( #8078, #2260, #12446, #1359 ) ) ;
#11345=ORIENTED_EDGE ( 'NONE', *, *, #1714, .F. ) ;
#11346=ORIENTED_EDGE ( 'NONE', *, *, #4794, .T. ) ;
#11347=AXIS2_PLACEMENT_3D ( 'NONE', #4005, #4210, #10490 ) ;
#11348=AXIS2_PLACEMENT_3D ( 'NONE', #9211, #609, #3074 ) ;
#11351=CIRCLE ( 'NONE', #7989, 4.750000000000000888 ) ;
#11355=DIRECTION ( 'NONE',  ( 0.000000000000000000, 0.000000000000000000, 1.000000000000000000 ) ) ;
#11357=CARTESIAN_POINT ( 'NONE',  ( -18.05918829504999934, 14.81548537210212046, 17.25000000000000000 ) ) ;
#11362=AXIS2_PLACEMENT_3D ( 'NONE', #11984, #1370, #8985 ) ;
#11363=CARTESIAN_POINT ( 'NONE',  ( -18.05918829504999934, 10.97290950744599947, 23.90000000000000213 ) ) ;
#11366=FACE_OUTER_BOUND ( 'NONE', #4849, .T. ) ;
#11367=CARTESIAN_POINT ( 'NONE',  ( -23.05918829504999934, 10.97290950744599947, 68.84999999999999432 ) ) ;
#11368=CARTESIAN_POINT ( 'NONE',  ( -23.33437236814141613, 12.98656286991741560, 68.21197126838345071 ) ) ;
#11371=CARTESIAN_POINT ( 'NONE',  ( -25.73489962141544751, -4.139534227248430120, 57.35000000000000142 ) ) ;
#11372=DIRECTION ( 'NONE',  ( 0.000000000000000000, 0.000000000000000000, -1.000000000000000000 ) ) ;
#11373=CIRCLE ( 'NONE', #8016, 15.45000000000000462 ) ;
#11374=CARTESIAN_POINT ( 'NONE',  ( -18.05918829504999934, 10.00028003023991907, 63.45000000000000284 ) ) ;
#11379=FACE_OUTER_BOUND ( 'NONE', #2616, .T. ) ;
#11380=VERTEX_POINT ( 'NONE', #11001 ) ;
#11381=CARTESIAN_POINT ( 'NONE',  ( -20.90380367978140796, 15.13103491944108470, 68.81278884182248134 ) ) ;
#11384=CARTESIAN_POINT ( 'NONE',  ( -18.05918829504999934, 19.07290950615085023, 63.35000000000700027 ) ) ;
#11385=DIRECTION ( 'NONE',  ( 0.000000000000000000, 0.000000000000000000, 1.000000000000000000 ) ) ;
#11387=CIRCLE ( 'NONE', #12282, 4.250000000000000000 ) ;
#11389=AXIS2_PLACEMENT_3D ( 'NONE', #1119, #10701, #6228 ) ;
#11391=ORIENTED_EDGE ( 'NONE', *, *, #9679, .F. ) ;
#11394=CARTESIAN_POINT ( 'NONE',  ( -14.49027952043798351, 30.08448262670741968, 55.77701067917464428 ) ) ;
#11396=ORIENTED_EDGE ( 'NONE', *, *, #8365, .F. ) ;
#11398=CIRCLE ( 'NONE', #11181, 2.700000000000001066 ) ;
#11400=FILL_AREA_STYLE ('',( #8177 ) ) ;
#11402=CARTESIAN_POINT ( 'NONE',  ( -18.05918829505000289, 3.354823934416959919, 61.65955166408550525 ) ) ;
#11405=FACE_OUTER_BOUND ( 'NONE', #7124, .T. ) ;
#11406=CARTESIAN_POINT ( 'NONE',  ( -23.49332020752115113, 0.2738342970428629952, 61.85000000000000142 ) ) ;
#11408=CARTESIAN_POINT ( 'NONE',  ( -18.05918829504999934, 10.97290950744599947, 57.35000000000000142 ) ) ;
#11409=CARTESIAN_POINT ( 'NONE',  ( -19.55892036123722022, 27.90662746311071629, 57.54959831248249458 ) ) ;
#11410=CARTESIAN_POINT ( 'NONE',  ( -11.30918829504999934, 10.97290950744599947, 63.35000000000000142 ) ) ;
#11413=ORIENTED_EDGE ( 'NONE', *, *, #1714, .T. ) ;
#11415=EDGE_CURVE ( 'NONE', #3674, #5251, #5522, .T. ) ;
#11416=ORIENTED_EDGE ( 'NONE', *, *, #8796, .T. ) ;
#11418=ORIENTED_EDGE ( 'NONE', *, *, #5686, .T. ) ;
#11421=CARTESIAN_POINT ( 'NONE',  ( -20.28447066877352611, 30.25344248482696585, 60.89002542176228872 ) ) ;
#11422=AXIS2_PLACEMENT_3D ( 'NONE', #10057, #1386, #7722 ) ;
#11423=CARTESIAN_POINT ( 'NONE',  ( -18.05918829504999934, 10.97290950744599947, 68.84999999999999432 ) ) ;
#11424=DIRECTION ( 'NONE',  ( 0.000000000000000000, 1.000000000000000000, 2.202823461557851130E-15 ) ) ;
#11426=LINE ( 'NONE', #10249, #11825 ) ;
#11427=ADVANCED_FACE ( 'NONE', ( #2492 ), #1199, .T. ) ;
#11428=AXIS2_PLACEMENT_3D ( 'NONE', #11501, #5006, #7164 ) ;
#11429=LINE ( 'NONE', #13583, #6377 ) ;
#11431=EDGE_LOOP ( 'NONE', ( #13198, #2333, #11121, #10943 ) ) ;
#11432=DIRECTION ( 'NONE',  ( -1.000000000000000000, 1.799713116287177675E-15, 0.000000000000000000 ) ) ;
#11433=DIRECTION ( 'NONE',  ( -2.267612386897784912E-16, 1.000000000000000000, 0.000000000000000000 ) ) ;
#11434=EDGE_CURVE ( 'NONE', #2075, #7909, #4498, .T. ) ;
#11436=CARTESIAN_POINT ( 'NONE',  ( -23.64255140084592099, 12.71465888092544638, 68.00600096910662273 ) ) ;
#11437=CARTESIAN_POINT ( 'NONE',  ( -21.69796668809184936, 15.09714177616359798, 30.59999999999999787 ) ) ;
#11439=LINE ( 'NONE', #1879, #7361 ) ;
#11440=AXIS2_PLACEMENT_3D ( 'NONE', #6320, #4302, #6162 ) ;
#11441=CARTESIAN_POINT ( 'NONE',  ( -34.72201093190195564, 10.97290950744599947, 5.250000000000000000 ) ) ;
#11442=FACE_BOUND ( 'NONE', #5694, .T. ) ;
#11443=ORIENTED_EDGE ( 'NONE', *, *, #12847, .F. ) ;
#11446=VERTEX_POINT ( 'NONE', #6647 ) ;
#11448=CARTESIAN_POINT ( 'NONE',  ( -18.05918829504999934, 10.97290950744599947, 6.250000000000000000 ) ) ;
#11449=VERTEX_POINT ( 'NONE', #7759 ) ;
#11450=EDGE_LOOP ( 'NONE', ( #5263, #12365, #5144, #11749, #216, #6831, #5855, #3945, #2783, #10430, #12995, #6844, #2623, #7626 ) ) ;
#11452=EDGE_CURVE ( 'NONE', #918, #13546, #9593, .T. ) ;
#11453=CARTESIAN_POINT ( 'NONE',  ( -25.73489962141550080, -4.139534227248430120, 60.85000000000000142 ) ) ;
#11454=DIRECTION ( 'NONE',  ( 0.000000000000000000, 0.000000000000000000, -1.000000000000000000 ) ) ;
#11456=VERTEX_POINT ( 'NONE', #148 ) ;
#11457=CARTESIAN_POINT ( 'NONE',  ( -1.859188294733151059, 19.07290950803865215, 63.35000000001166143 ) ) ;
#11458=CARTESIAN_POINT ( 'NONE',  ( -1.059188295049996231, -6.027090492554000534, 68.85549045786049760 ) ) ;
#11460=CIRCLE ( 'NONE', #9007, 16.50000000000000000 ) ;
#11462=CARTESIAN_POINT ( 'NONE',  ( -15.59946857746960447, 30.22967062530674909, 60.68251737619485198 ) ) ;
#11463=ORIENTED_EDGE ( 'NONE', *, *, #7012, .F. ) ;
#11464=CARTESIAN_POINT ( 'NONE',  ( -18.05918829504999934, 10.97290950744599947, 64.85000000000000853 ) ) ;
#11466=DIRECTION ( 'NONE',  ( -1.000000000000000000, 0.000000000000000000, 0.000000000000000000 ) ) ;
#11469=CARTESIAN_POINT ( 'NONE',  ( -35.05918829505000645, 27.97290950744599769, 7.250000000000000000 ) ) ;
#11470=FACE_BOUND ( 'NONE', #7717, .T. ) ;
#11471=LINE ( 'NONE', #8184, #2491 ) ;
#11473=ORIENTED_EDGE ( 'NONE', *, *, #2498, .T. ) ;
#11475=EDGE_CURVE ( 'NONE', #4563, #3000, #6446, .T. ) ;
#11476=CARTESIAN_POINT ( 'NONE',  ( -5.789834139046009298, 27.54455229823479812, 64.85000000000000853 ) ) ;
#11478=EDGE_LOOP ( 'NONE', ( #5868, #2022, #11061, #9299 ) ) ;
#11479=VERTEX_POINT ( 'NONE', #6517 ) ;
#11482=CARTESIAN_POINT ( 'NONE',  ( -20.15923745082466567, 30.26546654931225788, 60.99209064090569399 ) ) ;
#11484=LINE ( 'NONE', #10437, #10881 ) ;
#11486=EDGE_CURVE ( 'NONE', #2900, #5058, #4883, .T. ) ;
#11487=AXIS2_PLACEMENT_3D ( 'NONE', #10633, #144, #1056 ) ;
#11488=CYLINDRICAL_SURFACE ( 'NONE', #8930, 24.92993838181874722 ) ;
#11493=EDGE_LOOP ( 'NONE', ( #13720, #3346 ) ) ;
#11496=CARTESIAN_POINT ( 'NONE',  ( -7.241070169793063727, -7.867426463707971607, 83.57661607529820458 ) ) ;
#11497=ORIENTED_EDGE ( 'NONE', *, *, #3497, .F. ) ;
#11498=DIRECTION ( 'NONE',  ( 0.000000000000000000, 0.000000000000000000, 1.000000000000000000 ) ) ;
#11499=DIRECTION ( 'NONE',  ( 1.000000000000000000, 0.000000000000000000, 0.000000000000000000 ) ) ;
#11501=CARTESIAN_POINT ( 'NONE',  ( -18.05918829504999934, 10.97290950744599947, 27.09999999999999787 ) ) ;
#11504=DIRECTION ( 'NONE',  ( 0.000000000000000000, 0.000000000000000000, -1.000000000000000000 ) ) ;
#11505=ADVANCED_FACE ( 'NONE', ( #13223 ), #6788, .T. ) ;
#11506=PLANE ( 'NONE',  #13682 ) ;
#11509=CIRCLE ( 'NONE', #8826, 6.849999999999999645 ) ;
#11511=ADVANCED_FACE ( 'NONE', ( #7056 ), #13284, .F. ) ;
#11512=ORIENTED_EDGE ( 'NONE', *, *, #1244, .T. ) ;
#11513=CARTESIAN_POINT ( 'NONE',  ( 3.690811704950004657, -6.027090492554000534, 7.250000000000000000 ) ) ;
#11514=VERTEX_POINT ( 'NONE', #4711 ) ;
#11516=CARTESIAN_POINT ( 'NONE',  ( -20.60782847033100040, 15.39217156908933859, 68.75034594041223102 ) ) ;
#11519=DIRECTION ( 'NONE',  ( 0.000000000000000000, 1.000000000000000000, 0.000000000000000000 ) ) ;
#11520=EDGE_CURVE ( 'NONE', #9971, #1130, #13780, .T. ) ;
#11524=EDGE_LOOP ( 'NONE', ( #2130, #7159 ) ) ;
#11525=CARTESIAN_POINT ( 'NONE',  ( -14.34316551184594424, 30.06124217888930872, 56.29137106245990196 ) ) ;
#11530=CARTESIAN_POINT ( 'NONE',  ( -23.42001676333060090, -4.028726038184999858, 63.45000000000000284 ) ) ;
#11536=AXIS2_PLACEMENT_3D ( 'NONE', #11999, #11031, #4741 ) ;
#11537=FACE_OUTER_BOUND ( 'NONE', #23, .T. ) ;
#11538=DIRECTION ( 'NONE',  ( 0.4528443260392608916, 0.8915896008669279560, 0.000000000000000000 ) ) ;
#11539=CARTESIAN_POINT ( 'NONE',  ( -17.66997072932066359, 27.96944788186879194, 58.81217888752696155 ) ) ;
#11540=PLANE ( 'NONE',  #12507 ) ;
#11542=ORIENTED_EDGE ( 'NONE', *, *, #3991, .F. ) ;
#11543=AXIS2_PLACEMENT_3D ( 'NONE', #590, #10365, #4922 ) ;
#11545=ADVANCED_FACE ( 'NONE', ( #3722 ), #13269, .F. ) ;
#11546=ORIENTED_EDGE ( 'NONE', *, *, #3572, .T. ) ;
#11548=CARTESIAN_POINT ( 'NONE',  ( -18.05918829504999934, 10.97290950744599947, 61.86500000000000199 ) ) ;
#11549=ORIENTED_EDGE ( 'NONE', *, *, #10067, .F. ) ;
#11550=CARTESIAN_POINT ( 'NONE',  ( -18.96245718805280944, 30.34273348207711507, 61.58489515985737484 ) ) ;
#11551=VECTOR ( 'NONE', #7660, 1000.000000000000000 ) ;
#11552=CARTESIAN_POINT ( 'NONE',  ( -18.93945023811382455, 26.94867995574305297, 56.13543987128847590 ) ) ;
#11554=CARTESIAN_POINT ( 'NONE',  ( -25.33503448090910126, 29.19143287883919768, 64.85000000000000853 ) ) ;
#11556=AXIS2_PLACEMENT_3D ( 'NONE', #1134, #2282, #6519 ) ;
#11557=PLANE ( 'NONE',  #10941 ) ;
#11559=ORIENTED_EDGE ( 'NONE', *, *, #10936, .F. ) ;
#11561=AXIS2_PLACEMENT_3D ( 'NONE', #3432, #7770, #10895 ) ;
#11565=ORIENTED_EDGE ( 'NONE', *, *, #828, .T. ) ;
#11567=VECTOR ( 'NONE', #8086, 1000.000000000000114 ) ;
#11570=EDGE_CURVE ( 'NONE', #1264, #13079, #5090, .T. ) ;
#11573=DIRECTION ( 'NONE',  ( -1.000000000000000000, 0.000000000000000000, 0.000000000000000000 ) ) ;
#11574=DIRECTION ( 'NONE',  ( 0.000000000000000000, 0.000000000000000000, 1.000000000000000000 ) ) ;
#11580=AXIS2_PLACEMENT_3D ( 'NONE', #11374, #5076, #2947 ) ;
#11583=CONICAL_SURFACE ( 'NONE', #12029, 4.250000000000000000, 0.7853981633974518317 ) ;
#11584=ORIENTED_EDGE ( 'NONE', *, *, #13603, .T. ) ;
#11587=EDGE_CURVE ( 'NONE', #2353, #9556, #5528, .T. ) ;
#11589=DIRECTION ( 'NONE',  ( -1.000000000000000000, 0.000000000000000000, 0.000000000000000000 ) ) ;
#11593=LINE ( 'NONE', #9227, #9784 ) ;
#11594=EDGE_CURVE ( 'NONE', #1667, #803, #7125, .T. ) ;
#11596=AXIS2_PLACEMENT_3D ( 'NONE', #2612, #10143, #10081 ) ;
#11597=CIRCLE ( 'NONE', #6016, 34.69999999999999574 ) ;
#11600=CARTESIAN_POINT ( 'NONE',  ( -14.49575039789787390, 30.08533272846046813, 58.93884046276453148 ) ) ;
#11601=EDGE_LOOP ( 'NONE', ( #13470, #11797, #10869, #13708 ) ) ;
#11602=PLANE ( 'NONE',  #6151 ) ;
#11603=ADVANCED_FACE ( 'NONE', ( #6303 ), #7253, .T. ) ;
#11604=DIRECTION ( 'NONE',  ( 0.000000000000000000, -1.000000000000000000, 0.000000000000000000 ) ) ;
#11605=EDGE_LOOP ( 'NONE', ( #9636, #10304, #65, #909 ) ) ;
#11607=CYLINDRICAL_SURFACE ( 'NONE', #10242, 34.69999999999999574 ) ;
#11610=CONICAL_SURFACE ( 'NONE', #6913, 6.850000000000002309, 0.7853981633974433940 ) ;
#11613=CIRCLE ( 'NONE', #466, 7.618085573000000110 ) ;
#11615=DIRECTION ( 'NONE',  ( 0.000000000000000000, 0.000000000000000000, -1.000000000000000000 ) ) ;
#11616=ORIENTED_EDGE ( 'NONE', *, *, #7980, .T. ) ;
#11617=ORIENTED_EDGE ( 'NONE', *, *, #12028, .F. ) ;
#11619=AXIS2_PLACEMENT_3D ( 'NONE', #4267, #11871, #7583 ) ;
#11620=AXIS2_PLACEMENT_3D ( 'NONE', #12964, #2232, #2376 ) ;
#11621=VERTEX_POINT ( 'NONE', #9377 ) ;
#11623=ORIENTED_EDGE ( 'NONE', *, *, #10775, .T. ) ;
#11624=DIRECTION ( 'NONE',  ( 0.000000000000000000, 0.000000000000000000, -1.000000000000000000 ) ) ;
#11625=CARTESIAN_POINT ( 'NONE',  ( -35.05918829505000645, -6.027090492554000534, 5.250000000000000000 ) ) ;
#11626=ORIENTED_EDGE ( 'NONE', *, *, #7645, .F. ) ;
#11628=LINE ( 'NONE', #8608, #13412 ) ;
#11629=CARTESIAN_POINT ( 'NONE',  ( -17.92868857854553610, 26.97291705118750116, 55.84994910580621763 ) ) ;
#11632=FACE_OUTER_BOUND ( 'NONE', #7235, .T. ) ;
#11633=CIRCLE ( 'NONE', #12749, 6.450000000000001066 ) ;
#11637=B_SPLINE_CURVE_WITH_KNOTS ( 'NONE', 3,
 ( #7767, #13290, #7838, #10935 ),
 .UNSPECIFIED., .F., .F.,
 ( 4, 4 ),
 ( 0.000000000000000000, 1.000000000000000000 ),
 .UNSPECIFIED. ) ;
#11638=VERTEX_POINT ( 'NONE', #8326 ) ;
#11640=CONICAL_SURFACE ( 'NONE', #12755, 2.800000000000000266, 0.7853981633974419507 ) ;
#11645=VERTEX_POINT ( 'NONE', #5035 ) ;
#11654=CARTESIAN_POINT ( 'NONE',  ( 0.000000000000000000, 0.000000000000000000, 0.000000000000000000 ) ) ;
#11660=CARTESIAN_POINT ( 'NONE',  ( -10.25088531517542023, -8.860076549334110041, 17.25000000000000000 ) ) ;
#11663=EDGE_LOOP ( 'NONE', ( #1623, #8006, #11549, #2118, #6020 ) ) ;
#11664=CARTESIAN_POINT ( 'NONE',  ( -13.12714905285830547, 8.656502101311028596, 68.40310675162322696 ) ) ;
#11667=DIRECTION ( 'NONE',  ( 0.000000000000000000, -1.000000000000000000, 0.000000000000000000 ) ) ;
#11668=ORIENTED_EDGE ( 'NONE', *, *, #5532, .T. ) ;
#11669=CARTESIAN_POINT ( 'NONE',  ( -15.99409762314761885, 6.127015440082126396, 68.58244592664642880 ) ) ;
#11670=DIRECTION ( 'NONE',  ( 0.000000000000000000, 0.000000000000000000, 1.000000000000000000 ) ) ;
#11672=CIRCLE ( 'NONE', #5202, 1.725000000000000755 ) ;
#11673=CARTESIAN_POINT ( 'NONE',  ( -15.27301918356318033, 30.19258199384825403, 54.36937504594504134 ) ) ;
#11675=VERTEX_POINT ( 'NONE', #9509 ) ;
#11679=CARTESIAN_POINT ( 'NONE',  ( -1.059188295049996231, -6.027090492554000534, 17.25000000000000000 ) ) ;
#11683=DIRECTION ( 'NONE',  ( 0.000000000000000000, 0.000000000000000000, 1.000000000000000000 ) ) ;
#11684=ADVANCED_FACE ( 'NONE', ( #11405 ), #12233, .T. ) ;
#11685=DIRECTION ( 'NONE',  ( 0.000000000000000000, 0.000000000000000000, -1.000000000000000000 ) ) ;
#11686=ORIENTED_EDGE ( 'NONE', *, *, #13401, .F. ) ;
#11687=EDGE_LOOP ( 'NONE', ( #8799, #5282, #760, #2070 ) ) ;
#11688=ADVANCED_FACE ( 'NONE', ( #10353 ), #6200, .F. ) ;
#11693=CARTESIAN_POINT ( 'NONE',  ( -8.930582367738718830, 12.35910059330153921, 64.85000000000000853 ) ) ;
#11694=DIRECTION ( 'NONE',  ( 0.000000000000000000, 0.000000000000000000, -1.000000000000000000 ) ) ;
#11695=ORIENTED_EDGE ( 'NONE', *, *, #5785, .F. ) ;
#11696=DIRECTION ( 'NONE',  ( -0.2878798879079283446, 0.9576665234506834823, 0.000000000000000000 ) ) ;
#11700=EDGE_CURVE ( 'NONE', #11290, #4952, #5311, .T. ) ;
#11701=CARTESIAN_POINT ( 'NONE',  ( -1.059188295049996231, -6.027090492554000534, 64.85000000000000853 ) ) ;
#11703=ORIENTED_EDGE ( 'NONE', *, *, #12185, .F. ) ;
#11704=EDGE_CURVE ( 'NONE', #13581, #5483, #2211, .T. ) ;
#11706=CARTESIAN_POINT ( 'NONE',  ( -25.32001676333059947, -4.028726038184999858, 62.14999999999999858 ) ) ;
#11710=CIRCLE ( 'NONE', #7015, 3.000000000000001332 ) ;
#11711=CARTESIAN_POINT ( 'NONE',  ( -20.64360816717656988, 30.21612105584335595, 54.14118912831367680 ) ) ;
#11713=LINE ( 'NONE', #2158, #4197 ) ;
#11715=CARTESIAN_POINT ( 'NONE',  ( -30.80918829504999934, 27.97290950744599769, 64.35000000000000853 ) ) ;
#11717=( NAMED_UNIT ( * ) PLANE_ANGLE_UNIT ( ) SI_UNIT ( $, .RADIAN. ) );
#11718=VECTOR ( 'NONE', #7573, 1000.000000000000227 ) ;
#11720=DIRECTION ( 'NONE',  ( 0.000000000000000000, 0.000000000000000000, -1.000000000000000000 ) ) ;
#11721=EDGE_CURVE ( 'NONE', #9242, #6126, #7987, .T. ) ;
#11722=VERTEX_POINT ( 'NONE', #5438 ) ;
#11723=ORIENTED_EDGE ( 'NONE', *, *, #9793, .T. ) ;
#11727=CARTESIAN_POINT ( 'NONE',  ( -35.05918829505000645, -6.027090492554000534, 64.85000000000000853 ) ) ;
#11730=CARTESIAN_POINT ( 'NONE',  ( -18.05918829504999934, 10.97290950744599947, 57.35000000000000142 ) ) ;
#11731=ORIENTED_EDGE ( 'NONE', *, *, #1546, .F. ) ;
#11733=ORIENTED_EDGE ( 'NONE', *, *, #221, .T. ) ;
#11734=CARTESIAN_POINT ( 'NONE',  ( -18.05918829504999934, 10.97290950744599947, 62.14999999999999858 ) ) ;
#11736=DIRECTION ( 'NONE',  ( -1.000000000000000000, 0.000000000000000000, 0.000000000000000000 ) ) ;
#11739=CARTESIAN_POINT ( 'NONE',  ( -12.87735031270726083, -6.265087914666309210, 63.45000000000000284 ) ) ;
#11740=CARTESIAN_POINT ( 'NONE',  ( -1.899121662050003101, 2.892876190445991202, 63.34900083300006202 ) ) ;
#11742=FACE_BOUND ( 'NONE', #9682, .T. ) ;
#11743=ORIENTED_EDGE ( 'NONE', *, *, #2226, .F. ) ;
#11745=DIRECTION ( 'NONE',  ( 1.000000000000000000, 0.000000000000000000, 0.000000000000000000 ) ) ;
#11747=EDGE_CURVE ( 'NONE', #7555, #2082, #2408, .T. ) ;
#11748=ORIENTED_EDGE ( 'NONE', *, *, #10568, .T. ) ;
#11749=ORIENTED_EDGE ( 'NONE', *, *, #1282, .F. ) ;
#11750=AXIS2_PLACEMENT_3D ( 'NONE', #13607, #10275, #900 ) ;
#11753=DIRECTION ( 'NONE',  ( 0.000000000000000000, 0.000000000000000000, -1.000000000000000000 ) ) ;
#11754=ORIENTED_EDGE ( 'NONE', *, *, #13648, .T. ) ;
#11755=DIRECTION ( 'NONE',  ( -0.9576665234506835933, -0.2878798879079284001, 0.000000000000000000 ) ) ;
#11760=CARTESIAN_POINT ( 'NONE',  ( -35.72201093190194854, 10.97290950744599947, 5.250000000000000000 ) ) ;
#11763=EDGE_CURVE ( 'NONE', #5219, #10722, #13340, .T. ) ;
#11764=DIRECTION ( 'NONE',  ( 0.000000000000000000, 0.000000000000000000, 1.000000000000000000 ) ) ;
#11767=VECTOR ( 'NONE', #6687, 1000.000000000000000 ) ;
#11771=CARTESIAN_POINT ( 'NONE',  ( -20.82467356178127105, 30.19507513500936824, 54.34448619228547983 ) ) ;
#11772=CARTESIAN_POINT ( 'NONE',  ( -7.241070169793059286, 29.81324547859994922, 17.25000000000000000 ) ) ;
#11773=CARTESIAN_POINT ( 'NONE',  ( -2.819094421049990640, 3.352862570445993562, 61.63595870799996845 ) ) ;
#11775=DIRECTION ( 'NONE',  ( 0.000000000000000000, 0.000000000000000000, 1.000000000000000000 ) ) ;
#11777=FACE_OUTER_BOUND ( 'NONE', #7895, .T. ) ;
#11781=ORIENTED_EDGE ( 'NONE', *, *, #688, .F. ) ;
#11782=EDGE_LOOP ( 'NONE', ( #1995, #3156 ) ) ;
#11785=CARTESIAN_POINT ( 'NONE',  ( -1.059188295049996231, -6.027090492554000534, 7.250000000000000000 ) ) ;
#11786=FACE_OUTER_BOUND ( 'NONE', #983, .T. ) ;
#11787=( NAMED_UNIT ( * ) SI_UNIT ( $, .STERADIAN. ) SOLID_ANGLE_UNIT ( ) );
#11789=AXIS2_PLACEMENT_3D ( 'NONE', #1610, #2682, #6839 ) ;
#11790=AXIS2_PLACEMENT_3D ( 'NONE', #13030, #529, #6599 ) ;
#11791=CARTESIAN_POINT ( 'NONE',  ( -35.05918829505000645, 27.97290950744599769, 58.85000000000000142 ) ) ;
#11794=CARTESIAN_POINT ( 'NONE',  ( -10.78334210919089919, 29.19143287883919768, 64.85000000000000853 ) ) ;
#11797=ORIENTED_EDGE ( 'NONE', *, *, #221, .F. ) ;
#11801=ORIENTED_EDGE ( 'NONE', *, *, #523, .T. ) ;
#11802=VERTEX_POINT ( 'NONE', #5376 ) ;
#11803=CARTESIAN_POINT ( 'NONE',  ( -11.70083760351054103, 35.47811937223634970, 17.25000000000000000 ) ) ;
#11811=CARTESIAN_POINT ( 'NONE',  ( -34.78181777225609750, 10.00028003023991907, 63.45000000000000284 ) ) ;
#11812=AXIS2_PLACEMENT_3D ( 'NONE', #7905, #581, #6858 ) ;
#11814=ADVANCED_FACE ( 'NONE', ( #8740 ), #136, .T. ) ;
#11825=VECTOR ( 'NONE', #659, 1000.000000000000000 ) ;
#11827=CARTESIAN_POINT ( 'NONE',  ( 0.09777679598750591006, 23.36596564213564875, 7.250000000000000000 ) ) ;
#11828=ORIENTED_EDGE ( 'NONE', *, *, #4395, .F. ) ;
#11832=CYLINDRICAL_SURFACE ( 'NONE', #6723, 4.000000000000000888 ) ;
#11833=CARTESIAN_POINT ( 'NONE',  ( 1.097360187335109982, -3.327306731351814761, 68.85549045786049760 ) ) ;
#11836=VECTOR ( 'NONE', #1871, 1000.000000000000227 ) ;
#11838=VECTOR ( 'NONE', #8187, 1000.000000000000114 ) ;
#11839=VECTOR ( 'NONE', #1661, 1000.000000000000114 ) ;
#11841=EDGE_LOOP ( 'NONE', ( #9664, #1740, #1477, #1434, #185, #3946 ) ) ;
#11845=DIRECTION ( 'NONE',  ( -0.6615960714621568206, 0.7498604124941127269, 0.000000000000000000 ) ) ;
#11846=CARTESIAN_POINT ( 'NONE',  ( -20.35918349919666781, 30.24616810948638701, 53.87192440031903118 ) ) ;
#11849=CIRCLE ( 'NONE', #11619, 6.450000000000019718 ) ;
#11850=CARTESIAN_POINT ( 'NONE',  ( -18.05918829504999934, 10.97290950744599947, 62.85000000000000142 ) ) ;
#11852=CIRCLE ( 'NONE', #6275, 16.72262947720610171 ) ;
#11854=FACE_OUTER_BOUND ( 'NONE', #5725, .T. ) ;
#11855=CARTESIAN_POINT ( 'NONE',  ( -1.059188295049996231, 10.97290950744599947, 64.35000000000000853 ) ) ;
#11856=DIRECTION ( 'NONE',  ( 1.000000000000000000, 0.000000000000000000, 0.000000000000000000 ) ) ;
#11858=EDGE_CURVE ( 'NONE', #12302, #5782, #8527, .T. ) ;
#11860=CIRCLE ( 'NONE', #8960, 8.250000000000001776 ) ;
#11865=DIRECTION ( 'NONE',  ( 0.9496839325805416232, 0.3132098788326400096, 0.000000000000000000 ) ) ;
#11866=EDGE_LOOP ( 'NONE', ( #6005, #13558, #3549, #7456, #10522, #6102 ) ) ;
#11867=EDGE_LOOP ( 'NONE', ( #11293, #12378, #7160, #12592 ) ) ;
#11868=VERTEX_POINT ( 'NONE', #9654 ) ;
#11869=ORIENTED_EDGE ( 'NONE', *, *, #1488, .F. ) ;
#11870=CARTESIAN_POINT ( 'NONE',  ( -10.44110272205000101, 10.97290950744599947, 61.65955166399999854 ) ) ;
#11871=DIRECTION ( 'NONE',  ( -0.000000000000000000, -0.000000000000000000, 1.000000000000000000 ) ) ;
#11872=DIRECTION ( 'NONE',  ( 0.000000000000000000, 0.000000000000000000, -1.000000000000000000 ) ) ;
#11873=DIRECTION ( 'NONE',  ( 0.000000000000000000, 0.000000000000000000, -1.000000000000000000 ) ) ;
#11874=PLANE ( 'NONE',  #3598 ) ;
#11875=AXIS2_PLACEMENT_3D ( 'NONE', #7584, #11872, #9768 ) ;
#11876=FACE_OUTER_BOUND ( 'NONE', #4558, .T. ) ;
#11877=LINE ( 'NONE', #6620, #3983 ) ;
#11881=CARTESIAN_POINT ( 'NONE',  ( -15.78544589689968802, 30.24873049213536191, 53.85022182113912947 ) ) ;
#11884=ORIENTED_EDGE ( 'NONE', *, *, #11335, .F. ) ;
#11886=CARTESIAN_POINT ( 'NONE',  ( 8.157609394192110841, 24.73469418910620021, 17.25000000000000000 ) ) ;
#11889=STYLED_ITEM ( 'NONE', ( #4728 ), #5212 ) ;
#11890=ORIENTED_EDGE ( 'NONE', *, *, #8319, .T. ) ;
#11891=VERTEX_POINT ( 'NONE', #5790 ) ;
#11892=ORIENTED_EDGE ( 'NONE', *, *, #4950, .F. ) ;
#11894=ORIENTED_EDGE ( 'NONE', *, *, #350, .T. ) ;
#11897=AXIS2_PLACEMENT_3D ( 'NONE', #9814, #2355, #236 ) ;
#11900=EDGE_CURVE ( 'NONE', #8158, #7243, #12091, .T. ) ;
#11901=CARTESIAN_POINT ( 'NONE',  ( -18.05918829504999934, 10.97290950744599947, 57.35000000000000142 ) ) ;
#11902=VERTEX_POINT ( 'NONE', #11113 ) ;
#11904=DIRECTION ( 'NONE',  ( 1.000000000000000000, 0.000000000000000000, 0.000000000000000000 ) ) ;
#11906=DIRECTION ( 'NONE',  ( -1.000000000000000000, 0.000000000000000000, 0.000000000000000000 ) ) ;
#11909=CIRCLE ( 'NONE', #11024, 2.800000000000000266 ) ;
#11912=ORIENTED_EDGE ( 'NONE', *, *, #7920, .F. ) ;
#11916=FACE_OUTER_BOUND ( 'NONE', #1941, .T. ) ;
#11917=ADVANCED_FACE ( 'NONE', ( #11180 ), #5098, .F. ) ;
#11919=CARTESIAN_POINT ( 'NONE',  ( -18.82359282014710544, 30.34769730472570970, 53.07963013742637060 ) ) ;
#11920=CARTESIAN_POINT ( 'NONE',  ( -17.23821357112329977, 5.029341513162310484, 68.84999999999999432 ) ) ;
#11921=CARTESIAN_POINT ( 'NONE',  ( -15.41280400920135030, 7.973467857469549891, 30.59999999999999787 ) ) ;
#11924=ADVANCED_FACE ( 'NONE', ( #8029 ), #2549, .T. ) ;
#11930=VERTEX_POINT ( 'NONE', #6908 ) ;
#11933=EDGE_CURVE ( 'NONE', #9462, #5579, #500, .T. ) ;
#11934=DIRECTION ( 'NONE',  ( 1.000000000000000000, 0.000000000000000000, -0.000000000000000000 ) ) ;
#11943=EDGE_CURVE ( 'NONE', #10781, #12773, #1402, .T. ) ;
#11945=ORIENTED_EDGE ( 'NONE', *, *, #2330, .F. ) ;
#11946=CARTESIAN_POINT ( 'NONE',  ( -17.10968755856460177, 30.34086823225404217, 53.12849656952644750 ) ) ;
#11948=ORIENTED_EDGE ( 'NONE', *, *, #12459, .F. ) ;
#11950=FILL_AREA_STYLE ('',( #4404 ) ) ;
#11952=DIRECTION ( 'NONE',  ( 1.000000000000000000, 0.000000000000000000, 0.000000000000000000 ) ) ;
#11953=CARTESIAN_POINT ( 'NONE',  ( -18.05918829504999934, 10.97290950744599947, 57.35000000000000142 ) ) ;
#11954=EDGE_CURVE ( 'NONE', #13684, #5561, #9156, .T. ) ;
#11957=ORIENTED_EDGE ( 'NONE', *, *, #1865, .T. ) ;
#11960=DIRECTION ( 'NONE',  ( 1.000000000000000000, 0.000000000000000000, 0.000000000000000000 ) ) ;
#11961=ORIENTED_EDGE ( 'NONE', *, *, #6171, .F. ) ;
#11962=ORIENTED_EDGE ( 'NONE', *, *, #3076, .T. ) ;
#11965=CARTESIAN_POINT ( 'NONE',  ( -18.05918829504999934, 10.97290950744599947, 62.14999999999999858 ) ) ;
#11967=VECTOR ( 'NONE', #11015, 1000.000000000000000 ) ;
#11969=CARTESIAN_POINT ( 'NONE',  ( -16.65773704950522927, 26.91141943044650375, 56.81390271690813876 ) ) ;
#11971=DIRECTION ( 'NONE',  ( 0.000000000000000000, 0.000000000000000000, -1.000000000000000000 ) ) ;
#11977=DIRECTION ( 'NONE',  ( -1.000000000000000000, 0.000000000000000000, 0.000000000000000000 ) ) ;
#11978=DIRECTION ( 'NONE',  ( 0.000000000000000000, 0.000000000000000000, -1.000000000000000000 ) ) ;
#11980=CARTESIAN_POINT ( 'NONE',  ( -19.10270367411500203, 30.33713881009503410, 53.15513206184487416 ) ) ;
#11982=ORIENTED_EDGE ( 'NONE', *, *, #7081, .T. ) ;
#11984=CARTESIAN_POINT ( 'NONE',  ( -18.05918829504999934, 10.97290950744599947, 67.84999999999999432 ) ) ;
#11985=ADVANCED_FACE ( 'NONE', ( #6777 ), #12026, .T. ) ;
#11987=CARTESIAN_POINT ( 'NONE',  ( -35.05918829505000645, 27.97290950744599769, 5.250000000000000000 ) ) ;
#11988=CIRCLE ( 'NONE', #4408, 4.750000000000000888 ) ;
#11989=CARTESIAN_POINT ( 'NONE',  ( -35.05918829505000645, -6.027090492554000534, 64.85000000000000853 ) ) ;
#11996=DIRECTION ( 'NONE',  ( 1.000000000000000000, 0.000000000000000000, 0.000000000000000000 ) ) ;
#11997=ORIENTED_EDGE ( 'NONE', *, *, #4399, .T. ) ;
#11999=CARTESIAN_POINT ( 'NONE',  ( -11.74835982676941981, -4.028726038184999858, 62.14999999999999858 ) ) ;
#12000=DIRECTION ( 'NONE',  ( 0.000000000000000000, 1.000000000000000000, 0.000000000000000000 ) ) ;
#12002=EDGE_CURVE ( 'NONE', #10219, #5663, #5759, .T. ) ;
#12007=CIRCLE ( 'NONE', #9552, 6.419999999999999929 ) ;
#12011=ADVANCED_FACE ( 'NONE', ( #1468, #5717 ), #4695, .F. ) ;
#12013=DIRECTION ( 'NONE',  ( -1.000000000000000000, 0.000000000000000000, 0.000000000000000000 ) ) ;
#12015=VECTOR ( 'NONE', #12371, 1000.000000000000114 ) ;
#12016=ORIENTED_EDGE ( 'NONE', *, *, #3243, .T. ) ;
#12017=CARTESIAN_POINT ( 'NONE',  ( -18.05918829504999934, 10.97290950744599947, 63.14999999999999858 ) ) ;
#12018=AXIS2_PLACEMENT_3D ( 'NONE', #9057, #7024, #6961 ) ;
#12019=PLANE ( 'NONE',  #12283 ) ;
#12021=EDGE_LOOP ( 'NONE', ( #5915, #2524, #12954, #9429 ) ) ;
#12022=CARTESIAN_POINT ( 'NONE',  ( -16.40519811639460102, 9.098258476210720147, 67.84999999999999432 ) ) ;
#12026=CONICAL_SURFACE ( 'NONE', #9348, 16.75000000000000355, 0.7853981633974447263 ) ;
#12028=EDGE_CURVE ( 'NONE', #5017, #9550, #8000, .T. ) ;
#12029=AXIS2_PLACEMENT_3D ( 'NONE', #6540, #8699, #1156 ) ;
#12032=EDGE_LOOP ( 'NONE', ( #8981, #11869, #1982, #218 ) ) ;
#12033=VERTEX_POINT ( 'NONE', #10403 ) ;
#12034=EDGE_CURVE ( 'NONE', #10707, #10997, #9901, .T. ) ;
#12037=CARTESIAN_POINT ( 'NONE',  ( -41.50918829505000218, -6.027090492554000534, 17.25000000000000000 ) ) ;
#12040=VECTOR ( 'NONE', #11207, 1000.000000000000000 ) ;
#12041=LINE ( 'NONE', #5733, #7183 ) ;
#12046=CIRCLE ( 'NONE', #6473, 16.95000000000000284 ) ;
#12047=ORIENTED_EDGE ( 'NONE', *, *, #5244, .T. ) ;
#12049=CARTESIAN_POINT ( 'NONE',  ( -18.05918829504999934, 10.97290950744599947, 62.14999999999999858 ) ) ;
#12051=CARTESIAN_POINT ( 'NONE',  ( -24.20502162805000168, 10.97290950744599947, 60.60999999999999943 ) ) ;
#12052=CARTESIAN_POINT ( 'NONE',  ( -20.82417809436781297, 30.19514031291545919, 60.35623975441919242 ) ) ;
#12054=FACE_OUTER_BOUND ( 'NONE', #11601, .T. ) ;
#12057=CARTESIAN_POINT ( 'NONE',  ( -5.631644894983189431, 10.97290950744599947, 64.85000000000000853 ) ) ;
#12059=AXIS2_PLACEMENT_3D ( 'NONE', #5503, #7811, #2186 ) ;
#12065=AXIS2_PLACEMENT_3D ( 'NONE', #11987, #13031, #4524 ) ;
#12070=DIRECTION ( 'NONE',  ( 0.000000000000000000, -1.000000000000000000, 0.000000000000000000 ) ) ;
#12071=CARTESIAN_POINT ( 'NONE',  ( -18.05918829504999934, 14.81548537210212046, 7.250000000000000000 ) ) ;
#12075=DIRECTION ( 'NONE',  ( 1.000000000000000000, 0.000000000000000000, 0.000000000000000000 ) ) ;
#12078=CARTESIAN_POINT ( 'NONE',  ( -35.05918829505000645, 27.97290950744599769, 83.57661607529820458 ) ) ;
#12080=VECTOR ( 'NONE', #5859, 1000.000000000000000 ) ;
#12081=AXIS2_PLACEMENT_3D ( 'NONE', #9208, #6259, #12412 ) ;
#12082=CIRCLE ( 'NONE', #1828, 17.00000000000000355 ) ;
#12083=ORIENTED_EDGE ( 'NONE', *, *, #13379, .T. ) ;
#12084=ORIENTED_EDGE ( 'NONE', *, *, #10678, .F. ) ;
#12085=PLANE ( 'NONE',  #7687 ) ;
#12088=MECHANICAL_DESIGN_GEOMETRIC_PRESENTATION_REPRESENTATION('',(#5833),#4072);
#12089=FACE_OUTER_BOUND ( 'NONE', #2813, .T. ) ;
#12091=LINE ( 'NONE', #12022, #195 ) ;
#12092=EDGE_CURVE ( 'NONE', #12928, #2900, #860, .T. ) ;
#12093=EDGE_CURVE ( 'NONE', #7102, #6443, #5226, .T. ) ;
#12094=CARTESIAN_POINT ( 'NONE',  ( -1.461186629049982422, 19.27191034044602347, 63.13003331700004850 ) ) ;
#12097=AXIS2_PLACEMENT_3D ( 'NONE', #8698, #11019, #2509 ) ;
#12099=ORIENTED_EDGE ( 'NONE', *, *, #13177, .F. ) ;
#12100=VERTEX_POINT ( 'NONE', #7308 ) ;
#12102=ORIENTED_EDGE ( 'NONE', *, *, #5707, .T. ) ;
#12105=ORIENTED_EDGE ( 'NONE', *, *, #4569, .T. ) ;
#12106=EDGE_LOOP ( 'NONE', ( #7055, #13630, #8828, #4866 ) ) ;
#12109=DIRECTION ( 'NONE',  ( 0.000000000000000000, 0.000000000000000000, 1.000000000000000000 ) ) ;
#12111=ORIENTED_EDGE ( 'NONE', *, *, #12153, .F. ) ;
#12113=AXIS2_PLACEMENT_3D ( 'NONE', #4789, #6031, #10308 ) ;
#12114=CARTESIAN_POINT ( 'NONE',  ( -10.38347696868452097, 26.08535324214045303, 61.65000000000000568 ) ) ;
#12116=FACE_OUTER_BOUND ( 'NONE', #10121, .T. ) ;
#12117=EDGE_CURVE ( 'NONE', #1633, #6090, #8311, .T. ) ;
#12119=AXIS2_PLACEMENT_3D ( 'NONE', #6856, #3727, #5038 ) ;
#12125=EDGE_CURVE ( 'NONE', #11930, #5595, #10447, .T. ) ;
#12126=CARTESIAN_POINT ( 'NONE',  ( -21.58198509594925341, 30.09164131411911924, 59.05576624416044496 ) ) ;
#12127=EDGE_LOOP ( 'NONE', ( #10362, #2318 ) ) ;
#12129=DIRECTION ( 'NONE',  ( 0.000000000000000000, 0.000000000000000000, 1.000000000000000000 ) ) ;
#12131=DIRECTION ( 'NONE',  ( 0.000000000000000000, 1.000000000000000000, 0.000000000000000000 ) ) ;
#12133=CARTESIAN_POINT ( 'NONE',  ( -35.05918829505000645, -6.027090492554000534, 68.85549045786049760 ) ) ;
#12141=VERTEX_POINT ( 'NONE', #902 ) ;
#12144=LINE ( 'NONE', #10974, #11767 ) ;
#12153=EDGE_CURVE ( 'NONE', #3976, #10337, #11593, .T. ) ;
#12155=ORIENTED_EDGE ( 'NONE', *, *, #12814, .T. ) ;
#12156=CYLINDRICAL_SURFACE ( 'NONE', #9497, 16.66282263685194920 ) ;
#12157=EDGE_LOOP ( 'NONE', ( #13197, #11512, #13042, #7004 ) ) ;
#12160=CARTESIAN_POINT ( 'NONE',  ( -0.5591882950499970084, 10.97290950744599947, 64.85000000000000853 ) ) ;
#12161=DIRECTION ( 'NONE',  ( 0.000000000000000000, 0.000000000000000000, -1.000000000000000000 ) ) ;
#12162=DIRECTION ( 'NONE',  ( 0.000000000000000000, -1.000000000000000000, 0.000000000000000000 ) ) ;
#12165=DIRECTION ( 'NONE',  ( 1.000000000000000000, 0.000000000000000000, 0.000000000000000000 ) ) ;
#12166=ORIENTED_EDGE ( 'NONE', *, *, #9622, .F. ) ;
#12167=EDGE_CURVE ( 'NONE', #10920, #1440, #5995, .T. ) ;
#12168=AXIS2_PLACEMENT_3D ( 'NONE', #3772, #5914, #1605 ) ;
#12169=CARTESIAN_POINT ( 'NONE',  ( -17.92774181590637284, 30.36027202460865126, 61.70913974837020533 ) ) ;
#12170=ORIENTED_EDGE ( 'NONE', *, *, #6435, .F. ) ;
#12171=ORIENTED_EDGE ( 'NONE', *, *, #12908, .F. ) ;
#12173=EDGE_LOOP ( 'NONE', ( #7779, #3307, #6272, #771 ) ) ;
#12174=CARTESIAN_POINT ( 'NONE',  ( -18.05918829504999934, 10.97290950744599947, 62.14999999999999858 ) ) ;
#12179=CARTESIAN_POINT ( 'NONE',  ( -18.05918829504999934, 10.97290950744599947, 27.09999999999999787 ) ) ;
#12180=CIRCLE ( 'NONE', #3706, 16.75000000000000355 ) ;
#12181=LINE ( 'NONE', #6794, #8467 ) ;
#12184=AXIS2_PLACEMENT_3D ( 'NONE', #7632, #913, #7983 ) ;
#12185=EDGE_CURVE ( 'NONE', #8674, #1279, #8653, .T. ) ;
#12186=CARTESIAN_POINT ( 'NONE',  ( -18.05918829504999934, 10.97290950744599947, 57.35000000000000142 ) ) ;
#12187=ORIENTED_EDGE ( 'NONE', *, *, #2361, .F. ) ;
#12190=CARTESIAN_POINT ( 'NONE',  ( -21.53863742889154409, 30.09823897630959522, 55.53674328751647948 ) ) ;
#12192=CARTESIAN_POINT ( 'NONE',  ( 1.629816981350590055, -4.941769416738769571, 17.25000000000000000 ) ) ;
#12195=DIRECTION ( 'NONE',  ( 1.000000000000000000, 0.000000000000000000, 0.000000000000000000 ) ) ;
#12200=EDGE_CURVE ( 'NONE', #12616, #6439, #5979, .T. ) ;
#12201=CARTESIAN_POINT ( 'NONE',  ( -15.34212233881444831, 16.32244711264754855, 60.04999999999999716 ) ) ;
#12203=DIRECTION ( 'NONE',  ( 0.000000000000000000, 0.000000000000000000, 1.000000000000000000 ) ) ;
#12204=DIRECTION ( 'NONE',  ( 0.6615960714621564875, -0.7498604124941129490, 0.000000000000000000 ) ) ;
#12208=DIRECTION ( 'NONE',  ( 0.000000000000000000, 0.000000000000000000, -1.000000000000000000 ) ) ;
#12209=DIRECTION ( 'NONE',  ( 0.000000000000000000, 0.000000000000000000, 1.000000000000000000 ) ) ;
#12210=VERTEX_POINT ( 'NONE', #8641 ) ;
#12211=DIRECTION ( 'NONE',  ( -1.000000000000000000, 0.000000000000000000, 0.000000000000000000 ) ) ;
#12212=CARTESIAN_POINT ( 'NONE',  ( -35.05918829505000645, -6.027090492554000534, 7.250000000000000000 ) ) ;
#12214=CARTESIAN_POINT ( 'NONE',  ( -18.05918829504999934, 10.97290950744599947, 60.04999999999999716 ) ) ;
#12216=AXIS2_PLACEMENT_3D ( 'NONE', #13166, #5889, #12466 ) ;
#12221=DIRECTION ( 'NONE',  ( 0.4528443260392608360, 0.8915896008669277339, 0.000000000000000000 ) ) ;
#12225=FACE_OUTER_BOUND ( 'NONE', #7287, .T. ) ;
#12227=CARTESIAN_POINT ( 'NONE',  ( -1.059188295049996231, 27.97290950744599769, 5.250000000000000000 ) ) ;
#12229=FACE_BOUND ( 'NONE', #4753, .T. ) ;
#12230=CARTESIAN_POINT ( 'NONE',  ( -18.05918829504999934, 10.97290950744599947, 67.84999999999999432 ) ) ;
#12231=DIRECTION ( 'NONE',  ( 1.000000000000000000, 0.000000000000000000, 0.000000000000000000 ) ) ;
#12233=TOROIDAL_SURFACE ( 'NONE', #11347, 10.00000000000000000, 2.000000000000000000 ) ;
#12234=AXIS2_PLACEMENT_3D ( 'NONE', #11317, #7110, #3087 ) ;
#12235=AXIS2_PLACEMENT_3D ( 'NONE', #4975, #3795, #10157 ) ;
#12237=CARTESIAN_POINT ( 'NONE',  ( -16.82673727123299301, 30.32761401379713817, 61.47513517491817936 ) ) ;
#12238=EDGE_LOOP ( 'NONE', ( #4984, #7121, #10334, #1701 ) ) ;
#12239=VERTEX_POINT ( 'NONE', #6486 ) ;
#12240=CARTESIAN_POINT ( 'NONE',  ( -18.05918829504999934, 10.97290950744599947, 30.59999999999999787 ) ) ;
#12241=VERTEX_POINT ( 'NONE', #6617 ) ;
#12242=DIRECTION ( 'NONE',  ( 0.000000000000000000, 0.000000000000000000, -1.000000000000000000 ) ) ;
#12248=DIRECTION ( 'NONE',  ( 1.000000000000000000, 0.000000000000000000, 0.000000000000000000 ) ) ;
#12249=ADVANCED_FACE ( 'NONE', ( #7656 ), #60, .F. ) ;
#12252=ADVANCED_FACE ( 'NONE', ( #9641 ), #121, .T. ) ;
#12255=ORIENTED_EDGE ( 'NONE', *, *, #10795, .T. ) ;
#12256=EDGE_CURVE ( 'NONE', #223, #1784, #7748, .T. ) ;
#12257=ORIENTED_EDGE ( 'NONE', *, *, #4279, .F. ) ;
#12261=CARTESIAN_POINT ( 'NONE',  ( -10.22585496205000055, 10.97290950744599947, 60.04999999999999716 ) ) ;
#12262=ORIENTED_EDGE ( 'NONE', *, *, #13673, .T. ) ;
#12264=CARTESIAN_POINT ( 'NONE',  ( -20.84908644685638279, 30.19213140065619783, 54.37388926677692780 ) ) ;
#12265=DIRECTION ( 'NONE',  ( 0.4528443260392608360, 0.8915896008669278450, 0.000000000000000000 ) ) ;
#12267=LINE ( 'NONE', #9324, #1276 ) ;
#12272=VERTEX_POINT ( 'NONE', #12981 ) ;
#12273=EDGE_CURVE ( 'NONE', #1420, #5251, #6201, .T. ) ;
#12275=DIRECTION ( 'NONE',  ( 0.6615960714621568206, -0.7498604124941125049, 0.000000000000000000 ) ) ;
#12276=CARTESIAN_POINT ( 'NONE',  ( 2.262399129208279902, 22.44393519180574970, 17.25000000000000000 ) ) ;
#12277=ORIENTED_EDGE ( 'NONE', *, *, #2732, .F. ) ;
#12280=CARTESIAN_POINT ( 'NONE',  ( -35.05918829505000645, 27.97290950744599769, 5.250000000000000000 ) ) ;
#12281=CARTESIAN_POINT ( 'NONE',  ( -28.87730642030694739, -7.867426463707980488, 17.25000000000000000 ) ) ;
#12282=AXIS2_PLACEMENT_3D ( 'NONE', #603, #11294, #537 ) ;
#12283=AXIS2_PLACEMENT_3D ( 'NONE', #9653, #7665, #1111 ) ;
#12284=CIRCLE ( 'NONE', #8261, 16.66282263685194920 ) ;
#12285=CARTESIAN_POINT ( 'NONE',  ( -22.21635405521520923, 13.97298182380577281, 68.75391885985828822 ) ) ;
#12287=AXIS2_PLACEMENT_3D ( 'NONE', #2250, #7798, #10493 ) ;
#12288=CARTESIAN_POINT ( 'NONE',  ( -35.05918829505000645, 27.97290950744599769, 64.35000000000000853 ) ) ;
#12292=DIRECTION ( 'NONE',  ( 0.000000000000000000, 0.000000000000000000, 1.000000000000000000 ) ) ;
#12294=EDGE_CURVE ( 'NONE', #11638, #3446, #9801, .T. ) ;
#12295=AXIS2_PLACEMENT_3D ( 'NONE', #7557, #11978, #11845 ) ;
#12298=VECTOR ( 'NONE', #2534, 1000.000000000000000 ) ;
#12301=PLANE ( 'NONE',  #13274 ) ;
#12302=VERTEX_POINT ( 'NONE', #10977 ) ;
#12304=CARTESIAN_POINT ( 'NONE',  ( -10.25088531517539892, 30.80589556422609832, 5.250000000000000000 ) ) ;
#12305=FACE_BOUND ( 'NONE', #1797, .T. ) ;
#12308=AXIS2_PLACEMENT_3D ( 'NONE', #9789, #1112, #5238 ) ;
#12310=AXIS2_PLACEMENT_3D ( 'NONE', #7540, #8471, #10857 ) ;
#12312=AXIS2_PLACEMENT_3D ( 'NONE', #175, #5414, #9691 ) ;
#12315=EDGE_CURVE ( 'NONE', #10428, #4952, #4746, .T. ) ;
#12316=VERTEX_POINT ( 'NONE', #277 ) ;
#12317=CARTESIAN_POINT ( 'NONE',  ( -1.059188295049996231, 27.97290950744599769, 64.35000000000000853 ) ) ;
#12320=ORIENTED_EDGE ( 'NONE', *, *, #350, .F. ) ;
#12322=VERTEX_POINT ( 'NONE', #3638 ) ;
#12325=CARTESIAN_POINT ( 'NONE',  ( -18.05918829504999934, 18.59295644444599915, 61.63595870800000398 ) ) ;
#12326=CARTESIAN_POINT ( 'NONE',  ( -12.26420230435512160, 9.417873376788568507, 68.84999999999999432 ) ) ;
#12327=CARTESIAN_POINT ( 'NONE',  ( 2.262399129208274573, -0.4981161769137525952, 83.57661607529820458 ) ) ;
#12328=DIRECTION ( 'NONE',  ( 0.000000000000000000, 0.000000000000000000, -1.000000000000000000 ) ) ;
#12329=CARTESIAN_POINT ( 'NONE',  ( -38.38077571930825371, -0.4981161769137670281, 17.25000000000000000 ) ) ;
#12330=CARTESIAN_POINT ( 'NONE',  ( -18.05918829504999934, 10.97290950744599947, 64.85000000000000853 ) ) ;
#12331=CIRCLE ( 'NONE', #6064, 17.00000000000000000 ) ;
#12334=ORIENTED_EDGE ( 'NONE', *, *, #206, .F. ) ;
#12335=EDGE_CURVE ( 'NONE', #3979, #11332, #13048, .T. ) ;
#12337=ORIENTED_EDGE ( 'NONE', *, *, #9533, .T. ) ;
#12340=CARTESIAN_POINT ( 'NONE',  ( -19.63224265096508958, 30.30694957903927644, 61.32011773191905490 ) ) ;
#12341=FACE_OUTER_BOUND ( 'NONE', #8337, .T. ) ;
#12342=DIRECTION ( 'NONE',  ( 0.000000000000000000, 0.000000000000000000, 1.000000000000000000 ) ) ;
#12343=CARTESIAN_POINT ( 'NONE',  ( -18.05918829504999934, 10.97290950744599947, 68.84999999999999432 ) ) ;
#12345=AXIS2_PLACEMENT_3D ( 'NONE', #9466, #5255, #10579 ) ;
#12348=CARTESIAN_POINT ( 'NONE',  ( -23.24102627739274851, -6.265087914666289670, 62.14999999999999858 ) ) ;
#12349=ORIENTED_EDGE ( 'NONE', *, *, #8220, .T. ) ;
#12351=DIRECTION ( 'NONE',  ( 0.000000000000000000, 0.000000000000000000, 1.000000000000000000 ) ) ;
#12353=DIRECTION ( 'NONE',  ( 0.000000000000000000, 0.000000000000000000, -1.000000000000000000 ) ) ;
#12354=AXIS2_PLACEMENT_3D ( 'NONE', #7257, #124, #10823 ) ;
#12357=CARTESIAN_POINT ( 'NONE',  ( -35.05918829505000645, 27.97290950744599769, 64.35000000000000853 ) ) ;
#12360=CARTESIAN_POINT ( 'NONE',  ( -24.20502162805000168, 10.97290950744599947, 60.60999999999999943 ) ) ;
#12361=DIRECTION ( 'NONE',  ( 0.000000000000000000, 0.000000000000000000, -1.000000000000000000 ) ) ;
#12362=EDGE_LOOP ( 'NONE', ( #5422, #6987, #8271, #12655, #1621, #4722, #5402, #1242 ) ) ;
#12364=CARTESIAN_POINT ( 'NONE',  ( -37.75918829505000218, 27.97290950744599769, 58.85000000000000142 ) ) ;
#12365=ORIENTED_EDGE ( 'NONE', *, *, #10553, .T. ) ;
#12371=DIRECTION ( 'NONE',  ( 0.3984948954980490621, -4.880154982482439852E-17, 0.9171705502587831349 ) ) ;
#12372=EDGE_CURVE ( 'NONE', #11621, #11264, #3763, .T. ) ;
#12373=CARTESIAN_POINT ( 'NONE',  ( -38.38077571930825371, 22.44393519180574970, 5.250000000000000000 ) ) ;
#12375=CARTESIAN_POINT ( 'NONE',  ( -35.05918829505000645, -6.027090492554000534, 83.57661607529820458 ) ) ;
#12376=ORIENTED_EDGE ( 'NONE', *, *, #7438, .F. ) ;
#12377=EDGE_CURVE ( 'NONE', #4651, #12584, #9110, .T. ) ;
#12378=ORIENTED_EDGE ( 'NONE', *, *, #9365, .T. ) ;
#12379=CARTESIAN_POINT ( 'NONE',  ( -17.59482673585142365, 30.35570588519015445, 61.67721350625757282 ) ) ;
#12381=CARTESIAN_POINT ( 'NONE',  ( -18.05918829505000645, 3.394200320306482332, 61.95399527338132373 ) ) ;
#12385=ORIENTED_EDGE ( 'NONE', *, *, #11252, .T. ) ;
#12386=ADVANCED_FACE ( 'NONE', ( #2664 ), #2884, .F. ) ;
#12387=DIRECTION ( 'NONE',  ( 0.000000000000000000, 0.000000000000000000, 1.000000000000000000 ) ) ;
#12389=LINE ( 'NONE', #7062, #876 ) ;
#12391=AXIS2_PLACEMENT_3D ( 'NONE', #4703, #10150, #3788 ) ;
#12393=ORIENTED_EDGE ( 'NONE', *, *, #9126, .T. ) ;
#12396=CYLINDRICAL_SURFACE ( 'NONE', #1748, 24.92993838181874722 ) ;
#12397=ADVANCED_FACE ( 'NONE', ( #5638 ), #3492, .T. ) ;
#12398=DIRECTION ( 'NONE',  ( 1.000000000000000000, 0.000000000000000000, 0.000000000000000000 ) ) ;
#12399=CARTESIAN_POINT ( 'NONE',  ( -32.35918829505000360, -6.027090492554000534, 7.250000000000000000 ) ) ;
#12400=DIRECTION ( 'NONE',  ( 0.000000000000000000, -2.202823461557850341E-15, 1.000000000000000000 ) ) ;
#12404=ADVANCED_FACE ( 'NONE', ( #2533 ), #9002, .T. ) ;
#12407=CARTESIAN_POINT ( 'NONE',  ( -28.87730642030694739, -7.867426463707978712, 83.57661607529820458 ) ) ;
#12410=DIRECTION ( 'NONE',  ( 0.6615960714621565986, -0.7498604124941128379, 0.000000000000000000 ) ) ;
#12411=DIRECTION ( 'NONE',  ( -1.000000000000000000, 0.000000000000000000, 0.000000000000000000 ) ) ;
#12412=DIRECTION ( 'NONE',  ( 1.000000000000000000, 0.000000000000000000, 0.000000000000000000 ) ) ;
#12416=FACE_OUTER_BOUND ( 'NONE', #10217, .T. ) ;
#12417=CIRCLE ( 'NONE', #3943, 8.300000000000000711 ) ;
#12418=DIRECTION ( 'NONE',  ( 0.000000000000000000, 0.000000000000000000, 1.000000000000000000 ) ) ;
#12419=EDGE_CURVE ( 'NONE', #9316, #10219, #341, .T. ) ;
#12423=EDGE_LOOP ( 'NONE', ( #11565, #7552 ) ) ;
#12425=DIRECTION ( 'NONE',  ( 0.000000000000000000, 0.000000000000000000, 1.000000000000000000 ) ) ;
#12427=ORIENTED_EDGE ( 'NONE', *, *, #13592, .T. ) ;
#12428=CARTESIAN_POINT ( 'NONE',  ( -20.73856204053882735, 15.27682634614306600, 68.78022907841716460 ) ) ;
#12433=DIRECTION ( 'NONE',  ( -1.000000000000000000, 0.000000000000000000, 0.000000000000000000 ) ) ;
#12434=EDGE_CURVE ( 'NONE', #5647, #6318, #407, .T. ) ;
#12435=DIRECTION ( 'NONE',  ( 1.000000000000000000, 0.000000000000000000, 0.000000000000000000 ) ) ;
#12438=CARTESIAN_POINT ( 'NONE',  ( -14.84085382869762881, 30.13625835401696307, 59.70232134295659421 ) ) ;
#12439=CIRCLE ( 'NONE', #8645, 34.69999999999999574 ) ;
#12441=EDGE_LOOP ( 'NONE', ( #3502, #4015, #7116, #13351, #10665, #790, #2261, #3878, #11733, #8916, #702, #3975, #1686, #4969, #4816 ) ) ;
#12442=CIRCLE ( 'NONE', #2431, 16.00000000000000000 ) ;
#12443=SURFACE_STYLE_USAGE ( .BOTH. , #13423 ) ;
#12445=EDGE_LOOP ( 'NONE', ( #10294, #4863, #6786, #4264 ) ) ;
#12446=ORIENTED_EDGE ( 'NONE', *, *, #13140, .F. ) ;
#12447=CARTESIAN_POINT ( 'NONE',  ( -14.08961186627706041, 6.473747032481329988, 68.84999999999999432 ) ) ;
#12451=CARTESIAN_POINT ( 'NONE',  ( -16.59761566455133774, 27.91013588845822468, 57.74153177338070009 ) ) ;
#12453=DIRECTION ( 'NONE',  ( 0.4528443260392608916, 0.8915896008669277339, 0.000000000000000000 ) ) ;
#12454=CIRCLE ( 'NONE', #8880, 6.145833333000000565 ) ;
#12455=AXIS2_PLACEMENT_3D ( 'NONE', #1172, #11873, #10892 ) ;
#12457=EDGE_CURVE ( 'NONE', #7434, #11514, #13774, .T. ) ;
#12458=EDGE_LOOP ( 'NONE', ( #9993, #8352, #6467, #11912, #11997 ) ) ;
#12459=EDGE_CURVE ( 'NONE', #651, #7262, #1524, .T. ) ;
#12461=ORIENTED_EDGE ( 'NONE', *, *, #1540, .T. ) ;
#12466=DIRECTION ( 'NONE',  ( 1.000000000000000000, 0.000000000000000000, 0.000000000000000000 ) ) ;
#12467=CARTESIAN_POINT ( 'NONE',  ( -20.58011868346011042, 30.22311051615698929, 60.62245744008113491 ) ) ;
#12468=CARTESIAN_POINT ( 'NONE',  ( -18.05918829504999934, 10.97290950744599947, 60.60999999999999943 ) ) ;
#12473=EDGE_LOOP ( 'NONE', ( #6296, #5816 ) ) ;
#12477=ORIENTED_EDGE ( 'NONE', *, *, #2127, .F. ) ;
#12478=ORIENTED_EDGE ( 'NONE', *, *, #12613, .F. ) ;
#12479=CARTESIAN_POINT ( 'NONE',  ( -10.79835982676942052, -4.028726038184999858, 62.14999999999999858 ) ) ;
#12481=DIRECTION ( 'NONE',  ( 0.4528443260392608916, 0.8915896008669277339, 0.000000000000000000 ) ) ;
#12482=CARTESIAN_POINT ( 'NONE',  ( -10.38347696868452097, 26.08535324214045303, 57.35000000000000142 ) ) ;
#12483=DIRECTION ( 'NONE',  ( 0.000000000000000000, 0.000000000000000000, 1.000000000000000000 ) ) ;
#12489=CIRCLE ( 'NONE', #13154, 6.450000000000009948 ) ;
#12492=AXIS2_PLACEMENT_3D ( 'NONE', #3989, #6979, #10405 ) ;
#12494=ORIENTED_EDGE ( 'NONE', *, *, #2482, .T. ) ;
#12496=EDGE_CURVE ( 'NONE', #1821, #11264, #3316, .T. ) ;
#12499=CARTESIAN_POINT ( 'NONE',  ( -21.25890827522755089, 14.81772886755349639, 68.85000000000002274 ) ) ;
#12500=DIRECTION ( 'NONE',  ( 1.000000000000000000, 0.000000000000000000, 0.000000000000000000 ) ) ;
#12501=FACE_OUTER_BOUND ( 'NONE', #2560, .T. ) ;
#12502=DIRECTION ( 'NONE',  ( 0.000000000000000000, 0.000000000000000000, -1.000000000000000000 ) ) ;
#12504=CARTESIAN_POINT ( 'NONE',  ( -35.05918829505000645, -6.027090492554000534, 64.85000000000000853 ) ) ;
#12505=VECTOR ( 'NONE', #8786, 1000.000000000000114 ) ;
#12506=AXIS2_PLACEMENT_3D ( 'NONE', #2755, #9071, #1742 ) ;
#12507=AXIS2_PLACEMENT_3D ( 'NONE', #3299, #2128, #1989 ) ;
#12509=EDGE_LOOP ( 'NONE', ( #4705, #4971, #4122, #1638 ) ) ;
#12510=CARTESIAN_POINT ( 'NONE',  ( -14.39336303962373975, 30.06926057631024918, 56.09279642605752514 ) ) ;
#12511=EDGE_LOOP ( 'NONE', ( #3532, #9724 ) ) ;
#12513=EDGE_LOOP ( 'NONE', ( #2570, #6158, #3484, #8499 ) ) ;
#12516=DIRECTION ( 'NONE',  ( 0.3202092937642119774, 0.6304490528084089052, 0.7071067811865507924 ) ) ;
#12517=CIRCLE ( 'NONE', #6492, 17.00000000000000355 ) ;
#12518=FACE_OUTER_BOUND ( 'NONE', #12032, .T. ) ;
#12519=CIRCLE ( 'NONE', #13182, 8.300000000000000711 ) ;
#12521=ADVANCED_FACE ( 'NONE', ( #1808 ), #6113, .F. ) ;
#12522=CARTESIAN_POINT ( 'NONE',  ( -18.05918829504999934, 10.97290950744599947, 64.35000000000000853 ) ) ;
#12523=FACE_OUTER_BOUND ( 'NONE', #12173, .T. ) ;
#12525=FACE_OUTER_BOUND ( 'NONE', #2784, .T. ) ;
#12526=DIRECTION ( 'NONE',  ( 1.000000000000000000, 0.000000000000000000, 0.000000000000000000 ) ) ;
#12527=CARTESIAN_POINT ( 'NONE',  ( -25.86749127492454647, -8.860076549334129581, 17.25000000000000000 ) ) ;
#12529=FACE_OUTER_BOUND ( 'NONE', #6843, .T. ) ;
#12530=CIRCLE ( 'NONE', #1367, 16.72262947720610171 ) ;
#12532=CIRCLE ( 'NONE', #5826, 16.75000000000000355 ) ;
#12536=ORIENTED_EDGE ( 'NONE', *, *, #2326, .F. ) ;
#12537=EDGE_LOOP ( 'NONE', ( #1260, #4973, #2569, #7302 ) ) ;
#12538=ORIENTED_EDGE ( 'NONE', *, *, #714, .T. ) ;
#12539=DIRECTION ( 'NONE',  ( 0.000000000000000000, 0.000000000000000000, -1.000000000000000000 ) ) ;
#12540=CARTESIAN_POINT ( 'NONE',  ( -19.61957230515337969, 30.30780693223203670, 61.32664748691393442 ) ) ;
#12541=VECTOR ( 'NONE', #13742, 1000.000000000000000 ) ;
#12544=LINE ( 'NONE', #4857, #4638 ) ;
#12545=DIRECTION ( 'NONE',  ( 0.000000000000000000, 0.000000000000000000, -1.000000000000000000 ) ) ;
#12546=ADVANCED_FACE ( 'NONE', ( #9137 ), #10386, .T. ) ;
#12552=DIRECTION ( 'NONE',  ( 0.000000000000000000, 0.000000000000000000, -1.000000000000000000 ) ) ;
#12557=DIRECTION ( 'NONE',  ( 0.000000000000000000, 0.000000000000000000, -1.000000000000000000 ) ) ;
#12560=CARTESIAN_POINT ( 'NONE',  ( -34.05918829504999934, 10.97290950744599947, 7.250000000000000000 ) ) ;
#12562=DIRECTION ( 'NONE',  ( 0.9576665234506833713, -0.2878798879079291217, 0.000000000000000000 ) ) ;
#12564=DIRECTION ( 'NONE',  ( -0.4528443260392610026, -0.8915896008669278450, 0.000000000000000000 ) ) ;
#12567=ORIENTED_EDGE ( 'NONE', *, *, #2816, .T. ) ;
#12569=CIRCLE ( 'NONE', #5864, 6.049999999999999822 ) ;
#12571=DIRECTION ( 'NONE',  ( 0.000000000000000000, 0.000000000000000000, -1.000000000000000000 ) ) ;
#12573=CARTESIAN_POINT ( 'NONE',  ( -21.36716865236079954, 14.72221156991656166, 68.84999999999999432 ) ) ;
#12578=CARTESIAN_POINT ( 'NONE',  ( -29.51816008892539855, -2.179141222803619993, 62.14999999999999858 ) ) ;
#12579=CIRCLE ( 'NONE', #5643, 6.595833333000001630 ) ;
#12580=EDGE_CURVE ( 'NONE', #6443, #12635, #7766, .T. ) ;
#12582=CARTESIAN_POINT ( 'NONE',  ( -14.42071735626405093, 30.07360145807300000, 55.99350896921582432 ) ) ;
#12583=VERTEX_POINT ( 'NONE', #10192 ) ;
#12584=VERTEX_POINT ( 'NONE', #10264 ) ;
#12586=DIRECTION ( 'NONE',  ( 0.000000000000000000, 0.000000000000000000, 1.000000000000000000 ) ) ;
#12587=CARTESIAN_POINT ( 'NONE',  ( -1.059188295049996231, -6.027090492554000534, 64.85000000000000853 ) ) ;
#12592=ORIENTED_EDGE ( 'NONE', *, *, #3088, .F. ) ;
#12594=LINE ( 'NONE', #6226, #3874 ) ;
#12595=CARTESIAN_POINT ( 'NONE',  ( -18.97946290528394186, 27.94856484295734234, 58.55107660166387262 ) ) ;
#12596=STYLED_ITEM ( 'NONE', ( #3537 ), #229 ) ;
#12597=LINE ( 'NONE', #7395, #3373 ) ;
#12598=EDGE_CURVE ( 'NONE', #1146, #759, #4946, .T. ) ;
#12604=CARTESIAN_POINT ( 'NONE',  ( -18.99164311995750865, 26.94578616932480486, 56.17493374376507376 ) ) ;
#12607=CIRCLE ( 'NONE', #11487, 7.166108729582679970 ) ;
#12610=ORIENTED_EDGE ( 'NONE', *, *, #9594, .T. ) ;
#12613=EDGE_CURVE ( 'NONE', #2730, #1970, #13522, .T. ) ;
#12614=VECTOR ( 'NONE', #12425, 1000.000000000000000 ) ;
#12616=VERTEX_POINT ( 'NONE', #2159 ) ;
#12618=CARTESIAN_POINT ( 'NONE',  ( -24.20502162805000168, 10.97290950744599947, 60.60999999999999943 ) ) ;
#12620=FACE_OUTER_BOUND ( 'NONE', #2134, .T. ) ;
#12622=VERTEX_POINT ( 'NONE', #7362 ) ;
#12625=DIRECTION ( 'NONE',  ( 0.000000000000000000, -1.000000000000000000, 0.000000000000000000 ) ) ;
#12626=CARTESIAN_POINT ( 'NONE',  ( -18.05918829504999934, 10.97290950744599947, 60.04999999999999716 ) ) ;
#12627=( NAMED_UNIT ( * ) SI_UNIT ( $, .STERADIAN. ) SOLID_ANGLE_UNIT ( ) );
#12628=EDGE_CURVE ( 'NONE', #5559, #8370, #3120, .T. ) ;
#12629=VECTOR ( 'NONE', #4443, 1000.000000000000114 ) ;
#12631=EDGE_CURVE ( 'NONE', #7318, #4114, #1756, .T. ) ;
#12632=EDGE_CURVE ( 'NONE', #12239, #5283, #8426, .T. ) ;
#12633=ORIENTED_EDGE ( 'NONE', *, *, #11225, .F. ) ;
#12635=VERTEX_POINT ( 'NONE', #6396 ) ;
#12637=ORIENTED_EDGE ( 'NONE', *, *, #12780, .T. ) ;
#12638=DIRECTION ( 'NONE',  ( 0.000000000000000000, 0.000000000000000000, -1.000000000000000000 ) ) ;
#12639=ORIENTED_EDGE ( 'NONE', *, *, #2598, .F. ) ;
#12640=VECTOR ( 'NONE', #3035, 1000.000000000000114 ) ;
#12642=DIRECTION ( 'NONE',  ( 1.000000000000000000, 0.000000000000000000, 0.000000000000000000 ) ) ;
#12645=CIRCLE ( 'NONE', #4178, 4.750000000000000888 ) ;
#12646=EDGE_CURVE ( 'NONE', #2414, #8660, #9564, .T. ) ;
#12647=CARTESIAN_POINT ( 'NONE',  ( -14.58337460918420980, 30.09884447278222197, 55.52393896758509584 ) ) ;
#12648=ORIENTED_EDGE ( 'NONE', *, *, #2968, .T. ) ;
#12649=VERTEX_POINT ( 'NONE', #10662 ) ;
#12650=ORIENTED_EDGE ( 'NONE', *, *, #6812, .T. ) ;
#12653=CLOSED_SHELL ( 'NONE', ( #1526, #12011, #13283, #7751, #3290, #10985, #6544, #7453, #5654, #5454, #10551, #8964, #11603, #11814, #10880, #406, #7047, #10381, #3230 ) ) ;
#12654=CARTESIAN_POINT ( 'NONE',  ( -34.72201093190195564, 10.97290950744599947, 6.250000000000000000 ) ) ;
#12655=ORIENTED_EDGE ( 'NONE', *, *, #5883, .T. ) ;
#12658=AXIS2_PLACEMENT_3D ( 'NONE', #11785, #1234, #1031 ) ;
#12659=CARTESIAN_POINT ( 'NONE',  ( -28.87730642030695094, 29.81324547859994922, 17.25000000000000000 ) ) ;
#12660=CARTESIAN_POINT ( 'NONE',  ( -17.86151640326295365, 27.97292178005357499, 58.85016477904981258 ) ) ;
#12664=ORIENTED_EDGE ( 'NONE', *, *, #5332, .F. ) ;
#12672=CONICAL_SURFACE ( 'NONE', #11561, 6.850000000000002309, 0.7853981633974433940 ) ;
#12673=CARTESIAN_POINT ( 'NONE',  ( -18.33386804087177779, 26.97094072739188064, 55.86735471292099930 ) ) ;
#12674=AXIS2_PLACEMENT_3D ( 'NONE', #1435, #3619, #385 ) ;
#12675=DIRECTION ( 'NONE',  ( 0.000000000000000000, -1.000000000000000000, 0.000000000000000000 ) ) ;
#12676=DIRECTION ( 'NONE',  ( -1.000000000000000000, 0.000000000000000000, 0.000000000000000000 ) ) ;
#12678=DIRECTION ( 'NONE',  ( 1.000000000000000000, 0.000000000000000000, 0.000000000000000000 ) ) ;
#12680=COLOUR_RGB ( '', 0.66274510, 0.83137255, 0.94901961) ;
#12681=AXIS2_PLACEMENT_3D ( 'NONE', #12212, #11099, #12075 ) ;
#12686=DIRECTION ( 'NONE',  ( -1.000000000000000000, 0.000000000000000000, 0.000000000000000000 ) ) ;
#12688=CARTESIAN_POINT ( 'NONE',  ( -18.05918829504999934, 10.97290950744599947, 57.35000000000000142 ) ) ;
#12689=DIRECTION ( 'NONE',  ( 0.000000000000000000, 0.000000000000000000, -1.000000000000000000 ) ) ;
#12690=DIRECTION ( 'NONE',  ( 0.000000000000000000, 0.000000000000000000, -1.000000000000000000 ) ) ;
#12695=DIRECTION ( 'NONE',  ( -0.9496839325805410681, 0.3132098788326420080, 0.000000000000000000 ) ) ;
#12700=ORIENTED_EDGE ( 'NONE', *, *, #10117, .T. ) ;
#12701=LINE ( 'NONE', #8504, #8155 ) ;
#12703=ORIENTED_EDGE ( 'NONE', *, *, #3714, .F. ) ;
#12706=CARTESIAN_POINT ( 'NONE',  ( -1.336558817843898073, 10.00028003023991907, 62.14999999999999858 ) ) ;
#12707=AXIS2_PLACEMENT_3D ( 'NONE', #4980, #13432, #925 ) ;
#12709=CARTESIAN_POINT ( 'NONE',  ( -15.94576320551015236, 6.169660524810645086, 68.60247846904903213 ) ) ;
#12710=CIRCLE ( 'NONE', #10934, 2.700000000000001066 ) ;
#12711=DIRECTION ( 'NONE',  ( -1.000000000000000000, 0.000000000000000000, 0.000000000000000000 ) ) ;
#12712=EDGE_CURVE ( 'NONE', #7844, #13212, #2003, .T. ) ;
#12714=AXIS2_PLACEMENT_3D ( 'NONE', #4160, #8409, #12678 ) ;
#12715=ORIENTED_EDGE ( 'NONE', *, *, #8899, .F. ) ;
#12716=B_SPLINE_CURVE_WITH_KNOTS ( 'NONE', 3,
 ( #7894, #12169, #11263, #12379, #4626, #1550, #1685, #5926, #6918, #2620, #8886, #12237, #2693, #3589, #10086, #9023, #508, #7826, #6846, #11124, #13276, #11192, #10215, #635, #13419, #3864, #8114, #6721, #1972, #1835, #9236, #13686, #6073, #1760, #11462, #6004, #3033, #2970, #13486, #6212, #4970, #9501, #10288, #4132, #700, #3927, #7185, #8317, #10409, #7246, #8383, #8174, #12438, #7316, #10555, #10482, #5102, #1898, #910, #2898, #13746, #13618, #6138, #9441, #11600, #7117, #7050, #4073, #984, #8450, #11525, #12510, #12582, #834, #773, #5171, #11394, #9370, #12647, #3094, #2051, #6294, #5233, #4201, #13547, #2827, #11324, #10348, #5030, #9300, #3999, #8247, #9781, #6418, #12782, #4476, #3362, #12838, #11673, #8731, #6354, #10829, #131, #5499, #10691, #4276, #6625, #2181, #8581, #1321, #8519, #3233, #1247, #11881, #2258, #12717, #12913, #10763, #9711, #5435, #204, #8648, #1107, #1180, #7593, #2334, #7442, #4401, #10619, #12989, #3437, #7663, #5575, #11946, #4548, #6496, #9865, #6561, #2400, #10901, #288 ),
 .UNSPECIFIED., .F., .F.,
 ( 4, 2, 1, 1, 2, 2, 2, 2, 1, 1, 2, 2, 2, 2, 1, 1, 1, 2, 2, 2, 2, 2, 2, 2, 1, 1, 2, 2, 2, 2, 1, 1, 2, 2, 2, 2, 1, 2, 2, 2, 2, 2, 1, 1, 2, 2, 2, 2, 1, 1, 2, 2, 2, 2, 1, 1, 1, 1, 2, 2, 2, 2, 1, 1, 2, 2, 2, 2, 1, 1, 2, 2, 2, 2, 1, 1, 2, 2, 2, 2, 1, 2, 2, 4 ),
 ( 0.000000000000000000, 0.03125000000000808381, 0.04687500000001171285, 0.05468750000001329492, 0.05859375000001391248, 0.06250000000001453004, 0.09375000000002493838, 0.1093750000000304895, 0.1171875000000335981, 0.1210937500000347916, 0.1230468750000347222, 0.1250000000000346390, 0.1562500000000229816, 0.1718750000000167089, 0.1796875000000135725, 0.1835937500000119627, 0.1855468750000118794, 0.1865234375000117961, 0.1875000000000117129, 0.2031250000000025535, 0.2109374999999971134, 0.2187499999999916733, 0.2343749999999801548, 0.2421874999999742706, 0.2460937499999713562, 0.2480468749999690525, 0.2490234374999678868, 0.2499999999999667211, 0.2812499999999455436, 0.2968749999999342193, 0.3046874999999286127, 0.3085937499999257261, 0.3105468749999242828, 0.3124999999999228395, 0.3437499999998901434, 0.3593749999998738787, 0.3671874999998657740, 0.3710937499998609446, 0.3749999999998561151, 0.4999999999997231659, 0.5624999999996567190, 0.5937499999996241895, 0.6093749999996073141, 0.6171874999995996536, 0.6210937499995951017, 0.6249999999995905497, 0.6562499999995563549, 0.6718749999995385913, 0.6796874999995304867, 0.6835937499995262678, 0.6855468749995233813, 0.6874999999995206057, 0.7187499999994910738, 0.7343749999994761968, 0.7421874999994693134, 0.7460937499994665378, 0.7480468749994652056, 0.7490234374994638733, 0.7495117187494632072, 0.7499999999994625410, 0.7656249999995053956, 0.7734374999995261568, 0.7773437499995370370, 0.7792968749995425881, 0.7802734374995453637, 0.7812499999995481392, 0.7968749999995949906, 0.8046874999996184163, 0.8085937499996297406, 0.8105468749996348476, 0.8115234374996367350, 0.8124999999996386224, 0.8437499999997121192, 0.8593749999997484235, 0.8671874999997662981, 0.8710937499997747357, 0.8730468749997783995, 0.8749999999997821742, 0.9062499999998400169, 0.9218749999998684386, 0.9296874999998825384, 0.9335937499998891997, 0.9374999999998958611, 1.000000000000000000 ),
 .UNSPECIFIED. ) ;
#12717=CARTESIAN_POINT ( 'NONE',  ( -15.82084781710581289, 30.25218297716627092, 53.82068884647250684 ) ) ;
#12718=ORIENTED_EDGE ( 'NONE', *, *, #8159, .T. ) ;
#12721=ORIENTED_EDGE ( 'NONE', *, *, #7155, .T. ) ;
#12722=DIRECTION ( 'NONE',  ( -1.000000000000000000, 0.000000000000000000, 0.000000000000000000 ) ) ;
#12723=CARTESIAN_POINT ( 'NONE',  ( -10.38347696868452097, 26.08535324214045303, 60.85000000000000142 ) ) ;
#12725=DIRECTION ( 'NONE',  ( 0.000000000000000000, 0.000000000000000000, 1.000000000000000000 ) ) ;
#12726=CARTESIAN_POINT ( 'NONE',  ( 2.262399129208274129, 22.44393519180576746, 83.57661607529820458 ) ) ;
#12727=AXIS2_PLACEMENT_3D ( 'NONE', #12758, #1935, #10529 ) ;
#12728=AXIS2_PLACEMENT_3D ( 'NONE', #3707, #11314, #7884 ) ;
#12729=AXIS2_PLACEMENT_3D ( 'NONE', #3375, #9934, #10993 ) ;
#12731=CARTESIAN_POINT ( 'NONE',  ( 0.09777679598749940137, 23.36596564213564875, 64.85000000000000853 ) ) ;
#12732=EDGE_CURVE ( 'NONE', #1952, #5721, #4664, .T. ) ;
#12733=FACE_OUTER_BOUND ( 'NONE', #1769, .T. ) ;
#12734=ORIENTED_EDGE ( 'NONE', *, *, #12496, .F. ) ;
#12737=AXIS2_PLACEMENT_3D ( 'NONE', #4047, #12562, #8497 ) ;
#12740=ORIENTED_EDGE ( 'NONE', *, *, #6002, .T. ) ;
#12741=DIRECTION ( 'NONE',  ( 0.000000000000000000, 0.000000000000000000, 1.000000000000000000 ) ) ;
#12744=CARTESIAN_POINT ( 'NONE',  ( -36.21615338608749823, -1.420146627243662030, 68.85549045786049760 ) ) ;
#12745=FACE_OUTER_BOUND ( 'NONE', #9245, .T. ) ;
#12748=DIRECTION ( 'NONE',  ( 0.3132098788326400096, -0.9496839325805418452, 0.000000000000000000 ) ) ;
#12749=AXIS2_PLACEMENT_3D ( 'NONE', #11679, #2121, #11736 ) ;
#12750=( BOUNDED_SURFACE ( )  B_SPLINE_SURFACE ( 3, 3, ( 
 ( #9736, #10142, #7953, #6910 ),
 ( #1677, #10079, #626, #9157 ),
 ( #237, #6584, #10859, #2820 ),
 ( #5922, #2427, #8684, #1749 ) ),
 .UNSPECIFIED., .F., .F., .F. ) 
 B_SPLINE_SURFACE_WITH_KNOTS ( ( 4, 4 ),
 ( 4, 4 ),
 ( 0.000000000000000000, 1.000000000000000000 ),
 ( 0.000000000000000000, 1.000000000000000000 ),
 .UNSPECIFIED. ) 
 GEOMETRIC_REPRESENTATION_ITEM ( )  RATIONAL_B_SPLINE_SURFACE ( (
 ( 1.000000000000000000, 0.3333333333333329818, 0.3333333333333329818, 1.000000000000000000),
 ( 0.7553208711179729695, 0.2517736237059909898, 0.2517736237059909898, 0.7553208711179729695),
 ( 0.7553208711179729695, 0.2517736237059909898, 0.2517736237059909898, 0.7553208711179729695),
 ( 1.000000000000000000, 0.3333333333333329818, 0.3333333333333329818, 1.000000000000000000) ) ) 
 REPRESENTATION_ITEM ( '' )  SURFACE ( )  );
#12755=AXIS2_PLACEMENT_3D ( 'NONE', #6892, #4744, #11160 ) ;
#12758=CARTESIAN_POINT ( 'NONE',  ( -1.059188295049996231, -6.027090492554000534, 7.250000000000000000 ) ) ;
#12759=CARTESIAN_POINT ( 'NONE',  ( -20.31679026759186613, 30.25033400041233733, 53.83638459472079774 ) ) ;
#12761=DIRECTION ( 'NONE',  ( -1.000000000000000000, 0.000000000000000000, 0.000000000000000000 ) ) ;
#12762=CARTESIAN_POINT ( 'NONE',  ( -22.02876472382295248, 15.47207198241065029, 31.09999999999999787 ) ) ;
#12764=ORIENTED_EDGE ( 'NONE', *, *, #13528, .T. ) ;
#12765=DIRECTION ( 'NONE',  ( 0.000000000000000000, 0.000000000000000000, -1.000000000000000000 ) ) ;
#12768=EDGE_LOOP ( 'NONE', ( #13535, #13092, #10682, #1414 ) ) ;
#12769=VERTEX_POINT ( 'NONE', #8496 ) ;
#12771=LINE ( 'NONE', #9697, #5676 ) ;
#12773=VERTEX_POINT ( 'NONE', #12762 ) ;
#12774=CARTESIAN_POINT ( 'NONE',  ( -13.41866240927501508, 8.399302110258624054, 68.54361232608823684 ) ) ;
#12775=AXIS2_PLACEMENT_3D ( 'NONE', #11423, #3742, #11219 ) ;
#12777=DIRECTION ( 'NONE',  ( 0.7071067811865489050, 0.000000000000000000, -0.7071067811865460184 ) ) ;
#12780=EDGE_CURVE ( 'NONE', #1687, #10704, #3209, .T. ) ;
#12781=AXIS2_PLACEMENT_3D ( 'NONE', #11408, #9032, #12248 ) ;
#12782=CARTESIAN_POINT ( 'NONE',  ( -15.25210833619480510, 30.19004818236263077, 54.39484650223464257 ) ) ;
#12785=CARTESIAN_POINT ( 'NONE',  ( -18.05918829504999934, 10.97290950744599947, 68.84999999999999432 ) ) ;
#12786=EDGE_CURVE ( 'NONE', #999, #8284, #7781, .T. ) ;
#12787=DIRECTION ( 'NONE',  ( -1.000000000000000000, 0.000000000000000000, 0.000000000000000000 ) ) ;
#12788=( NAMED_UNIT ( * ) SI_UNIT ( $, .STERADIAN. ) SOLID_ANGLE_UNIT ( ) );
#12791=LINE ( 'NONE', #12726, #4885 ) ;
#12793=CARTESIAN_POINT ( 'NONE',  ( -18.05918829504999934, 2.892876190446000084, 63.34900083300000517 ) ) ;
#12794=CARTESIAN_POINT ( 'NONE',  ( -5.631644894983189431, 10.97290950744599947, 73.76763816269230745 ) ) ;
#12797=CYLINDRICAL_SURFACE ( 'NONE', #3248, 4.749999999999997335 ) ;
#12798=ORIENTED_EDGE ( 'NONE', *, *, #7168, .T. ) ;
#12799=ORIENTED_EDGE ( 'NONE', *, *, #8761, .T. ) ;
#12802=DIRECTION ( 'NONE',  ( -0.08563346120589268584, -1.048707441657055866E-17, -0.9963267086261908823 ) ) ;
#12803=CARTESIAN_POINT ( 'NONE',  ( -25.73489962141544751, -4.139534227248430120, 60.85000000000000142 ) ) ;
#12804=VERTEX_POINT ( 'NONE', #4731 ) ;
#12805=CARTESIAN_POINT ( 'NONE',  ( -18.05918829504999934, 30.47290950744599769, 57.35000000000000142 ) ) ;
#12809=CARTESIAN_POINT ( 'NONE',  ( 3.190811704950004657, 27.97290950744599769, 64.35000000000000853 ) ) ;
#12811=EDGE_CURVE ( 'NONE', #6784, #999, #11021, .T. ) ;
#12812=CARTESIAN_POINT ( 'NONE',  ( -38.63164489498320364, 10.97290950744599947, 64.85000000000000853 ) ) ;
#12813=ORIENTED_EDGE ( 'NONE', *, *, #12580, .T. ) ;
#12814=EDGE_CURVE ( 'NONE', #3894, #12773, #8986, .T. ) ;
#12815=DIRECTION ( 'NONE',  ( 0.000000000000000000, 0.000000000000000000, 1.000000000000000000 ) ) ;
#12816=DIRECTION ( 'NONE',  ( 0.4528443260392608916, 0.8915896008669277339, 0.000000000000000000 ) ) ;
#12817=CARTESIAN_POINT ( 'NONE',  ( -12.26420230435512160, 9.417873376788568507, 67.84999999999999432 ) ) ;
#12818=CIRCLE ( 'NONE', #3036, 4.750000000000000000 ) ;
#12822=DIRECTION ( 'NONE',  ( -1.000000000000000000, 0.000000000000000000, 0.000000000000000000 ) ) ;
#12823=CARTESIAN_POINT ( 'NONE',  ( -1.059188295049996231, -6.027090492554000534, 5.250000000000000000 ) ) ;
#12825=DIRECTION ( 'NONE',  ( 0.000000000000000000, 0.000000000000000000, 1.000000000000000000 ) ) ;
#12827=DIRECTION ( 'NONE',  ( 0.9496839325805410681, -0.3132098788326420080, 0.000000000000000000 ) ) ;
#12829=CYLINDRICAL_SURFACE ( 'NONE', #2500, 8.250000000000001776 ) ;
#12830=ADVANCED_FACE ( 'NONE', ( #8777, #7918 ), #3621, .F. ) ;
#12833=AXIS2_PLACEMENT_3D ( 'NONE', #1508, #6885, #3483 ) ;
#12834=DIRECTION ( 'NONE',  ( 0.3202092937642119774, 0.6304490528084099044, 0.7071067811865499042 ) ) ;
#12835=CARTESIAN_POINT ( 'NONE',  ( -18.05918829504999934, 10.97290950744599947, 30.59999999999999787 ) ) ;
#12836=ORIENTED_EDGE ( 'NONE', *, *, #739, .F. ) ;
#12838=CARTESIAN_POINT ( 'NONE',  ( -15.27055863119252699, 30.19228463276535734, 54.37235416479132510 ) ) ;
#12840=DIRECTION ( 'NONE',  ( 0.000000000000000000, 0.000000000000000000, 1.000000000000000000 ) ) ;
#12841=DIRECTION ( 'NONE',  ( 0.9496839325805410681, 0.3132098788326420080, 0.000000000000000000 ) ) ;
#12842=DIRECTION ( 'NONE',  ( 0.2878798879079283446, -0.9576665234506834823, 0.000000000000000000 ) ) ;
#12844=ORIENTED_EDGE ( 'NONE', *, *, #2165, .F. ) ;
#12846=DIRECTION ( 'NONE',  ( 0.4528443260392608360, 0.8915896008669278450, 0.000000000000000000 ) ) ;
#12847=EDGE_CURVE ( 'NONE', #10843, #8732, #3994, .T. ) ;
#12848=CARTESIAN_POINT ( 'NONE',  ( -18.05918829504999934, 10.00028003023991907, 62.14999999999999858 ) ) ;
#12849=AXIS2_PLACEMENT_3D ( 'NONE', #4817, #422, #12221 ) ;
#12851=CARTESIAN_POINT ( 'NONE',  ( -18.05918829504999934, 7.130333642789880244, 68.85549045786049760 ) ) ;
#12852=EDGE_CURVE ( 'NONE', #9911, #6154, #8896, .T. ) ;
#12855=ORIENTED_EDGE ( 'NONE', *, *, #739, .T. ) ;
#12858=VERTEX_POINT ( 'NONE', #1372 ) ;
#12859=ORIENTED_EDGE ( 'NONE', *, *, #13194, .F. ) ;
#12869=DIRECTION ( 'NONE',  ( 0.000000000000000000, 0.000000000000000000, 1.000000000000000000 ) ) ;
#12870=DIRECTION ( 'NONE',  ( 0.000000000000000000, 0.000000000000000000, 1.000000000000000000 ) ) ;
#12871=DIRECTION ( 'NONE',  ( 0.000000000000000000, 0.000000000000000000, -1.000000000000000000 ) ) ;
#12873=CARTESIAN_POINT ( 'NONE',  ( -30.48673169511680214, 10.97290950744599947, 17.25000000000000000 ) ) ;
#12875=AXIS2_PLACEMENT_3D ( 'NONE', #4331, #2388, #9854 ) ;
#12877=DIRECTION ( 'NONE',  ( -0.6615960714621564875, 0.7498604124941129490, 0.000000000000000000 ) ) ;
#12878=CIRCLE ( 'NONE', #10216, 4.250000000000003553 ) ;
#12880=AXIS2_PLACEMENT_3D ( 'NONE', #13169, #2528, #10053 ) ;
#12884=CARTESIAN_POINT ( 'NONE',  ( -20.83881167003955781, 30.19337278744001196, 54.36146151962581285 ) ) ;
#12885=CARTESIAN_POINT ( 'NONE',  ( -18.05918829504999934, 10.97290950744599947, 60.75000000000000000 ) ) ;
#12886=FACE_OUTER_BOUND ( 'NONE', #11866, .T. ) ;
#12888=LINE ( 'NONE', #5625, #684 ) ;
#12889=DIRECTION ( 'NONE',  ( -1.000000000000000000, 0.000000000000000000, 0.000000000000000000 ) ) ;
#12890=EDGE_CURVE ( 'NONE', #3252, #12241, #5950, .T. ) ;
#12891=CIRCLE ( 'NONE', #9782, 34.70000000000000284 ) ;
#12892=CIRCLE ( 'NONE', #10007, 17.66282263685195275 ) ;
#12893=LINE ( 'NONE', #7492, #11718 ) ;
#12894=ORIENTED_EDGE ( 'NONE', *, *, #3008, .T. ) ;
#12895=ORIENTED_EDGE ( 'NONE', *, *, #12598, .T. ) ;
#12896=EDGE_LOOP ( 'NONE', ( #9882, #8709, #1581, #894, #3892, #6369 ) ) ;
#12897=VERTEX_POINT ( 'NONE', #594 ) ;
#12898=LINE ( 'NONE', #11870, #7730 ) ;
#12899=CARTESIAN_POINT ( 'NONE',  ( -18.05918829504999934, 10.97290950744599947, 62.14999999999999858 ) ) ;
#12902=VECTOR ( 'NONE', #6807, 1000.000000000000000 ) ;
#12904=DIRECTION ( 'NONE',  ( 1.000000000000000000, 0.000000000000000000, 0.000000000000000000 ) ) ;
#12907=FACE_OUTER_BOUND ( 'NONE', #2897, .T. ) ;
#12908=EDGE_CURVE ( 'NONE', #6318, #9883, #12267, .T. ) ;
#12910=VERTEX_POINT ( 'NONE', #13445 ) ;
#12912=VECTOR ( 'NONE', #10422, 1000.000000000000000 ) ;
#12913=CARTESIAN_POINT ( 'NONE',  ( -15.82870473472232753, 30.25294134154687598, 53.81423550378804066 ) ) ;
#12914=DIRECTION ( 'NONE',  ( -0.3132098788326420635, 0.9496839325805410681, 0.000000000000000000 ) ) ;
#12916=CARTESIAN_POINT ( 'NONE',  ( -15.54512322349380149, 8.123439939968370993, 27.09999999999999787 ) ) ;
#12917=ORIENTED_EDGE ( 'NONE', *, *, #2930, .T. ) ;
#12924=VERTEX_POINT ( 'NONE', #6097 ) ;
#12926=ADVANCED_FACE ( 'NONE', ( #9117 ), #795, .F. ) ;
#12927=ORIENTED_EDGE ( 'NONE', *, *, #13319, .T. ) ;
#12928=VERTEX_POINT ( 'NONE', #2925 ) ;
#12930=ORIENTED_EDGE ( 'NONE', *, *, #5640, .T. ) ;
#12931=EDGE_LOOP ( 'NONE', ( #11892, #13733, #11623, #59 ) ) ;
#12932=ORIENTED_EDGE ( 'NONE', *, *, #11594, .T. ) ;
#12933=B_SPLINE_CURVE_WITH_KNOTS ( 'NONE', 3,
 ( #6051, #11436, #11368, #9056, #9273, #1875, #10384, #1725, #13315, #8011, #12285, #2736, #2867 ),
 .UNSPECIFIED., .F., .F.,
 ( 4, 1, 1, 1, 1, 1, 2, 2, 4 ),
 ( 0.000000000000000000, 0.2499999999999435452, 0.3749999999999139022, 0.4374999999999008016, 0.4687499999998942513, 0.4843749999998905875, 0.4921874999998887001, 0.4999999999998868128, 1.000000000000000000 ),
 .UNSPECIFIED. ) ;
#12935=PRODUCT ( 'compact pneumatic cylinder', 'compact pneumatic cylinder', '', ( #1143 ) ) ;
#12937=DIRECTION ( 'NONE',  ( 0.000000000000000000, 0.000000000000000000, -1.000000000000000000 ) ) ;
#12938=CARTESIAN_POINT ( 'NONE',  ( -18.05918829504999934, 30.47290950744599769, 52.80340000000000344 ) ) ;
#12944=DIRECTION ( 'NONE',  ( 0.4528443260392610026, 0.8915896008669277339, 0.000000000000000000 ) ) ;
#12949=CIRCLE ( 'NONE', #6026, 2.700000000000001066 ) ;
#12950=ADVANCED_FACE ( 'NONE', ( #13577, #1924 ), #13371, .F. ) ;
#12951=EDGE_LOOP ( 'NONE', ( #8470, #8635, #10851, #3734 ) ) ;
#12952=CARTESIAN_POINT ( 'NONE',  ( -23.42001676333060090, -4.028726038184999858, 62.14999999999999858 ) ) ;
#12954=ORIENTED_EDGE ( 'NONE', *, *, #3018, .F. ) ;
#12955=DIRECTION ( 'NONE',  ( -0.000000000000000000, -0.000000000000000000, -1.000000000000000000 ) ) ;
#12957=EDGE_CURVE ( 'NONE', #13546, #12858, #6186, .T. ) ;
#12958=CARTESIAN_POINT ( 'NONE',  ( -18.62368403728828170, 30.35356550733773418, 53.03788860485584422 ) ) ;
#12959=VECTOR ( 'NONE', #12242, 1000.000000000000000 ) ;
#12960=CIRCLE ( 'NONE', #6935, 6.449999999999997513 ) ;
#12961=CARTESIAN_POINT ( 'NONE',  ( -3.743645030049981948, 18.13068114044599710, 61.70038048200006386 ) ) ;
#12962=VECTOR ( 'NONE', #6267, 1000.000000000000000 ) ;
#12963=DIRECTION ( 'NONE',  ( -1.000000000000000000, 0.000000000000000000, 0.000000000000000000 ) ) ;
#12964=CARTESIAN_POINT ( 'NONE',  ( -18.05918829504999934, 10.97290950744599947, 63.45000000000000284 ) ) ;
#12965=CARTESIAN_POINT ( 'NONE',  ( -18.05918829504999934, 10.97290950744599947, 63.54999999999999716 ) ) ;
#12966=EDGE_CURVE ( 'NONE', #7434, #4562, #12544, .T. ) ;
#12969=CIRCLE ( 'NONE', #10088, 3.500000000000000888 ) ;
#12970=EDGE_LOOP ( 'NONE', ( #10108, #9863 ) ) ;
#12973=ORIENTED_EDGE ( 'NONE', *, *, #5061, .F. ) ;
#12976=DIRECTION ( 'NONE',  ( 1.000000000000000000, 0.000000000000000000, 0.000000000000000000 ) ) ;
#12979=DIRECTION ( 'NONE',  ( 0.000000000000000000, 0.000000000000000000, -1.000000000000000000 ) ) ;
#12980=DIRECTION ( 'NONE',  ( 0.000000000000000000, 0.000000000000000000, 1.000000000000000000 ) ) ;
#12981=CARTESIAN_POINT ( 'NONE',  ( 3.690811704950009986, 27.97290950744599769, 64.85000000000000853 ) ) ;
#12982=CARTESIAN_POINT ( 'NONE',  ( -24.47918829505000105, 10.97290950744599947, 64.85000000000000853 ) ) ;
#12985=DIRECTION ( 'NONE',  ( -1.000000000000000000, 0.000000000000000000, 0.000000000000000000 ) ) ;
#12989=CARTESIAN_POINT ( 'NONE',  ( -16.63855339399303901, 30.31714196968558284, 53.30236028803027892 ) ) ;
#12992=CARTESIAN_POINT ( 'NONE',  ( -11.70083760351054103, 35.47811937223634970, 5.250000000000000000 ) ) ;
#12994=VECTOR ( 'NONE', #8117, 1000.000000000000000 ) ;
#12995=ORIENTED_EDGE ( 'NONE', *, *, #10827, .F. ) ;
#12997=CYLINDRICAL_SURFACE ( 'NONE', #1793, 6.450000000000001066 ) ;
#12998=EDGE_CURVE ( 'NONE', #6577, #9897, #11484, .T. ) ;
#13003=VERTEX_POINT ( 'NONE', #868 ) ;
#13008=EDGE_LOOP ( 'NONE', ( #9583, #12099, #2182, #11559 ) ) ;
#13010=CARTESIAN_POINT ( 'NONE',  ( -15.54654308236029792, 19.85770471824265115, 64.85000000000000853 ) ) ;
#13011=EDGE_LOOP ( 'NONE', ( #4561, #3021, #5153, #6981 ) ) ;
#13015=FACE_OUTER_BOUND ( 'NONE', #8967, .T. ) ;
#13016=CARTESIAN_POINT ( 'NONE',  ( -1.059188295049996231, 10.97290950744599947, 57.35000000000000142 ) ) ;
#13017=EDGE_CURVE ( 'NONE', #7262, #8225, #12439, .T. ) ;
#13018=CARTESIAN_POINT ( 'NONE',  ( -35.05918829505000645, -6.027090492554000534, 64.35000000000000853 ) ) ;
#13020=ORIENTED_EDGE ( 'NONE', *, *, #9951, .T. ) ;
#13021=ORIENTED_EDGE ( 'NONE', *, *, #4412, .F. ) ;
#13022=ORIENTED_EDGE ( 'NONE', *, *, #8850, .F. ) ;
#13025=CYLINDRICAL_SURFACE ( 'NONE', #12295, 4.000000000000000888 ) ;
#13027=CARTESIAN_POINT ( 'NONE',  ( -20.04570110035189856, 30.27520963117099839, 53.62886082399810306 ) ) ;
#13030=CARTESIAN_POINT ( 'NONE',  ( -27.15409092487699994, 0.3335619008453594714, 62.14999999999999858 ) ) ;
#13031=DIRECTION ( 'NONE',  ( 0.000000000000000000, 0.000000000000000000, -1.000000000000000000 ) ) ;
#13032=ADVANCED_FACE ( 'NONE', ( #9258 ), #7071, .F. ) ;
#13035=ORIENTED_EDGE ( 'NONE', *, *, #10237, .F. ) ;
#13038=ORIENTED_EDGE ( 'NONE', *, *, #10248, .T. ) ;
#13039=ORIENTED_EDGE ( 'NONE', *, *, #3001, .F. ) ;
#13042=ORIENTED_EDGE ( 'NONE', *, *, #13552, .T. ) ;
#13044=CARTESIAN_POINT ( 'NONE',  ( -12.47577096721731849, 9.231207973652310272, 68.00596099852270982 ) ) ;
#13048=LINE ( 'NONE', #11162, #13341 ) ;
#13049=CYLINDRICAL_SURFACE ( 'NONE', #6265, 17.66282263685195275 ) ;
#13053=CIRCLE ( 'NONE', #7440, 33.00000000000000000 ) ;
#13057=EDGE_LOOP ( 'NONE', ( #5602, #1058, #7263, #8062 ) ) ;
#13058=FACE_OUTER_BOUND ( 'NONE', #1855, .T. ) ;
#13060=CYLINDRICAL_SURFACE ( 'NONE', #587, 17.66282263685195275 ) ;
#13061=AXIS2_PLACEMENT_3D ( 'NONE', #11173, #6704, #2749 ) ;
#13062=CYLINDRICAL_SURFACE ( 'NONE', #673, 17.00000000000000000 ) ;
#13065=DIRECTION ( 'NONE',  ( -1.821689671877679746E-15, -1.000000000000000000, 2.732534507816519619E-15 ) ) ;
#13071=EDGE_LOOP ( 'NONE', ( #351, #11346, #12320, #12166 ) ) ;
#13072=CARTESIAN_POINT ( 'NONE',  ( 3.190811704950004657, 27.97290950744599769, 58.85000000000000142 ) ) ;
#13073=EDGE_LOOP ( 'NONE', ( #3281, #857, #7280, #4343 ) ) ;
#13078=CARTESIAN_POINT ( 'NONE',  ( -20.57325336660620252, 13.82237907492362083, 27.09999999999999787 ) ) ;
#13079=VERTEX_POINT ( 'NONE', #10718 ) ;
#13080=CARTESIAN_POINT ( 'NONE',  ( -18.05918829504999934, 10.97290950744599947, 60.40999999999999659 ) ) ;
#13082=LINE ( 'NONE', #3525, #12040 ) ;
#13084=ORIENTED_EDGE ( 'NONE', *, *, #5943, .T. ) ;
#13092=ORIENTED_EDGE ( 'NONE', *, *, #11954, .F. ) ;
#13094=CARTESIAN_POINT ( 'NONE',  ( -20.95080569073241605, 30.17981166141560578, 54.49760474301193369 ) ) ;
#13098=CARTESIAN_POINT ( 'NONE',  ( -18.05918829504999934, 10.97290950744599947, 58.54999999999999716 ) ) ;
#13100=DIRECTION ( 'NONE',  ( -1.000000000000000000, 0.000000000000000000, 0.000000000000000000 ) ) ;
#13101=CIRCLE ( 'NONE', #5992, 4.749999999999997335 ) ;
#13105=CYLINDRICAL_SURFACE ( 'NONE', #8705, 16.72262947720610171 ) ;
#13106=EDGE_LOOP ( 'NONE', ( #3048, #4642, #10776, #4147 ) ) ;
#13107=ORIENTED_EDGE ( 'NONE', *, *, #7727, .F. ) ;
#13108=LINE ( 'NONE', #7789, #12505 ) ;
#13114=DIRECTION ( 'NONE',  ( 0.000000000000000000, 0.000000000000000000, 1.000000000000000000 ) ) ;
#13116=DIRECTION ( 'NONE',  ( 0.000000000000000000, 0.000000000000000000, -1.000000000000000000 ) ) ;
#13120=VECTOR ( 'NONE', #1825, 1000.000000000000114 ) ;
#13122=ORIENTED_EDGE ( 'NONE', *, *, #9080, .T. ) ;
#13128=AXIS2_PLACEMENT_3D ( 'NONE', #5272, #10535, #12963 ) ;
#13130=DIRECTION ( 'NONE',  ( -1.000000000000000000, 0.000000000000000000, 0.000000000000000000 ) ) ;
#13132=CARTESIAN_POINT ( 'NONE',  ( -18.05918829504999934, 10.97290950744599947, 30.59999999999999787 ) ) ;
#13133=DIRECTION ( 'NONE',  ( 0.4678190685372728419, -0.5302313826179317902, 0.7071067811865437980 ) ) ;
#13137=DIRECTION ( 'NONE',  ( -0.1353548076753729457, -1.657618319688509444E-17, -0.9907971921837297469 ) ) ;
#13140=EDGE_CURVE ( 'NONE', #9237, #8057, #6629, .T. ) ;
#13141=CYLINDRICAL_SURFACE ( 'NONE', #2370, 4.250000000000000000 ) ;
#13142=ORIENTED_EDGE ( 'NONE', *, *, #7508, .T. ) ;
#13143=ORIENTED_EDGE ( 'NONE', *, *, #1753, .F. ) ;
#13144=EDGE_LOOP ( 'NONE', ( #11201, #6636, #1197, #12813, #2350 ) ) ;
#13147=CARTESIAN_POINT ( 'NONE',  ( -1.059188295049996231, -6.027090492554000534, 64.85000000000000853 ) ) ;
#13149=ORIENTED_EDGE ( 'NONE', *, *, #11475, .T. ) ;
#13152=VECTOR ( 'NONE', #9095, 1000.000000000000000 ) ;
#13154=AXIS2_PLACEMENT_3D ( 'NONE', #10042, #461, #7783 ) ;
#13163=CARTESIAN_POINT ( 'NONE',  ( -25.22489219260310023, -4.443078545630350540, 62.14999999999999858 ) ) ;
#13164=ORIENTED_EDGE ( 'NONE', *, *, #11225, .T. ) ;
#13166=CARTESIAN_POINT ( 'NONE',  ( -18.05918829504999934, 10.97290950744599947, 116.8499999999999943 ) ) ;
#13167=CARTESIAN_POINT ( 'NONE',  ( -21.30030954502889173, 30.13305483534595197, 59.66158781348052997 ) ) ;
#13169=CARTESIAN_POINT ( 'NONE',  ( -18.05918829504999934, 10.97290950744599947, 60.04999999999999716 ) ) ;
#13175=AXIS2_PLACEMENT_3D ( 'NONE', #9181, #3877, #13433 ) ;
#13176=CIRCLE ( 'NONE', #12287, 6.145833333000000565 ) ;
#13177=EDGE_CURVE ( 'NONE', #12897, #7297, #12878, .T. ) ;
#13178=ORIENTED_EDGE ( 'NONE', *, *, #12847, .T. ) ;
#13181=PLANE ( 'NONE',  #8466 ) ;
#13182=AXIS2_PLACEMENT_3D ( 'NONE', #1499, #5754, #12131 ) ;
#13183=EDGE_LOOP ( 'NONE', ( #3522, #7184, #1030, #3555 ) ) ;
#13188=DIRECTION ( 'NONE',  ( 1.000000000000000000, 0.000000000000000000, 0.000000000000000000 ) ) ;
#13189=DIRECTION ( 'NONE',  ( 0.000000000000000000, 0.000000000000000000, 1.000000000000000000 ) ) ;
#13190=DIRECTION ( 'NONE',  ( -1.000000000000000000, 0.000000000000000000, 0.000000000000000000 ) ) ;
#13192=DIRECTION ( 'NONE',  ( 0.000000000000000000, 0.000000000000000000, -1.000000000000000000 ) ) ;
#13193=LINE ( 'NONE', #8861, #10902 ) ;
#13194=EDGE_CURVE ( 'NONE', #11014, #7637, #835, .T. ) ;
#13195=SHAPE_REPRESENTATION ( 'compact pneumatic cylinder', ( #6434 ), #5097 ) ;
#13196=CIRCLE ( 'NONE', #4283, 34.70000000000000284 ) ;
#13197=ORIENTED_EDGE ( 'NONE', *, *, #7104, .F. ) ;
#13198=ORIENTED_EDGE ( 'NONE', *, *, #12315, .F. ) ;
#13200=ORIENTED_EDGE ( 'NONE', *, *, #11241, .T. ) ;
#13202=ORIENTED_EDGE ( 'NONE', *, *, #3433, .T. ) ;
#13208=ADVANCED_FACE ( 'NONE', ( #5325 ), #8345, .F. ) ;
#13210=EDGE_CURVE ( 'NONE', #6644, #8435, #9756, .T. ) ;
#13212=VERTEX_POINT ( 'NONE', #7340 ) ;
#13213=ORIENTED_EDGE ( 'NONE', *, *, #6328, .T. ) ;
#13217=DIRECTION ( 'NONE',  ( 1.000000000000000000, 0.000000000000000000, 0.000000000000000000 ) ) ;
#13219=VERTEX_POINT ( 'NONE', #12373 ) ;
#13220=ORIENTED_EDGE ( 'NONE', *, *, #7980, .F. ) ;
#13223=FACE_OUTER_BOUND ( 'NONE', #3574, .T. ) ;
#13225=EDGE_LOOP ( 'NONE', ( #1699, #2782, #1379, #2593 ) ) ;
#13227=DIRECTION ( 'NONE',  ( 0.000000000000000000, 0.000000000000000000, -1.000000000000000000 ) ) ;
#13228=CARTESIAN_POINT ( 'NONE',  ( -18.05918829504999934, 10.97290950744599947, 60.85000000000000142 ) ) ;
#13230=DIRECTION ( 'NONE',  ( 0.000000000000000000, 0.000000000000000000, 1.000000000000000000 ) ) ;
#13233=CIRCLE ( 'NONE', #1406, 16.00000000000000000 ) ;
#13235=EDGE_LOOP ( 'NONE', ( #4121, #3932, #5743, #8602 ) ) ;
#13237=VERTEX_POINT ( 'NONE', #501 ) ;
#13239=CARTESIAN_POINT ( 'NONE',  ( -21.89015644058605758, 30.04220389462367891, 56.84109027995026509 ) ) ;
#13242=LINE ( 'NONE', #3682, #3620 ) ;
#13243=CONICAL_SURFACE ( 'NONE', #6000, 16.95000000000000284, 0.7853981633974447263 ) ;
#13244=DIRECTION ( 'NONE',  ( 0.000000000000000000, 0.000000000000000000, 1.000000000000000000 ) ) ;
#13245=EDGE_CURVE ( 'NONE', #898, #10213, #9996, .T. ) ;
#13246=DIRECTION ( 'NONE',  ( -0.9496839325805410681, 0.3132098788326420080, 0.000000000000000000 ) ) ;
#13248=CARTESIAN_POINT ( 'NONE',  ( -18.05918829504999934, 10.97290950744599947, 61.86500000000000199 ) ) ;
#13249=CYLINDRICAL_SURFACE ( 'NONE', #5069, 2.500000000000000000 ) ;
#13250=CARTESIAN_POINT ( 'NONE',  ( -18.05918829504999934, 10.97290950744599947, 63.02000000000000313 ) ) ;
#13253=CARTESIAN_POINT ( 'NONE',  ( -35.05918829505000645, -6.027090492554000534, 64.85000000000000853 ) ) ;
#13255=DIRECTION ( 'NONE',  ( 0.000000000000000000, 0.000000000000000000, -1.000000000000000000 ) ) ;
#13257=CARTESIAN_POINT ( 'NONE',  ( -36.05918829505000645, 10.97290950744599947, 62.14999999999999858 ) ) ;
#13258=ORIENTED_EDGE ( 'NONE', *, *, #7920, .T. ) ;
#13261=EDGE_CURVE ( 'NONE', #3141, #1834, #3536, .T. ) ;
#13262=VERTEX_POINT ( 'NONE', #7620 ) ;
#13263=DIRECTION ( 'NONE',  ( 0.000000000000000000, 0.000000000000000000, -1.000000000000000000 ) ) ;
#13265=DIRECTION ( 'NONE',  ( 0.000000000000000000, 0.000000000000000000, 1.000000000000000000 ) ) ;
#13267=ADVANCED_FACE ( 'NONE', ( #13335 ), #12750, .T. ) ;
#13268=DIRECTION ( 'NONE',  ( 0.4528443260392608916, 0.8915896008669279560, 0.000000000000000000 ) ) ;
#13269=( BOUNDED_SURFACE ( )  B_SPLINE_SURFACE ( 3, 3, ( 
 ( #8045, #640, #2561, #9941 ),
 ( #13426, #368, #575, #9174 ),
 ( #11128, #5806, #11202, #3599 ),
 ( #12325, #4776, #3870, #7968 ) ),
 .UNSPECIFIED., .F., .F., .T. ) 
 B_SPLINE_SURFACE_WITH_KNOTS ( ( 4, 4 ),
 ( 4, 4 ),
 ( 0.000000000000000000, 1.000000000000000000 ),
 ( 0.000000000000000000, 1.000000000000000000 ),
 .UNSPECIFIED. ) 
 GEOMETRIC_REPRESENTATION_ITEM ( )  RATIONAL_B_SPLINE_SURFACE ( (
 ( 1.000000000000000000, 0.3333333333333329818, 0.3333333333333329818, 1.000000000000000000),
 ( 0.4470472315060959878, 0.1490157438353659769, 0.1490157438353659769, 0.4470472315060959878),
 ( 0.4470472315060959878, 0.1490157438353659769, 0.1490157438353659769, 0.4470472315060959878),
 ( 1.000000000000000000, 0.3333333333333329818, 0.3333333333333329818, 1.000000000000000000) ) ) 
 REPRESENTATION_ITEM ( '' )  SURFACE ( )  );
#13271=DIRECTION ( 'NONE',  ( -1.000000000000000000, 0.000000000000000000, 0.000000000000000000 ) ) ;
#13272=CARTESIAN_POINT ( 'NONE',  ( -1.396365658198039927, 10.97290950744599947, 6.250000000000000000 ) ) ;
#13273=ORIENTED_EDGE ( 'NONE', *, *, #9951, .F. ) ;
#13274=AXIS2_PLACEMENT_3D ( 'NONE', #10200, #7808, #617 ) ;
#13276=CARTESIAN_POINT ( 'NONE',  ( -16.30032143609284034, 30.29381900179400589, 61.21967481679787682 ) ) ;
#13277=EDGE_CURVE ( 'NONE', #8708, #349, #153, .T. ) ;
#13278=ORIENTED_EDGE ( 'NONE', *, *, #2343, .F. ) ;
#13279=ORIENTED_EDGE ( 'NONE', *, *, #8938, .F. ) ;
#13280=EDGE_LOOP ( 'NONE', ( #4811, #1956, #117, #4610 ) ) ;
#13282=ORIENTED_EDGE ( 'NONE', *, *, #8256, .T. ) ;
#13283=ADVANCED_FACE ( 'NONE', ( #8107 ), #13413, .T. ) ;
#13284=CYLINDRICAL_SURFACE ( 'NONE', #8226, 2.700000000000000178 ) ;
#13285=DIRECTION ( 'NONE',  ( 0.000000000000000000, 0.000000000000000000, 1.000000000000000000 ) ) ;
#13286=VERTEX_POINT ( 'NONE', #4760 ) ;
#13287=EDGE_CURVE ( 'NONE', #4217, #6494, #1065, .T. ) ;
#13290=CARTESIAN_POINT ( 'NONE',  ( -19.55918829504999934, 27.19822998463872565, 57.14449823292531505 ) ) ;
#13291=ADVANCED_FACE ( 'NONE', ( #9815, #12229, #13015 ), #6653, .T. ) ;
#13293=DIRECTION ( 'NONE',  ( 0.000000000000000000, 0.000000000000000000, -1.000000000000000000 ) ) ;
#13295=EDGE_LOOP ( 'NONE', ( #7405, #7457, #12478, #13737, #6174 ) ) ;
#13297=CIRCLE ( 'NONE', #1032, 16.75000000000000355 ) ;
#13300=EDGE_CURVE ( 'NONE', #10154, #6107, #12454, .T. ) ;
#13301=CARTESIAN_POINT ( 'NONE',  ( -20.84843554743573435, 30.19221003206969201, 54.37310230029029157 ) ) ;
#13302=CARTESIAN_POINT ( 'NONE',  ( -20.04397650943645459, 13.22249074492834175, 24.10000000000000142 ) ) ;
#13306=EDGE_CURVE ( 'NONE', #2826, #8318, #7986, .T. ) ;
#13307=CARTESIAN_POINT ( 'NONE',  ( -30.80918829504999934, 27.97290950744599769, 58.85000000000000142 ) ) ;
#13309=CARTESIAN_POINT ( 'NONE',  ( -18.05918829504999934, 10.97290950744599947, 68.84999999999999432 ) ) ;
#13310=LINE ( 'NONE', #12276, #5122 ) ;
#13311=CARTESIAN_POINT ( 'NONE',  ( -23.57208814848684852, -7.366404416634599883, 62.14999999999999858 ) ) ;
#13312=FILL_AREA_STYLE ('',( #3632 ) ) ;
#13313=AXIS2_PLACEMENT_3D ( 'NONE', #9418, #8082, #3834 ) ;
#13314=CYLINDRICAL_SURFACE ( 'NONE', #10966, 5.000000000000000888 ) ;
#13315=CARTESIAN_POINT ( 'NONE',  ( -22.67016924028392921, 13.57258417831237729, 68.55666012861996705 ) ) ;
#13317=DIRECTION ( 'NONE',  ( 0.000000000000000000, 0.000000000000000000, 1.000000000000000000 ) ) ;
#13319=EDGE_CURVE ( 'NONE', #9911, #2900, #8312, .T. ) ;
#13320=DIRECTION ( 'NONE',  ( -1.000000000000000000, 0.000000000000000000, 0.000000000000000000 ) ) ;
#13324=EDGE_LOOP ( 'NONE', ( #10528, #5109, #3491, #3024 ) ) ;
#13325=EDGE_LOOP ( 'NONE', ( #2810, #7011, #6533 ) ) ;
#13328=ORIENTED_EDGE ( 'NONE', *, *, #9899, .F. ) ;
#13335=FACE_OUTER_BOUND ( 'NONE', #233, .T. ) ;
#13336=DIRECTION ( 'NONE',  ( -1.000000000000000000, 0.000000000000000000, 0.000000000000000000 ) ) ;
#13338=EDGE_CURVE ( 'NONE', #11332, #6506, #2668, .T. ) ;
#13339=AXIS2_PLACEMENT_3D ( 'NONE', #7095, #5976, #6117 ) ;
#13340=CIRCLE ( 'NONE', #10462, 16.00000000000000000 ) ;
#13341=VECTOR ( 'NONE', #3694, 1000.000000000000114 ) ;
#13342=CIRCLE ( 'NONE', #1758, 4.749999999999997335 ) ;
#13343=VERTEX_POINT ( 'NONE', #768 ) ;
#13344=LINE ( 'NONE', #2554, #4579 ) ;
#13346=ORIENTED_EDGE ( 'NONE', *, *, #9760, .T. ) ;
#13347=ORIENTED_EDGE ( 'NONE', *, *, #2914, .T. ) ;
#13348=DIRECTION ( 'NONE',  ( 1.000000000000000000, 3.574581708073420512E-15, 0.000000000000000000 ) ) ;
#13349=DIRECTION ( 'NONE',  ( 0.000000000000000000, 0.000000000000000000, -1.000000000000000000 ) ) ;
#13351=ORIENTED_EDGE ( 'NONE', *, *, #12167, .T. ) ;
#13352=CARTESIAN_POINT ( 'NONE',  ( -25.73489962141544751, -4.139534227248430120, 58.35000000000000142 ) ) ;
#13354=CARTESIAN_POINT ( 'NONE',  ( -8.964285665223000521, 0.3335619008453594714, 63.45000000000000284 ) ) ;
#13355=AXIS2_PLACEMENT_3D ( 'NONE', #5092, #1964, #979 ) ;
#13359=ADVANCED_FACE ( 'NONE', ( #13744 ), #5094, .T. ) ;
#13364=VECTOR ( 'NONE', #7197, 1000.000000000000000 ) ;
#13366=EDGE_CURVE ( 'NONE', #8674, #5058, #4069, .T. ) ;
#13367=TOROIDAL_SURFACE ( 'NONE', #3132, 16.66282263685194920, 1.000000000000000000 ) ;
#13368=DIRECTION ( 'NONE',  ( 0.000000000000000000, -1.000000000000000000, 1.672022627447524796E-15 ) ) ;
#13369=CARTESIAN_POINT ( 'NONE',  ( -21.88875334366193570, 30.04243591130237689, 57.61769108546867102 ) ) ;
#13371=PLANE ( 'NONE',  #7977 ) ;
#13372=CARTESIAN_POINT ( 'NONE',  ( 2.262399129208275017, -0.4981161769137599782, 17.25000000000000000 ) ) ;
#13373=DIRECTION ( 'NONE',  ( 0.000000000000000000, 0.000000000000000000, -1.000000000000000000 ) ) ;
#13375=VERTEX_POINT ( 'NONE', #9498 ) ;
#13377=AXIS2_PLACEMENT_3D ( 'NONE', #7112, #1678, #7043 ) ;
#13378=CIRCLE ( 'NONE', #4915, 18.00000000000000000 ) ;
#13379=EDGE_CURVE ( 'NONE', #10213, #7294, #8207, .T. ) ;
#13380=CARTESIAN_POINT ( 'NONE',  ( -18.05918829504999934, 10.97290950744599947, 64.85000000000000853 ) ) ;
#13381=DIRECTION ( 'NONE',  ( -1.000000000000000000, 0.000000000000000000, 0.000000000000000000 ) ) ;
#13382=ORIENTED_EDGE ( 'NONE', *, *, #2498, .F. ) ;
#13383=DIRECTION ( 'NONE',  ( 0.000000000000000000, 0.000000000000000000, -1.000000000000000000 ) ) ;
#13384=CARTESIAN_POINT ( 'NONE',  ( -12.00918829505000041, 10.97290950744599947, 64.85000000000000853 ) ) ;
#13385=DIRECTION ( 'NONE',  ( 0.000000000000000000, 0.000000000000000000, -1.000000000000000000 ) ) ;
#13386=CARTESIAN_POINT ( 'NONE',  ( -18.05918829504999934, 10.97290950744599947, 7.250000000000000000 ) ) ;
#13389=DIRECTION ( 'NONE',  ( 1.000000000000000000, 0.000000000000000000, 0.000000000000000000 ) ) ;
#13390=CONICAL_SURFACE ( 'NONE', #7347, 16.00000000000000000, 0.7853981633974476129 ) ;
#13392=FACE_OUTER_BOUND ( 'NONE', #9895, .T. ) ;
#13398=AXIS2_PLACEMENT_3D ( 'NONE', #12071, #9055, #2592 ) ;
#13399=AXIS2_PLACEMENT_3D ( 'NONE', #5214, #9548, #13523 ) ;
#13400=ORIENTED_EDGE ( 'NONE', *, *, #2910, .F. ) ;
#13401=EDGE_CURVE ( 'NONE', #8804, #2573, #12007, .T. ) ;
#13402=EDGE_LOOP ( 'NONE', ( #10223, #10047 ) ) ;
#13405=ORIENTED_EDGE ( 'NONE', *, *, #12125, .T. ) ;
#13406=EDGE_LOOP ( 'NONE', ( #13143, #6902 ) ) ;
#13407=FACE_OUTER_BOUND ( 'NONE', #11687, .T. ) ;
#13408=LINE ( 'NONE', #3854, #10495 ) ;
#13412=VECTOR ( 'NONE', #6319, 1000.000000000000000 ) ;
#13413=CYLINDRICAL_SURFACE ( 'NONE', #411, 34.69999999999999574 ) ;
#13416=CARTESIAN_POINT ( 'NONE',  ( -18.05918829504999934, 10.97290950744599947, 57.35000000000000142 ) ) ;
#13417=ORIENTED_EDGE ( 'NONE', *, *, #13454, .T. ) ;
#13418=ORIENTED_EDGE ( 'NONE', *, *, #6998, .T. ) ;
#13419=CARTESIAN_POINT ( 'NONE',  ( -15.94002774258076016, 30.26343021274545109, 60.97416097055285178 ) ) ;
#13420=AXIS2_PLACEMENT_3D ( 'NONE', #8970, #3668, #5666 ) ;
#13421=ORIENTED_EDGE ( 'NONE', *, *, #1485, .T. ) ;
#13422=VERTEX_POINT ( 'NONE', #5996 ) ;
#13423=SURFACE_SIDE_STYLE ('',( #1763 ) ) ;
#13426=CARTESIAN_POINT ( 'NONE',  ( -18.05918829505001355, 18.23680593644599668, 62.03182374100007479 ) ) ;
#13427=EDGE_CURVE ( 'NONE', #8398, #1604, #1284, .T. ) ;
#13429=VERTEX_POINT ( 'NONE', #5168 ) ;
#13430=CARTESIAN_POINT ( 'NONE',  ( -1.059188295049996231, 27.97290950744599769, 7.250000000000000000 ) ) ;
#13432=DIRECTION ( 'NONE',  ( 0.000000000000000000, 0.000000000000000000, 1.000000000000000000 ) ) ;
#13433=DIRECTION ( 'NONE',  ( -1.000000000000000000, 0.000000000000000000, 0.000000000000000000 ) ) ;
#13434=AXIS2_PLACEMENT_3D ( 'NONE', #2156, #5471, #7778 ) ;
#13436=CIRCLE ( 'NONE', #3861, 12.00000000000000355 ) ;
#13440=ADVANCED_FACE ( 'NONE', ( #2963 ), #7180, .T. ) ;
#13442=DIRECTION ( 'NONE',  ( 0.000000000000000000, 0.000000000000000000, -1.000000000000000000 ) ) ;
#13445=CARTESIAN_POINT ( 'NONE',  ( -15.34212233881444831, 16.32244711264754855, 57.35000000000000142 ) ) ;
#13447=CARTESIAN_POINT ( 'NONE',  ( -16.55918829504999579, 27.40458623260099813, 57.35000000000000142 ) ) ;
#13448=AXIS2_PLACEMENT_3D ( 'NONE', #579, #711, #1630 ) ;
#13450=CARTESIAN_POINT ( 'NONE',  ( -18.05918829504999934, 10.97290950744599947, 64.54999999999999716 ) ) ;
#13451=PLANE ( 'NONE',  #1951 ) ;
#13452=EDGE_LOOP ( 'NONE', ( #5031, #7982, #2824, #1457 ) ) ;
#13453=DIRECTION ( 'NONE',  ( 0.000000000000000000, 0.000000000000000000, -1.000000000000000000 ) ) ;
#13454=EDGE_CURVE ( 'NONE', #1735, #11332, #4470, .T. ) ;
#13455=CARTESIAN_POINT ( 'NONE',  ( -18.05918829504999934, 10.97290950744599947, 68.84999999999999432 ) ) ;
#13456=CARTESIAN_POINT ( 'NONE',  ( -18.05918829504999934, 10.97290950744599947, 61.65000000000000568 ) ) ;
#13457=CIRCLE ( 'NONE', #10344, 16.72262947720610171 ) ;
#13458=DIRECTION ( 'NONE',  ( 0.000000000000000000, 0.000000000000000000, -1.000000000000000000 ) ) ;
#13459=LINE ( 'NONE', #3903, #3853 ) ;
#13461=EDGE_CURVE ( 'NONE', #5721, #11514, #6489, .T. ) ;
#13462=CARTESIAN_POINT ( 'NONE',  ( -0.3963656581980404825, 10.97290950744599947, 5.250000000000000000 ) ) ;
#13463=DIRECTION ( 'NONE',  ( 0.000000000000000000, 0.000000000000000000, -1.000000000000000000 ) ) ;
#13464=ADVANCED_FACE ( 'NONE', ( #12907 ), #8726, .F. ) ;
#13467=ADVANCED_FACE ( 'NONE', ( #10759 ), #12672, .F. ) ;
#13470=ORIENTED_EDGE ( 'NONE', *, *, #4163, .F. ) ;
#13471=ORIENTED_EDGE ( 'NONE', *, *, #13565, .F. ) ;
#13472=CYLINDRICAL_SURFACE ( 'NONE', #13499, 1.500000000000001332 ) ;
#13474=EDGE_LOOP ( 'NONE', ( #10410, #12084, #8892, #13704, #7842, #7371, #11961, #3170 ) ) ;
#13476=DIRECTION ( 'NONE',  ( -1.000000000000000000, 0.000000000000000000, 0.000000000000000000 ) ) ;
#13478=CARTESIAN_POINT ( 'NONE',  ( -22.71804201037815218, -4.525318844826149878, 62.14999999999999858 ) ) ;
#13479=CARTESIAN_POINT ( 'NONE',  ( -11.46335496205000126, 10.97290950744599947, 60.40999999999999659 ) ) ;
#13480=CARTESIAN_POINT ( 'NONE',  ( -35.05918829505000645, -6.027090492554000534, 17.25000000000000000 ) ) ;
#13481=DIRECTION ( 'NONE',  ( 0.000000000000000000, 0.000000000000000000, 1.000000000000000000 ) ) ;
#13483=DIRECTION ( 'NONE',  ( 0.000000000000000000, 0.000000000000000000, -1.000000000000000000 ) ) ;
#13486=CARTESIAN_POINT ( 'NONE',  ( -15.35487948403739544, 30.20233709177388803, 60.42691889655178272 ) ) ;
#13488=CONICAL_SURFACE ( 'NONE', #3919, 3.800000000000001155, 0.7853981633974476129 ) ;
#13490=DIRECTION ( 'NONE',  ( -1.000000000000000000, 0.000000000000000000, 0.000000000000000000 ) ) ;
#13494=ORIENTED_EDGE ( 'NONE', *, *, #5834, .F. ) ;
#13495=CARTESIAN_POINT ( 'NONE',  ( -24.37001676333060018, -4.028726038184999858, 63.45000000000000284 ) ) ;
#13496=DIRECTION ( 'NONE',  ( 0.000000000000000000, 0.000000000000000000, -1.000000000000000000 ) ) ;
#13497=EDGE_CURVE ( 'NONE', #1261, #1264, #11877, .T. ) ;
#13498=CARTESIAN_POINT ( 'NONE',  ( -1.059188295049996231, -6.027090492554000534, 64.35000000000000853 ) ) ;
#13499=AXIS2_PLACEMENT_3D ( 'NONE', #1887, #686, #11311 ) ;
#13501=DIRECTION ( 'NONE',  ( 0.7071067811865474617, 0.000000000000000000, 0.7071067811865474617 ) ) ;
#13505=DIRECTION ( 'NONE',  ( 1.000000000000000000, 0.000000000000000000, 0.000000000000000000 ) ) ;
#13506=DIRECTION ( 'NONE',  ( 0.000000000000000000, 0.000000000000000000, -1.000000000000000000 ) ) ;
#13507=CARTESIAN_POINT ( 'NONE',  ( -18.05918829504999934, 10.97290950744599947, 61.86500000000000199 ) ) ;
#13511=ADVANCED_FACE ( 'NONE', ( #4270 ), #11117, .T. ) ;
#13512=EDGE_CURVE ( 'NONE', #1130, #9971, #5744, .T. ) ;
#13515=ORIENTED_EDGE ( 'NONE', *, *, #2424, .T. ) ;
#13517=CARTESIAN_POINT ( 'NONE',  ( -18.05918829504999934, 10.97290950744599947, 64.54999999999999716 ) ) ;
#13518=CARTESIAN_POINT ( 'NONE',  ( -1.059188295049996231, 27.97290950744599769, 64.85000000000000853 ) ) ;
#13519=DIRECTION ( 'NONE',  ( 0.000000000000000000, 0.000000000000000000, -1.000000000000000000 ) ) ;
#13521=CARTESIAN_POINT ( 'NONE',  ( -18.05918829504999934, 10.97290950744599947, 57.35000000000000142 ) ) ;
#13522=LINE ( 'NONE', #8559, #3774 ) ;
#13523=DIRECTION ( 'NONE',  ( -0.6615960714621568206, 0.7498604124941127269, 0.000000000000000000 ) ) ;
#13524=VECTOR ( 'NONE', #4785, 1000.000000000000000 ) ;
#13525=DIRECTION ( 'NONE',  ( -0.3202092937642119774, -0.6304490528084099044, -0.7071067811865499042 ) ) ;
#13528=EDGE_CURVE ( 'NONE', #8989, #13262, #12891, .T. ) ;
#13532=EDGE_CURVE ( 'NONE', #7236, #9493, #4426, .T. ) ;
#13535=ORIENTED_EDGE ( 'NONE', *, *, #8545, .F. ) ;
#13539=DIRECTION ( 'NONE',  ( 0.000000000000000000, 0.000000000000000000, 1.000000000000000000 ) ) ;
#13541=CARTESIAN_POINT ( 'NONE',  ( -18.05918829504999934, 10.97290950744599947, 63.64999999999999858 ) ) ;
#13542=DIRECTION ( 'NONE',  ( 0.000000000000000000, 0.000000000000000000, -1.000000000000000000 ) ) ;
#13546=VERTEX_POINT ( 'NONE', #3228 ) ;
#13547=CARTESIAN_POINT ( 'NONE',  ( -14.80437462465609144, 30.13112197626990607, 55.06331687826421017 ) ) ;
#13548=AXIS2_PLACEMENT_3D ( 'NONE', #1707, #11355, #8276 ) ;
#13549=AXIS2_PLACEMENT_3D ( 'NONE', #10260, #670, #4942 ) ;
#13552=EDGE_CURVE ( 'NONE', #1905, #7929, #9707, .T. ) ;
#13554=DIRECTION ( 'NONE',  ( -1.000000000000000000, 0.000000000000000000, 0.000000000000000000 ) ) ;
#13558=ORIENTED_EDGE ( 'NONE', *, *, #9153, .F. ) ;
#13560=LINE ( 'NONE', #7659, #10565 ) ;
#13561=CARTESIAN_POINT ( 'NONE',  ( -19.36881307809606056, 27.92256143814164560, 58.10788369877568016 ) ) ;
#13565=EDGE_CURVE ( 'NONE', #1636, #10781, #6635, .T. ) ;
#13566=AXIS2_PLACEMENT_3D ( 'NONE', #11063, #10927, #12109 ) ;
#13567=ORIENTED_EDGE ( 'NONE', *, *, #13552, .F. ) ;
#13574=ORIENTED_EDGE ( 'NONE', *, *, #11186, .T. ) ;
#13576=DIRECTION ( 'NONE',  ( 0.000000000000000000, 0.000000000000000000, 1.000000000000000000 ) ) ;
#13577=FACE_BOUND ( 'NONE', #7677, .T. ) ;
#13579=DIRECTION ( 'NONE',  ( 0.000000000000000000, 0.000000000000000000, -1.000000000000000000 ) ) ;
#13581=VERTEX_POINT ( 'NONE', #9923 ) ;
#13583=CARTESIAN_POINT ( 'NONE',  ( 1.640811704950000172, 27.97290950744599769, 64.85000000000000853 ) ) ;
#13585=ORIENTED_EDGE ( 'NONE', *, *, #4099, .F. ) ;
#13586=CARTESIAN_POINT ( 'NONE',  ( -18.05918829504999934, 10.97290950744599947, 57.35000000000000142 ) ) ;
#13587=DIRECTION ( 'NONE',  ( -1.000000000000000000, 0.000000000000000000, 0.000000000000000000 ) ) ;
#13589=CARTESIAN_POINT ( 'NONE',  ( -18.05918829504999934, 10.97290950744599947, 64.35000000000000853 ) ) ;
#13590=CARTESIAN_POINT ( 'NONE',  ( -18.05918829504999934, 10.97290950744599947, 64.35000000000000853 ) ) ;
#13592=EDGE_CURVE ( 'NONE', #759, #10847, #10666, .T. ) ;
#13593=LINE ( 'NONE', #2095, #12962 ) ;
#13596=AXIS2_PLACEMENT_3D ( 'NONE', #2233, #6471, #2030 ) ;
#13598=EDGE_LOOP ( 'NONE', ( #9372, #306 ) ) ;
#13599=AXIS2_PLACEMENT_3D ( 'NONE', #3630, #6756, #334 ) ;
#13600=DIRECTION ( 'NONE',  ( 0.6615960714621569316, -0.7498604124941123938, 0.000000000000000000 ) ) ;
#13601=ORIENTED_EDGE ( 'NONE', *, *, #9657, .T. ) ;
#13603=EDGE_CURVE ( 'NONE', #8732, #10843, #3108, .T. ) ;
#13605=EDGE_LOOP ( 'NONE', ( #7034, #10675, #8503, #13764 ) ) ;
#13607=CARTESIAN_POINT ( 'NONE',  ( -5.631644894983189431, 10.97290950744599947, 64.85000000000000853 ) ) ;
#13610=ORIENTED_EDGE ( 'NONE', *, *, #1514, .F. ) ;
#13616=VECTOR ( 'NONE', #11234, 1000.000000000000000 ) ;
#13618=CARTESIAN_POINT ( 'NONE',  ( -14.52722204234322945, 30.09020406744985365, 59.02705628552431705 ) ) ;
#13621=ORIENTED_EDGE ( 'NONE', *, *, #5025, .T. ) ;
#13622=CARTESIAN_POINT ( 'NONE',  ( -35.05918829505000645, 27.97290950744599769, 17.25000000000000000 ) ) ;
#13627=DIRECTION ( 'NONE',  ( 0.000000000000000000, 0.000000000000000000, -1.000000000000000000 ) ) ;
#13628=DIRECTION ( 'NONE',  ( -0.000000000000000000, -0.000000000000000000, 1.000000000000000000 ) ) ;
#13630=ORIENTED_EDGE ( 'NONE', *, *, #10795, .F. ) ;
#13631=CARTESIAN_POINT ( 'NONE',  ( -35.05918829505000645, 27.97290950744599769, 7.250000000000000000 ) ) ;
#13632=DIRECTION ( 'NONE',  ( -0.9496839325805410681, 0.3132098788326420080, 0.000000000000000000 ) ) ;
#13633=CARTESIAN_POINT ( 'NONE',  ( -18.05918829504999934, 10.97290950744599947, 58.54999999999999716 ) ) ;
#13634=CYLINDRICAL_SURFACE ( 'NONE', #4013, 4.250000000000000000 ) ;
#13636=CIRCLE ( 'NONE', #2056, 2.500000000000000000 ) ;
#13638=EDGE_CURVE ( 'NONE', #7318, #3046, #5705, .T. ) ;
#13642=ORIENTED_EDGE ( 'NONE', *, *, #10146, .T. ) ;
#13644=ORIENTED_EDGE ( 'NONE', *, *, #5261, .T. ) ;
#13645=EDGE_LOOP ( 'NONE', ( #2558, #12740, #4625, #5084 ) ) ;
#13646=ORIENTED_EDGE ( 'NONE', *, *, #584, .F. ) ;
#13647=CARTESIAN_POINT ( 'NONE',  ( -14.82135136386927954, 17.34777515364455169, 64.85000000000000853 ) ) ;
#13648=EDGE_CURVE ( 'NONE', #3038, #6850, #9108, .T. ) ;
#13660=DIRECTION ( 'NONE',  ( -0.1325514707600310149, -1.623287343885459848E-17, -0.9911761234005551646 ) ) ;
#13661=ORIENTED_EDGE ( 'NONE', *, *, #9195, .F. ) ;
#13662=ORIENTED_EDGE ( 'NONE', *, *, #1598, .F. ) ;
#13664=LINE ( 'NONE', #6109, #3297 ) ;
#13665=CARTESIAN_POINT ( 'NONE',  ( -3.759188295049999518, -6.027090492554000534, 64.85000000000000853 ) ) ;
#13670=FACE_BOUND ( 'NONE', #5850, .T. ) ;
#13671=VECTOR ( 'NONE', #4581, 1000.000000000000114 ) ;
#13673=EDGE_CURVE ( 'NONE', #3038, #8537, #410, .T. ) ;
#13674=EDGE_CURVE ( 'NONE', #2401, #2781, #13193, .T. ) ;
#13677=CARTESIAN_POINT ( 'NONE',  ( -18.05918829504999934, 10.97290950744599947, 24.10000000000000142 ) ) ;
#13678=CARTESIAN_POINT ( 'NONE',  ( -20.17037093922029456, 15.77813698237436668, 68.60160116090442273 ) ) ;
#13679=DIRECTION ( 'NONE',  ( 0.000000000000000000, 0.000000000000000000, -1.000000000000000000 ) ) ;
#13682=AXIS2_PLACEMENT_3D ( 'NONE', #12626, #12418, #3078 ) ;
#13683=ADVANCED_FACE ( 'NONE', ( #1521 ), #5778, .F. ) ;
#13684=VERTEX_POINT ( 'NONE', #1663 ) ;
#13686=CARTESIAN_POINT ( 'NONE',  ( -15.75919308146518283, 30.24616810854943694, 60.82807559156996291 ) ) ;
#13687=VERTEX_POINT ( 'NONE', #8937 ) ;
#13690=DIRECTION ( 'NONE',  ( -1.000000000000000000, 0.000000000000000000, 0.000000000000000000 ) ) ;
#13693=ORIENTED_EDGE ( 'NONE', *, *, #10582, .T. ) ;
#13694=DIRECTION ( 'NONE',  ( -1.000000000000000000, 0.000000000000000000, 0.000000000000000000 ) ) ;
#13696=CARTESIAN_POINT ( 'NONE',  ( -28.87730642030694739, 29.81324547859995278, 5.250000000000000000 ) ) ;
#13697=CARTESIAN_POINT ( 'NONE',  ( -16.55918829504999579, 27.90660372932210009, 57.35000000000000142 ) ) ;
#13699=ORIENTED_EDGE ( 'NONE', *, *, #13715, .F. ) ;
#13702=ORIENTED_EDGE ( 'NONE', *, *, #6171, .T. ) ;
#13704=ORIENTED_EDGE ( 'NONE', *, *, #8316, .F. ) ;
#13706=DIRECTION ( 'NONE',  ( -0.6615960714621568206, 0.7498604124941127269, 0.000000000000000000 ) ) ;
#13708=ORIENTED_EDGE ( 'NONE', *, *, #9080, .F. ) ;
#13710=CARTESIAN_POINT ( 'NONE',  ( -18.92810326151374056, 26.94929807862704507, 56.12730036355915075 ) ) ;
#13711=CARTESIAN_POINT ( 'NONE',  ( -18.05918829504999934, 7.130333642789880244, 64.85000000000000853 ) ) ;
#13714=LINE ( 'NONE', #12809, #1334 ) ;
#13715=EDGE_CURVE ( 'NONE', #4079, #1108, #3571, .T. ) ;
#13719=LINE ( 'NONE', #4169, #3339 ) ;
#13720=ORIENTED_EDGE ( 'NONE', *, *, #13306, .F. ) ;
#13721=CARTESIAN_POINT ( 'NONE',  ( -35.05918829505000645, -6.027090492554000534, 58.85000000000000142 ) ) ;
#13724=CARTESIAN_POINT ( 'NONE',  ( -34.21361676484809777, 5.678153534393399759, 62.14999999999999858 ) ) ;
#13726=CYLINDRICAL_SURFACE ( 'NONE', #10917, 17.00000000000000000 ) ;
#13727=CARTESIAN_POINT ( 'NONE',  ( -35.05918829505000645, -6.027090492554000534, 58.85000000000000142 ) ) ;
#13730=PLANE ( 'NONE',  #7999 ) ;
#13731=VECTOR ( 'NONE', #13660, 1000.000000000000114 ) ;
#13732=ADVANCED_FACE ( 'NONE', ( #11442, #1812, #3968, #8300, #967, #6185 ), #13730, .F. ) ;
#13733=ORIENTED_EDGE ( 'NONE', *, *, #2194, .T. ) ;
#13734=LINE ( 'NONE', #11660, #7443 ) ;
#13735=ORIENTED_EDGE ( 'NONE', *, *, #4324, .T. ) ;
#13736=ORIENTED_EDGE ( 'NONE', *, *, #8592, .F. ) ;
#13737=ORIENTED_EDGE ( 'NONE', *, *, #10201, .F. ) ;
#13739=VECTOR ( 'NONE', #4236, 1000.000000000000114 ) ;
#13741=DIRECTION ( 'NONE',  ( 1.000000000000000000, 0.000000000000000000, 0.000000000000000000 ) ) ;
#13742=DIRECTION ( 'NONE',  ( 0.000000000000000000, 0.000000000000000000, 1.000000000000000000 ) ) ;
#13743=CARTESIAN_POINT ( 'NONE',  ( -15.84935410452223792, 6.254721532704953901, 68.64057313984737618 ) ) ;
#13744=FACE_OUTER_BOUND ( 'NONE', #5189, .T. ) ;
#13746=CARTESIAN_POINT ( 'NONE',  ( -14.54431709152540897, 30.09282919894160813, 59.07233549947221718 ) ) ;
#13756=CIRCLE ( 'NONE', #12658, 2.700000000000000178 ) ;
#13757=CARTESIAN_POINT ( 'NONE',  ( -1.433900126049995061, 2.660265422446006500, 63.26601075299999621 ) ) ;
#13758=EDGE_CURVE ( 'NONE', #11456, #12316, #8092, .T. ) ;
#13759=CARTESIAN_POINT ( 'NONE',  ( -24.65502162805000097, 10.97290950744599947, 60.40999999999999659 ) ) ;
#13760=AXIS2_PLACEMENT_3D ( 'NONE', #8406, #12675, #3126 ) ;
#13761=AXIS2_PLACEMENT_3D ( 'NONE', #9482, #5072, #676 ) ;
#13762=ORIENTED_EDGE ( 'NONE', *, *, #7416, .F. ) ;
#13764=ORIENTED_EDGE ( 'NONE', *, *, #1540, .F. ) ;
#13766=EDGE_LOOP ( 'NONE', ( #12973, #5260, #7332, #10235 ) ) ;
#13767=CARTESIAN_POINT ( 'NONE',  ( -35.05918829505000645, -6.027090492554000534, 64.85000000000000853 ) ) ;
#13771=VECTOR ( 'NONE', #10552, 1000.000000000000000 ) ;
#13774=CIRCLE ( 'NONE', #7512, 4.250000000000003553 ) ;
#13776=EDGE_CURVE ( 'NONE', #7296, #223, #7523, .T. ) ;
#13777=VECTOR ( 'NONE', #11002, 1000.000000000000227 ) ;
#13780=CIRCLE ( 'NONE', #5978, 16.95000000000000284 ) ;
#13782=ORIENTED_EDGE ( 'NONE', *, *, #3991, .T. ) ;
#13783=CIRCLE ( 'NONE', #423, 16.50000000000000000 ) ;
#13788=DIRECTION ( 'NONE',  ( -0.3132098788326400651, 0.9496839325805417342, 0.000000000000000000 ) ) ;
#13791=FACE_OUTER_BOUND ( 'NONE', #8595, .T. ) ;
#13793=CARTESIAN_POINT ( 'NONE',  ( -35.05918829505000645, -6.027090492554000534, 64.85000000000000853 ) ) ;
#13796=CARTESIAN_POINT ( 'NONE',  ( -13.90184482195073912, 7.972993985840365561, 68.75388058398559110 ) ) ;
#13797=VECTOR ( 'NONE', #7742, 1000.000000000000000 ) ;
#13798=VECTOR ( 'NONE', #386, 1000.000000000000000 ) ;
#13799=MANIFOLD_SOLID_BREP ( 'Fillet1', #7014 ) ;
#13800=VECTOR ( 'NONE', #2644, 1000.000000000000000 ) ;
#13802=ORIENTED_EDGE ( 'NONE', *, *, #12852, .T. ) ;
#13804=VERTEX_POINT ( 'NONE', #10539 ) ;
ENDSEC;
END-ISO-10303-21;
